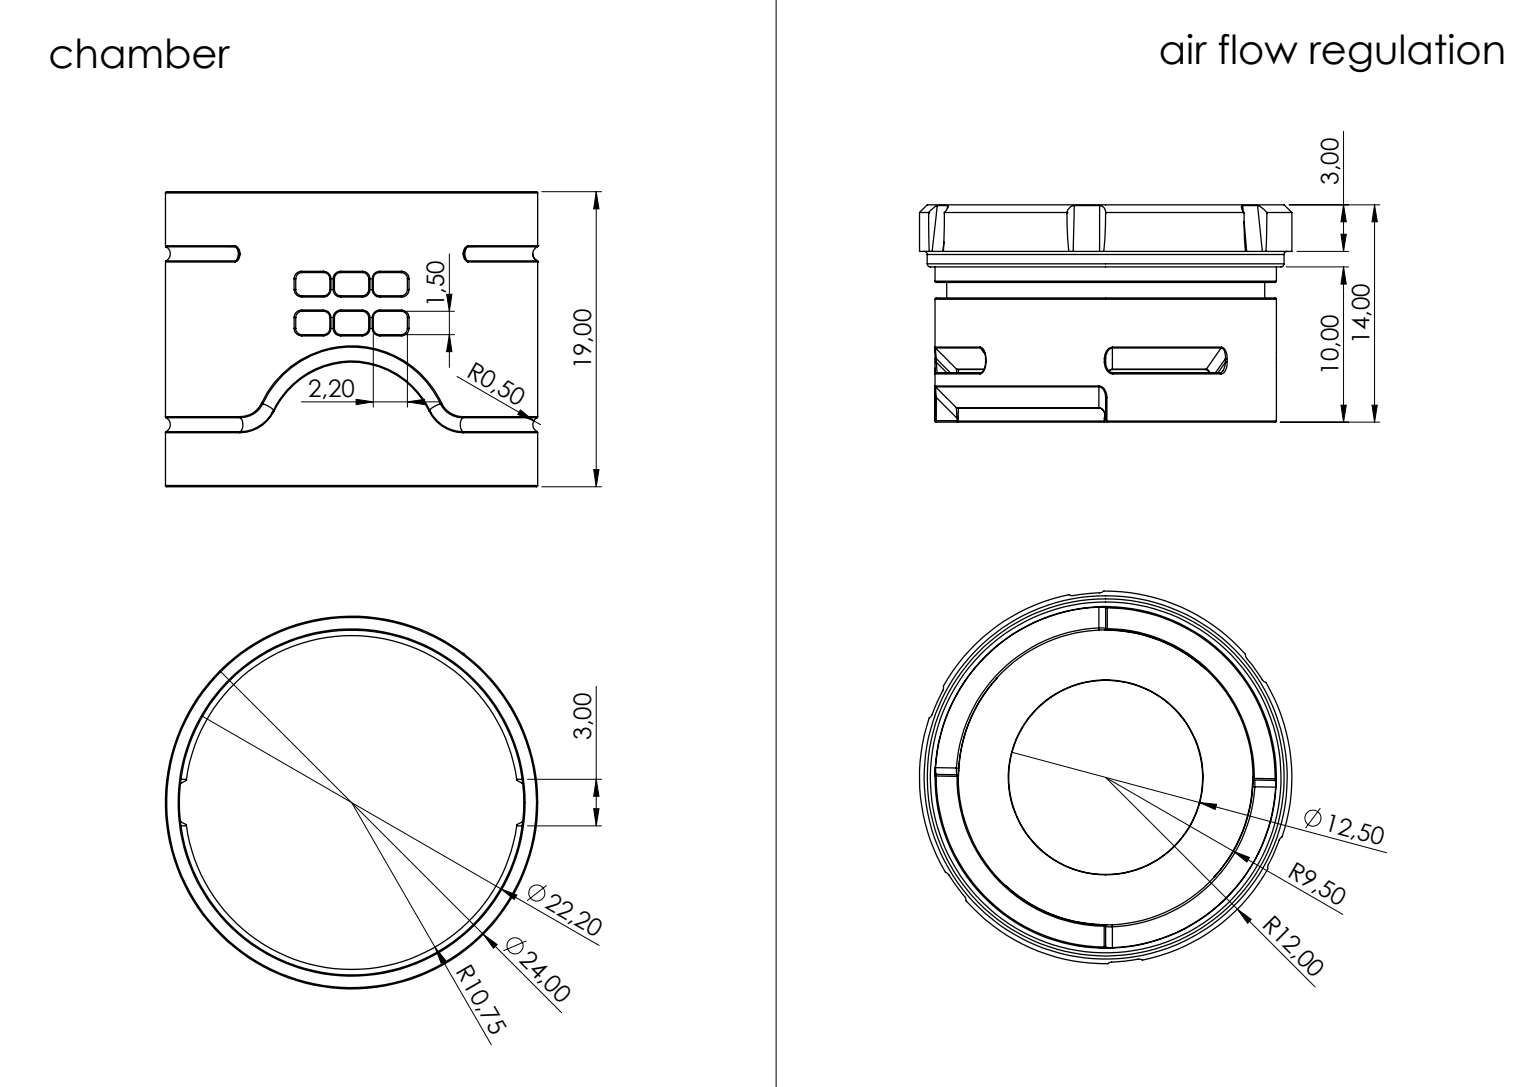
ISO-10303-21;
HEADER;
FILE_DESCRIPTION (('STEP AP214'),
    '1' );
FILE_NAME ('chamber.step',
    '2026-10-05T20:10:51',
    ( '' ),
    ( '' ),
    'SwSTEP 2.0',
    'SolidWorks 2020',
    '' );
FILE_SCHEMA (( 'AUTOMOTIVE_DESIGN' ));
ENDSEC;

DATA;
#17=CARTESIAN_POINT ( 'NONE',  ( 11.89942855770814312, 9.799999999999998934, 0.6999999999999992895 ) ) ;
#42=PRESENTATION_STYLE_ASSIGNMENT (( #185202 ) ) ;
#61=FACE_OUTER_BOUND ( 'NONE', #36024, .T. ) ;
#92=CARTESIAN_POINT ( 'NONE',  ( 6.928203230275524760, 15.51845925587262798, -9.797958971132702644 ) ) ;
#96=CARTESIAN_POINT ( 'NONE',  ( 11.88237951145550220, 12.34319347378715115, 0.9087114598430685586 ) ) ;
#105=CARTESIAN_POINT ( 'NONE',  ( -9.333041836226904309, 15.44694763438996077, -7.472413793095822321 ) ) ;
#118=ORIENTED_EDGE ( 'NONE', *, *, #154536, .F. ) ;
#120=CARTESIAN_POINT ( 'NONE',  ( 10.50000000000000355, 11.00832445802304882, -3.600000000000000533 ) ) ;
#124=VERTEX_POINT ( 'NONE', #206751 ) ;
#158=CARTESIAN_POINT ( 'NONE',  ( -10.12724623727299900, 3.700526055228949840, -6.355430437403613020 ) ) ;
#163=CARTESIAN_POINT ( 'NONE',  ( 11.84668730067608244, 12.69999999999998153, 1.399999999999998357 ) ) ;
#164=CARTESIAN_POINT ( 'NONE',  ( -11.92051736251532112, 12.44819756207321149, -1.381800029228967386 ) ) ;
#189=DIRECTION ( 'NONE',  ( 0.000000000000000000, 1.000000000000000000, 0.000000000000000000 ) ) ;
#190=FACE_OUTER_BOUND ( 'NONE', #152846, .T. ) ;
#192=ORIENTED_EDGE ( 'NONE', *, *, #191821, .F. ) ;
#199=ORIENTED_EDGE ( 'NONE', *, *, #95230, .T. ) ;
#216=CARTESIAN_POINT ( 'NONE',  ( 11.84668730067608244, 12.69999999999999929, -1.320000000000001616 ) ) ;
#223=EDGE_LOOP ( 'NONE', ( #165565, #34083, #144999, #128787 ) ) ;
#227=ORIENTED_EDGE ( 'NONE', *, *, #162616, .F. ) ;
#234=ORIENTED_EDGE ( 'NONE', *, *, #52222, .T. ) ;
#242=( NAMED_UNIT ( * ) PLANE_ANGLE_UNIT ( ) SI_UNIT ( $, .RADIAN. ) );
#252=CARTESIAN_POINT ( 'NONE',  ( 9.376191831160928913, 12.67849274587929820, -8.895508691099047738 ) ) ;
#267=LINE ( 'NONE', #66337, #6225 ) ;
#276=AXIS2_PLACEMENT_3D ( 'NONE', #147982, #164223, #79761 ) ;
#348=CARTESIAN_POINT ( 'NONE',  ( 8.061225138011870683, 15.94050400400142564, -9.794890688158101710 ) ) ;
#407=CARTESIAN_POINT ( 'NONE',  ( 9.501800845313253419, 13.11895608245291101, -7.330069317485494729 ) ) ;
#414=CIRCLE ( 'NONE', #87036, 11.09999999999999964 ) ;
#421=CARTESIAN_POINT ( 'NONE',  ( 11.91826849282518275, 12.69999999999999929, -1.400000000000001465 ) ) ;
#425=EDGE_CURVE ( 'NONE', #105059, #66250, #59241, .T. ) ;
#460=CARTESIAN_POINT ( 'NONE',  ( -11.37874721094434527, 6.569860378138817403, -3.816774967323496082 ) ) ;
#468=DIRECTION ( 'NONE',  ( -0.1510067114093955887, -0.000000000000000000, -0.9885327375000383388 ) ) ;
#486=DIRECTION ( 'NONE',  ( 1.000000000000000000, -0.000000000000000000, -0.000000000000000000 ) ) ;
#487=SURFACE_STYLE_USAGE ( .BOTH. , #166223 ) ;
#499=ORIENTED_EDGE ( 'NONE', *, *, #8528, .T. ) ;
#510=EDGE_CURVE ( 'NONE', #23152, #210434, #174637, .T. ) ;
#516=CARTESIAN_POINT ( 'NONE',  ( -10.62873463776380234, 12.29999999999998295, 3.199999999999997957 ) ) ;
#542=ORIENTED_EDGE ( 'NONE', *, *, #88694, .T. ) ;
#554=VECTOR ( 'NONE', #28356, 1000.000000000000000 ) ;
#599=CYLINDRICAL_SURFACE ( 'NONE', #53747, 0.3999999999999997446 ) ;
#634=CARTESIAN_POINT ( 'NONE',  ( -10.78402850230606447, 8.013881820625746499, 4.046242669647421408 ) ) ;
#648=EDGE_CURVE ( 'NONE', #121570, #167726, #212215, .T. ) ;
#662=UNCERTAINTY_MEASURE_WITH_UNIT (LENGTH_MEASURE( 1.000000000000000082E-05 ), #182215, 'distance_accuracy_value', 'NONE');
#671=DIRECTION ( 'NONE',  ( 1.000000000000000000, -0.000000000000000000, -0.000000000000000000 ) ) ;
#700=ADVANCED_FACE ( 'NONE', ( #185046 ), #198533, .T. ) ;
#702=VERTEX_POINT ( 'NONE', #118001 ) ;
#718=VECTOR ( 'NONE', #62707, 1000.000000000000000 ) ;
#733=CARTESIAN_POINT ( 'NONE',  ( -9.399770542442999144, 4.999985930147239799, -6.933469103752857521 ) ) ;
#743=CARTESIAN_POINT ( 'NONE',  ( -11.96215121607992593, 13.82833553780824154, -0.9565349792967606790 ) ) ;
#749=CARTESIAN_POINT ( 'NONE',  ( 11.53069314862830552, 7.261250335387300581, -3.355468136185856487 ) ) ;
#760=CARTESIAN_POINT ( 'NONE',  ( 10.67997715883384657, 8.352520031436601045, -3.105267373736821046 ) ) ;
#766=CIRCLE ( 'NONE', #108191, 0.07999999999999998779 ) ;
#773=EDGE_LOOP ( 'NONE', ( #1049, #99023, #98681, #151558, #138881, #82301, #133035, #37995, #73322, #97682, #96732, #136112, #8265, #74514, #72858, #38949, #164337, #200453 ) ) ;
#777=CARTESIAN_POINT ( 'NONE',  ( 0.08053691275167890185, 14.48153890507870223, 11.99972973886013961 ) ) ;
#831=EDGE_CURVE ( 'NONE', #191521, #28791, #95318, .T. ) ;
#836=( GEOMETRIC_REPRESENTATION_CONTEXT ( 3 ) GLOBAL_UNCERTAINTY_ASSIGNED_CONTEXT ( ( #213503 ) ) GLOBAL_UNIT_ASSIGNED_CONTEXT ( ( #89871, #123512, #158065 ) ) REPRESENTATION_CONTEXT ( 'NONE', 'WORKASPACE' ) );
#840=ORIENTED_EDGE ( 'NONE', *, *, #141283, .F. ) ;
#885=CARTESIAN_POINT ( 'NONE',  ( 11.84668730067608600, 13.40000000000000036, -1.400000000000001910 ) ) ;
#890=FACE_OUTER_BOUND ( 'NONE', #59511, .T. ) ;
#922=FACE_OUTER_BOUND ( 'NONE', #13196, .T. ) ;
#933=DIRECTION ( 'NONE',  ( 0.000000000000000000, 1.000000000000000000, 0.000000000000000000 ) ) ;
#936=VECTOR ( 'NONE', #86539, 1000.000000000000000 ) ;
#945=CARTESIAN_POINT ( 'NONE',  ( -1.499999999999964029, 8.500000000000000000, 9.886859966642596476 ) ) ;
#971=CARTESIAN_POINT ( 'NONE',  ( 11.33772463945037146, 12.69999999999998153, 3.599999999999999201 ) ) ;
#990=B_SPLINE_CURVE_WITH_KNOTS ( 'NONE', 3,
 ( #112463, #131886, #64702, #162226, #79885, #212006 ),
 .UNSPECIFIED., .F., .F.,
 ( 4, 2, 4 ),
 ( 0.001889712630306643673, 0.002203932548491402497, 0.002518152466676161320 ),
 .UNSPECIFIED. ) ;
#1001=AXIS2_PLACEMENT_3D ( 'NONE', #80650, #164042, #112153 ) ;
#1016=AXIS2_PLACEMENT_3D ( 'NONE', #89451, #186921, #6019 ) ;
#1034=CARTESIAN_POINT ( 'NONE',  ( -10.32660017610915837, 5.019824769181640889, 7.354833152352289183 ) ) ;
#1037=ADVANCED_FACE ( 'NONE', ( #178914 ), #183155, .F. ) ;
#1046=CARTESIAN_POINT ( 'NONE',  ( -11.45842088241054491, 11.09306470877032069, 3.566211699757684261 ) ) ;
#1049=ORIENTED_EDGE ( 'NONE', *, *, #67497, .T. ) ;
#1053=CARTESIAN_POINT ( 'NONE',  ( -15.75000000000000000, 10.19999999999998153, 3.599999999999999201 ) ) ;
#1054=FACE_OUTER_BOUND ( 'NONE', #104348, .T. ) ;
#1062=CARTESIAN_POINT ( 'NONE',  ( -11.37613258624509349, 7.826217927974032484, 3.683897043248439029 ) ) ;
#1063=CARTESIAN_POINT ( 'NONE',  ( 11.78331023100045627, 12.29999999999998295, 1.799999999999999600 ) ) ;
#1081=CARTESIAN_POINT ( 'NONE',  ( 11.89942855770813956, 12.22000000000000064, 0.6999999999999992895 ) ) ;
#1092=VECTOR ( 'NONE', #206274, 1000.000000000000000 ) ;
#1097=CIRCLE ( 'NONE', #56491, 11.92000000000000171 ) ;
#1116=CARTESIAN_POINT ( 'NONE',  ( 0.000000000000000000, 12.22000000000000064, 0.000000000000000000 ) ) ;
#1117=VERTEX_POINT ( 'NONE', #82446 ) ;
#1124=CARTESIAN_POINT ( 'NONE',  ( 11.55950211276791251, 11.37999999999998302, 3.221476510067114329 ) ) ;
#1132=CARTESIAN_POINT ( 'NONE',  ( 11.86239285000045918, 11.37999999999999901, -1.812080536912753059 ) ) ;
#1145=CARTESIAN_POINT ( 'NONE',  ( 6.902720183911290164, 14.55305236562705318, -9.761920501353818835 ) ) ;
#1159=ORIENTED_EDGE ( 'NONE', *, *, #134668, .F. ) ;
#1233=CARTESIAN_POINT ( 'NONE',  ( -10.89183333199790482, 4.909323612238607915, -5.036858318171161919 ) ) ;
#1240=LINE ( 'NONE', #117214, #18483 ) ;
#1265=CARTESIAN_POINT ( 'NONE',  ( -1.785627835867960034, 15.44799008577503585, -11.82984269095817353 ) ) ;
#1266=CARTESIAN_POINT ( 'NONE',  ( 11.78331023100045627, 11.29999999999999893, -1.800000000000001155 ) ) ;
#1268=CIRCLE ( 'NONE', #122445, 12.00000000000000178 ) ;
#1295=CARTESIAN_POINT ( 'NONE',  ( 11.86145016429273191, 10.90000000000000036, 1.099999999999996758 ) ) ;
#1299=VERTEX_POINT ( 'NONE', #59288 ) ;
#1315=CARTESIAN_POINT ( 'NONE',  ( -11.43653507270588499, 5.655220009861049668, 5.468867579827167980 ) ) ;
#1378=CARTESIAN_POINT ( 'NONE',  ( -10.43233925736708301, 5.066585305077033752, -5.254699789447807134 ) ) ;
#1379=CARTESIAN_POINT ( 'NONE',  ( -9.348561386651960348, 4.000000000000000888, 7.001914024036570261 ) ) ;
#1405=FACE_OUTER_BOUND ( 'NONE', #99903, .T. ) ;
#1425=CARTESIAN_POINT ( 'NONE',  ( 7.320801413324473650, 14.00000000000000000, -10.35317664616355771 ) ) ;
#1442=CARTESIAN_POINT ( 'NONE',  ( 10.62873463776380056, 12.30000000000000071, -3.200000000000001510 ) ) ;
#1480=CARTESIAN_POINT ( 'NONE',  ( 1.448815997565377156, 7.903552007303750848, -10.65195286442484601 ) ) ;
#1482=EDGE_CURVE ( 'NONE', #30243, #96092, #98102, .T. ) ;
#1521=CARTESIAN_POINT ( 'NONE',  ( -9.333041836230696831, 14.55305236563169302, -7.472413793098840351 ) ) ;
#1554=ORIENTED_EDGE ( 'NONE', *, *, #33991, .T. ) ;
#1620=CIRCLE ( 'NONE', #57014, 0.07999999999999998779 ) ;
#1668=AXIS2_PLACEMENT_3D ( 'NONE', #81303, #62908, #211285 ) ;
#1710=CARTESIAN_POINT ( 'NONE',  ( 0.3263184169966619752, 15.00000000000058265, -11.67999999558625213 ) ) ;
#1712=CARTESIAN_POINT ( 'NONE',  ( -10.44369633504468631, 5.112959841837462882, -5.232137017608344820 ) ) ;
#1743=DIRECTION ( 'NONE',  ( 0.000000000000000000, 0.000000000000000000, 1.000000000000000000 ) ) ;
#1752=DIRECTION ( 'NONE',  ( 0.000000000000000000, 0.000000000000000000, 1.000000000000000000 ) ) ;
#1769=CIRCLE ( 'NONE', #174839, 0.5000000000000016653 ) ;
#1774=( NAMED_UNIT ( * ) PLANE_ANGLE_UNIT ( ) SI_UNIT ( $, .RADIAN. ) );
#1783=CARTESIAN_POINT ( 'NONE',  ( 11.95359438121989726, 9.995781002913002311, -1.059536798430469107 ) ) ;
#1810=CARTESIAN_POINT ( 'NONE',  ( -11.75342398721120141, 4.618418902329548992, -5.022351803590792585 ) ) ;
#1821=( NAMED_UNIT ( * ) PLANE_ANGLE_UNIT ( ) SI_UNIT ( $, .RADIAN. ) );
#1825=ORIENTED_EDGE ( 'NONE', *, *, #25480, .F. ) ;
#1828=CARTESIAN_POINT ( 'NONE',  ( 11.09870862492791233, 7.996335997987229049, -4.583701278145491109 ) ) ;
#1840=CARTESIAN_POINT ( 'NONE',  ( 10.48872307347595090, 11.88768493876267485, 6.438521854865753014 ) ) ;
#1849=CARTESIAN_POINT ( 'NONE',  ( -11.88235317400313917, 12.34335760226970358, 0.9089793033029930358 ) ) ;
#1856=STYLED_ITEM ( 'NONE', ( #32642 ), #1037 ) ;
#1895=CARTESIAN_POINT ( 'NONE',  ( 0.000000000000000000, 3.553052365627050513, 0.000000000000000000 ) ) ;
#1976=CIRCLE ( 'NONE', #22858, 0.07999999999999946043 ) ;
#1999=DIRECTION ( 'NONE',  ( 0.000000000000000000, 1.000000000000000000, 0.000000000000000000 ) ) ;
#2010=CARTESIAN_POINT ( 'NONE',  ( 0.000000000000000000, 18.91999999999999815, 0.000000000000000000 ) ) ;
#2037=CARTESIAN_POINT ( 'NONE',  ( 8.748033642589533088, 13.52645069410513479, 8.214566069811549909 ) ) ;
#2094=FILL_AREA_STYLE_COLOUR ( '', #209766 ) ;
#2096=CARTESIAN_POINT ( 'NONE',  ( -9.928151704202875294, 5.423124072284297270, 6.082134274749043001 ) ) ;
#2098=LINE ( 'NONE', #81258, #144593 ) ;
#2101=AXIS2_PLACEMENT_3D ( 'NONE', #159302, #14090, #63931 ) ;
#2120=CARTESIAN_POINT ( 'NONE',  ( -10.63115277548007498, 5.888090174969209833, -5.475543521278559922 ) ) ;
#2123=FACE_OUTER_BOUND ( 'NONE', #176365, .T. ) ;
#2148=EDGE_CURVE ( 'NONE', #31723, #61426, #1268, .T. ) ;
#2180=DIRECTION ( 'NONE',  ( 0.000000000000000000, -1.000000000000000000, -9.023263958591317418E-17 ) ) ;
#2199=ORIENTED_EDGE ( 'NONE', *, *, #9864, .T. ) ;
#2205=DIRECTION ( 'NONE',  ( 1.000000000000000000, -0.000000000000000000, -0.000000000000000000 ) ) ;
#2216=VECTOR ( 'NONE', #157528, 1000.000000000000000 ) ;
#2241=CARTESIAN_POINT ( 'NONE',  ( -10.51596412982177853, 9.986590817315772028, -3.553961965504329967 ) ) ;
#2257=CIRCLE ( 'NONE', #26555, 12.00000000000000178 ) ;
#2259=ORIENTED_EDGE ( 'NONE', *, *, #27400, .F. ) ;
#2292=CARTESIAN_POINT ( 'NONE',  ( -10.84253909858433218, 4.919570308430901484, -5.035411995924089723 ) ) ;
#2295=DIRECTION ( 'NONE',  ( -0.000000000000000000, -1.000000000000000000, -0.000000000000000000 ) ) ;
#2314=EDGE_CURVE ( 'NONE', #158402, #95365, #73964, .T. ) ;
#2318=VERTEX_POINT ( 'NONE', #66709 ) ;
#2327=LINE ( 'NONE', #34843, #100006 ) ;
#2336=ORIENTED_EDGE ( 'NONE', *, *, #208712, .T. ) ;
#2343=( BOUNDED_SURFACE ( )  B_SPLINE_SURFACE ( 3, 2, ( 
 ( #205237, #55808, #154383 ),
 ( #105661, #204153, #141381 ),
 ( #56878, #5960, #187929 ),
 ( #41724, #157600, #207391 ),
 ( #73106, #125168, #189007 ),
 ( #158656, #171688, #191127 ) ),
 .UNSPECIFIED., .F., .F., .T. ) 
 B_SPLINE_SURFACE_WITH_KNOTS ( ( 4, 2, 4 ),
 ( 3, 3 ),
 ( 0.000000000000000000, 0.0003754689591423960443, 0.0007509379182847920886 ),
 ( 0.000000000000000000, 1.000000000000000000 ),
 .UNSPECIFIED. ) 
 GEOMETRIC_REPRESENTATION_ITEM ( )  RATIONAL_B_SPLINE_SURFACE ( (
 ( 1.000000000000000000, 0.7071067811865551223, 1.000000000000000000),
 ( 1.000000000000000000, 0.7018599272024059754, 1.000000000000000000),
 ( 1.000000000000000000, 0.6927733177260235742, 1.000000000000000000),
 ( 1.000000000000000000, 0.6772007068873748814, 1.000000000000000000),
 ( 1.000000000000000000, 0.6709974581637072610, 1.000000000000000000),
 ( 1.000000000000000000, 0.6711954675835395401, 1.000000000000000000) ) ) 
 REPRESENTATION_ITEM ( '' )  SURFACE ( )  );
#2377=CARTESIAN_POINT ( 'NONE',  ( -12.65133343644925823, 8.691152131673410608, 1.253321570098529181 ) ) ;
#2390=CARTESIAN_POINT ( 'NONE',  ( 12.43511541931632891, 7.569548269842172772, -1.878403980710225518 ) ) ;
#2396=CARTESIAN_POINT ( 'NONE',  ( -11.86145016429273191, 12.69999999999999929, 1.099999999999996758 ) ) ;
#2399=FACE_OUTER_BOUND ( 'NONE', #26284, .T. ) ;
#2404=ADVANCED_FACE ( 'NONE', ( #7621 ), #121100, .F. ) ;
#2430=DIRECTION ( 'NONE',  ( -0.6250000000000002220, 1.408756634010579298E-16, -0.7806247497997996776 ) ) ;
#2431=EDGE_CURVE ( 'NONE', #156842, #15788, #193107, .T. ) ;
#2440=CARTESIAN_POINT ( 'NONE',  ( -11.25771003949915539, 3.534410846742664702, -5.930344140359695260 ) ) ;
#2441=CARTESIAN_POINT ( 'NONE',  ( -9.811677024507259759, 4.107325997343203028, 6.339424533126782002 ) ) ;
#2445=CARTESIAN_POINT ( 'NONE',  ( -11.99141368677939035, 8.009080577729674744, -0.5230012777734741602 ) ) ;
#2489=CARTESIAN_POINT ( 'NONE',  ( 6.938157974219377522, 13.99567801284426416, -9.395936565436949550 ) ) ;
#2508=CARTESIAN_POINT ( 'NONE',  ( -9.569358774130488854, 4.446955548196734220, -7.167287524826102540 ) ) ;
#2546=CARTESIAN_POINT ( 'NONE',  ( 9.605087238846238051, 12.70381962237584972, -7.196083043797907308 ) ) ;
#2550=CARTESIAN_POINT ( 'NONE',  ( 11.88168329227126563, 13.88000000000000256, -1.685799833707129380 ) ) ;
#2561=B_SPLINE_CURVE_WITH_KNOTS ( 'NONE', 3,
 ( #59467, #111488, #126690, #58410, #193728, #8580, #125626, #176430, #94134, #192652 ),
 .UNSPECIFIED., .F., .F.,
 ( 4, 2, 2, 2, 4 ),
 ( 0.000000000000000000, 0.0003474354322518759990, 0.0006948708645037519980, 0.001042306296755630491, 0.001389741729007509200 ),
 .UNSPECIFIED. ) ;
#2571=CIRCLE ( 'NONE', #5975, 12.00000000000000178 ) ;
#2590=AXIS2_PLACEMENT_3D ( 'NONE', #106985, #204391, #120046 ) ;
#2602=CARTESIAN_POINT ( 'NONE',  ( -11.89942855770814134, 11.29999999999999893, 0.6999999999999992895 ) ) ;
#2611=CARTESIAN_POINT ( 'NONE',  ( -11.75854610579106563, 8.612401473491297921, 2.412033672967001774 ) ) ;
#2626=DIRECTION ( 'NONE',  ( 0.000000000000000000, 1.000000000000000000, 0.000000000000000000 ) ) ;
#2649=ORIENTED_EDGE ( 'NONE', *, *, #149426, .T. ) ;
#2690=EDGE_CURVE ( 'NONE', #41918, #170318, #144540, .T. ) ;
#2723=CARTESIAN_POINT ( 'NONE',  ( -11.88172094500854037, 13.87999994398404269, 1.685553348215819147 ) ) ;
#2748=CARTESIAN_POINT ( 'NONE',  ( -10.50000000000000533, 11.00709944181895494, 3.599999999999998312 ) ) ;
#2773=CARTESIAN_POINT ( 'NONE',  ( -3.501245407923440300, 14.00000000000179057, -11.28115623562633019 ) ) ;
#2776=CARTESIAN_POINT ( 'NONE',  ( -10.07169253693141897, 5.946554136026001913, 5.792750394403223702 ) ) ;
#2786=ORIENTED_EDGE ( 'NONE', *, *, #64280, .T. ) ;
#2791=ORIENTED_EDGE ( 'NONE', *, *, #98727, .F. ) ;
#2823=EDGE_CURVE ( 'NONE', #173974, #75921, #6244, .T. ) ;
#2828=AXIS2_PLACEMENT_3D ( 'NONE', #8850, #126966, #62933 ) ;
#2846=FACE_OUTER_BOUND ( 'NONE', #122610, .T. ) ;
#2872=CARTESIAN_POINT ( 'NONE',  ( -11.94654170777226376, 11.15174326158935969, -1.134972293687621647 ) ) ;
#2875=CARTESIAN_POINT ( 'NONE',  ( -11.29167836119662738, 5.103960725615834804, -5.764738477843053488 ) ) ;
#2885=CARTESIAN_POINT ( 'NONE',  ( -15.75000000000000000, 9.799999999999982947, 3.199999999999997957 ) ) ;
#2891=CARTESIAN_POINT ( 'NONE',  ( 10.91404093077409243, 8.232440706712328193, 5.004496970253279109 ) ) ;
#2902=STYLED_ITEM ( 'NONE', ( #95623 ), #40584 ) ;
#2903=DIRECTION ( 'NONE',  ( -0.000000000000000000, 1.000000000000000000, -0.000000000000000000 ) ) ;
#2904=CARTESIAN_POINT ( 'NONE',  ( 9.476778946274437843, 12.06403068260519795, 6.318147453416640857 ) ) ;
#2914=LINE ( 'NONE', #200062, #99689 ) ;
#2915=CARTESIAN_POINT ( 'NONE',  ( 8.731305104352237834, 13.51198939287863610, -8.232175732474900087 ) ) ;
#2916=CARTESIAN_POINT ( 'NONE',  ( -8.140681553543240412, 15.44816072426944409, -8.801270232398126225 ) ) ;
#2931=( NAMED_UNIT ( * ) SI_UNIT ( $, .STERADIAN. ) SOLID_ANGLE_UNIT ( ) );
#2979=DIRECTION ( 'NONE',  ( -0.000000000000000000, -1.000000000000000000, -0.000000000000000000 ) ) ;
#2982=EDGE_CURVE ( 'NONE', #8666, #41918, #10157, .T. ) ;
#3034=TOROIDAL_SURFACE ( 'NONE', #20367, 11.92000000000000171, 0.08000000000000000167 ) ;
#3047=DIRECTION ( 'NONE',  ( 0.000000000000000000, 0.000000000000000000, 1.000000000000000000 ) ) ;
#3078=SURFACE_STYLE_USAGE ( .BOTH. , #103821 ) ;
#3092=EDGE_CURVE ( 'NONE', #147946, #136086, #58918, .T. ) ;
#3164=CARTESIAN_POINT ( 'NONE',  ( -9.541824394042135893, 5.027248526908232762, 6.730710380108894775 ) ) ;
#3176=TOROIDAL_SURFACE ( 'NONE', #93235, 12.18000000000000149, 0.5000000000000008882 ) ;
#3208=FILL_AREA_STYLE ('',( #71413 ) ) ;
#3217=CARTESIAN_POINT ( 'NONE',  ( 9.305047017613615523, 4.518459255872631530, 7.450000000000001954 ) ) ;
#3226=AXIS2_PLACEMENT_3D ( 'NONE', #149518, #38967, #133299 ) ;
#3244=( NAMED_UNIT ( * ) SI_UNIT ( $, .STERADIAN. ) SOLID_ANGLE_UNIT ( ) );
#3251=CARTESIAN_POINT ( 'NONE',  ( -11.48243876534946040, 12.30000000000000071, -3.200000000000001510 ) ) ;
#3274=CARTESIAN_POINT ( 'NONE',  ( -11.55950211276791428, 9.719999999999982876, 3.221476510067114329 ) ) ;
#3277=DIRECTION ( 'NONE',  ( 0.000000000000000000, 1.000000000000000000, 0.000000000000000000 ) ) ;
#3278=CARTESIAN_POINT ( 'NONE',  ( -11.86145016429273014, 13.40000000000000036, -1.100000000000002087 ) ) ;
#3283=EDGE_CURVE ( 'NONE', #56620, #154122, #103069, .T. ) ;
#3292=ORIENTED_EDGE ( 'NONE', *, *, #59260, .F. ) ;
#3311=CYLINDRICAL_SURFACE ( 'NONE', #106397, 0.08000000000000020983 ) ;
#3312=CARTESIAN_POINT ( 'NONE',  ( -9.399990540229763880, 5.000000000000003553, 6.933248713717822476 ) ) ;
#3315=UNCERTAINTY_MEASURE_WITH_UNIT (LENGTH_MEASURE( 1.000000000000000082E-05 ), #57416, 'distance_accuracy_value', 'NONE');
#3327=DIRECTION ( 'NONE',  ( 0.000000000000000000, -1.000000000000000000, 0.000000000000000000 ) ) ;
#3345=CARTESIAN_POINT ( 'NONE',  ( -9.498276863157586902, 15.41940897614170147, -7.333831086994896609 ) ) ;
#3349=SURFACE_SIDE_STYLE ('',( #151777 ) ) ;
#3363=ORIENTED_EDGE ( 'NONE', *, *, #64050, .T. ) ;
#3376=CARTESIAN_POINT ( 'NONE',  ( 11.41381675112453387, 13.40000000000000036, -3.704697986577182522 ) ) ;
#3399=CARTESIAN_POINT ( 'NONE',  ( 11.86145016429272836, 10.90000000000000036, -1.100000000000000533 ) ) ;
#3408=CARTESIAN_POINT ( 'NONE',  ( -11.84668730067608600, 13.39999999999998259, 1.319999999999998286 ) ) ;
#3410=EDGE_CURVE ( 'NONE', #81409, #108056, #78356, .T. ) ;
#3443=DIRECTION ( 'NONE',  ( 0.000000000000000000, -1.000000000000000000, 0.000000000000000000 ) ) ;
#3450=CARTESIAN_POINT ( 'NONE',  ( -10.48266952940149466, 5.268049057482275366, -5.154014898524191146 ) ) ;
#3451=CARTESIAN_POINT ( 'NONE',  ( -15.75000000000000000, 10.90000000000000036, -1.400000000000001910 ) ) ;
#3473=ORIENTED_EDGE ( 'NONE', *, *, #13918, .F. ) ;
#3508=CARTESIAN_POINT ( 'NONE',  ( -11.78331023100045627, 9.719999999999998863, -1.800000000000001155 ) ) ;
#3527=DIRECTION ( 'NONE',  ( 1.000000000000000000, -0.000000000000000000, -0.000000000000000000 ) ) ;
#3534=AXIS2_PLACEMENT_3D ( 'NONE', #143410, #145552, #92518 ) ;
#3545=B_SPLINE_CURVE_WITH_KNOTS ( 'NONE', 3,
 ( #74509, #140613, #124411, #190369, #86484, #21450, #4136, #70204 ),
 .UNSPECIFIED., .F., .F.,
 ( 4, 2, 2, 4 ),
 ( 0.000000000000000000, 0.0007626201316526405984, 0.001525240263305281197, 0.003050480526610564996 ),
 .UNSPECIFIED. ) ;
#3558=CARTESIAN_POINT ( 'NONE',  ( 7.320801413324473650, 15.00000000000000000, -10.35317664616355771 ) ) ;
#3574=CARTESIAN_POINT ( 'NONE',  ( 11.92051736251532823, 13.65180243792678638, -1.381800029228912763 ) ) ;
#3585=CARTESIAN_POINT ( 'NONE',  ( -11.14501278000869355, 7.223412960316487386, -3.546411330735405265 ) ) ;
#3606=CARTESIAN_POINT ( 'NONE',  ( -9.380315450342122219, 15.46908200564950775, 7.483989756882012401 ) ) ;
#3626=CARTESIAN_POINT ( 'NONE',  ( 11.81905481421901705, 9.842643443827320482, 1.592167362352177262 ) ) ;
#3659=CARTESIAN_POINT ( 'NONE',  ( -11.89942855770814134, 12.30000000000000071, -0.7000000000000009548 ) ) ;
#3660=CARTESIAN_POINT ( 'NONE',  ( -11.86687934130374522, 11.10951949616558565, 1.056332641424306606 ) ) ;
#3670=CARTESIAN_POINT ( 'NONE',  ( -11.56555315273234719, 8.166926488375429116, 3.210420282871015996 ) ) ;
#3699=VERTEX_POINT ( 'NONE', #161302 ) ;
#3700=CARTESIAN_POINT ( 'NONE',  ( 11.92619526913699879, 13.39999999999998259, 1.328859060402684644 ) ) ;
#3703=ORIENTED_EDGE ( 'NONE', *, *, #93584, .T. ) ;
#3725=CARTESIAN_POINT ( 'NONE',  ( -11.99998504853427583, 9.073077996143771529, -0.6178450063080842547 ) ) ;
#3774=EDGE_CURVE ( 'NONE', #12777, #158047, #212151, .T. ) ;
#3832=CARTESIAN_POINT ( 'NONE',  ( 0.7124089920921370389, 15.00000000000000711, -12.66466791154696558 ) ) ;
#3834=CARTESIAN_POINT ( 'NONE',  ( -11.52114515671133610, 8.081606464056415362, 2.192706985476595261 ) ) ;
#3843=DIRECTION ( 'NONE',  ( -0.000000000000000000, 0.000000000000000000, -1.000000000000000000 ) ) ;
#3877=SURFACE_STYLE_USAGE ( .BOTH. , #85161 ) ;
#3879=AXIS2_PLACEMENT_3D ( 'NONE', #113728, #933, #69137 ) ;
#3912=DIRECTION ( 'NONE',  ( -0.1510067114093955887, -0.000000000000000000, -0.9885327375000383388 ) ) ;
#3914=EDGE_CURVE ( 'NONE', #204988, #120419, #141146, .T. ) ;
#3934=ORIENTED_EDGE ( 'NONE', *, *, #112984, .F. ) ;
#3938=EDGE_CURVE ( 'NONE', #101924, #2318, #9654, .T. ) ;
#3942=CARTESIAN_POINT ( 'NONE',  ( -10.83049189199067719, 4.361170120774730208, -4.636001201543571426 ) ) ;
#3953=CARTESIAN_POINT ( 'NONE',  ( 0.000000000000000000, 13.79999999999999893, 0.000000000000000000 ) ) ;
#3959=CARTESIAN_POINT ( 'NONE',  ( 11.65634836436412947, 7.079629224059313053, -2.645114728738123144 ) ) ;
#3971=CARTESIAN_POINT ( 'NONE',  ( 9.390682975800181964, 11.17576483377143681, 6.985571074475002362 ) ) ;
#3972=AXIS2_PLACEMENT_3D ( 'NONE', #186734, #173725, #206181 ) ;
#3998=FACE_OUTER_BOUND ( 'NONE', #11820, .T. ) ;
#4014=PRESENTATION_STYLE_ASSIGNMENT (( #149227 ) ) ;
#4035=MECHANICAL_DESIGN_GEOMETRIC_PRESENTATION_REPRESENTATION('',(#132131),#83686);
#4041=EDGE_CURVE ( 'NONE', #37994, #61984, #37334, .T. ) ;
#4062=ADVANCED_FACE ( 'NONE', ( #182490 ), #100491, .T. ) ;
#4080=CARTESIAN_POINT ( 'NONE',  ( -11.86685672517501899, 9.990810821401886699, 1.056525322636010289 ) ) ;
#4085=ORIENTED_EDGE ( 'NONE', *, *, #79933, .T. ) ;
#4132=CARTESIAN_POINT ( 'NONE',  ( -15.75000000000000000, 9.799999999999998934, -0.7000000000000009548 ) ) ;
#4134=STYLED_ITEM ( 'NONE', ( #8897 ), #173118 ) ;
#4136=CARTESIAN_POINT ( 'NONE',  ( -9.913101724262725511, 3.481548657788669399, -6.781968449710928049 ) ) ;
#4169=DIRECTION ( 'NONE',  ( 1.224643483124941457E-16, 0.002327115863041261980, 0.9999972922622142324 ) ) ;
#4178=CARTESIAN_POINT ( 'NONE',  ( 11.41381675112453387, 12.69999999999998153, 3.704697986577180746 ) ) ;
#4186=( GEOMETRIC_REPRESENTATION_CONTEXT ( 3 ) GLOBAL_UNCERTAINTY_ASSIGNED_CONTEXT ( ( #153294 ) ) GLOBAL_UNIT_ASSIGNED_CONTEXT ( ( #105235, #6623, #42376 ) ) REPRESENTATION_CONTEXT ( 'NONE', 'WORKASPACE' ) );
#4246=AXIS2_PLACEMENT_3D ( 'NONE', #61852, #191832, #43495 ) ;
#4278=CARTESIAN_POINT ( 'NONE',  ( 11.86145016429272836, 12.69999999999999929, 1.179999999999997051 ) ) ;
#4296=CARTESIAN_POINT ( 'NONE',  ( -11.94980361058169116, 10.89999999999999858, 1.099999999999994982 ) ) ;
#4304=CARTESIAN_POINT ( 'NONE',  ( -9.904322480959008246, 3.508507969777028279, 6.779889285468879478 ) ) ;
#4340=DIRECTION ( 'NONE',  ( 0.000000000000000000, -1.000000000000000000, 0.000000000000000000 ) ) ;
#4372=DIRECTION ( 'NONE',  ( 1.000000000000000000, -0.000000000000000000, -0.000000000000000000 ) ) ;
#4373=CARTESIAN_POINT ( 'NONE',  ( -10.36733242867369142, 5.031604590660524678, 7.295138277318285347 ) ) ;
#4380=ORIENTED_EDGE ( 'NONE', *, *, #59990, .T. ) ;
#4385=EDGE_LOOP ( 'NONE', ( #39707, #165219, #127190, #169715 ) ) ;
#4387=CARTESIAN_POINT ( 'NONE',  ( 10.51593585047793233, 11.11323312775290439, -3.554043120631340535 ) ) ;
#4390=ORIENTED_EDGE ( 'NONE', *, *, #129415, .F. ) ;
#4403=CIRCLE ( 'NONE', #77098, 0.07999999999999998779 ) ;
#4405=CIRCLE ( 'NONE', #87472, 0.08000000000000040412 ) ;
#4413=CARTESIAN_POINT ( 'NONE',  ( 11.94980361723123785, 13.50238056585427060, 1.099999926404769290 ) ) ;
#4421=ORIENTED_EDGE ( 'NONE', *, *, #70055, .F. ) ;
#4427=DIRECTION ( 'NONE',  ( 0.9885327375000381167, 0.000000000000000000, 0.1510067114093955609 ) ) ;
#4441=CARTESIAN_POINT ( 'NONE',  ( -15.75000000000000000, 10.19999999999998153, 3.599999999999999201 ) ) ;
#4454=CARTESIAN_POINT ( 'NONE',  ( -3.518398841103404173, 15.44797950387303054, -11.43484029727943607 ) ) ;
#4468=FACE_BOUND ( 'NONE', #29943, .T. ) ;
#4487=DIRECTION ( 'NONE',  ( -1.224646799147343346E-16, 0.000000000000000000, -1.000000000000000000 ) ) ;
#4490=ORIENTED_EDGE ( 'NONE', *, *, #99349, .T. ) ;
#4497=COLOUR_RGB ( '', 0.08235294, 0.09019608, 0.10196078) ;
#4506=CARTESIAN_POINT ( 'NONE',  ( -10.45142907045522129, 5.144535043903895932, -5.216774619840575333 ) ) ;
#4518=CARTESIAN_POINT ( 'NONE',  ( 9.741349722503858999, 13.15934765701661391, 8.090281636115273400 ) ) ;
#4563=VERTEX_POINT ( 'NONE', #5856 ) ;
#4571=CARTESIAN_POINT ( 'NONE',  ( -10.37901820579008039, 4.889546506944066451, 5.358714317323078014 ) ) ;
#4636=ORIENTED_EDGE ( 'NONE', *, *, #3283, .T. ) ;
#4637=ORIENTED_EDGE ( 'NONE', *, *, #35345, .F. ) ;
#4669=CARTESIAN_POINT ( 'NONE',  ( 7.046081134561259951, 15.44736638506130610, 9.660548086161224290 ) ) ;
#4670=CARTESIAN_POINT ( 'NONE',  ( -11.88168329227127096, 13.87999999999998479, 1.685799833707126050 ) ) ;
#4671=VERTEX_POINT ( 'NONE', #73005 ) ;
#4680=CARTESIAN_POINT ( 'NONE',  ( 11.86687934130374522, 11.10951949616558565, -1.056332641424308827 ) ) ;
#4734=CARTESIAN_POINT ( 'NONE',  ( -11.06825346762359885, 7.101010065767195734, 4.641007292122007577 ) ) ;
#4777=CARTESIAN_POINT ( 'NONE',  ( -0.07926568655891585991, 15.51719745866557432, 11.99972817042865181 ) ) ;
#4784=CARTESIAN_POINT ( 'NONE',  ( 0.000000000000000000, 9.719999999999982876, 0.000000000000000000 ) ) ;
#4785=CARTESIAN_POINT ( 'NONE',  ( 0.000000000000000000, 14.48154074412737202, 0.000000000000000000 ) ) ;
#4802=EDGE_CURVE ( 'NONE', #135251, #147625, #51264, .T. ) ;
#4811=CARTESIAN_POINT ( 'NONE',  ( 1.050790385995002740, 15.00000000000000355, 12.64745918785790302 ) ) ;
#4822=B_SPLINE_CURVE_WITH_KNOTS ( 'NONE', 3,
 ( #135801, #115345, #99038, #50281, #83828, #68630, #84903, #82769, #152050, #148843, #100092, #150990, #182388, #184520 ),
 .UNSPECIFIED., .F., .F.,
 ( 4, 2, 2, 2, 2, 2, 4 ),
 ( -5.999999995607368656E-08, 0.0007641236830326251584, 0.001146215524548915496, 0.001528307366065205725, 0.002292491049097787267, 0.002674582890614078581, 0.003056674732130369894 ),
 .UNSPECIFIED. ) ;
#4829=VERTEX_POINT ( 'NONE', #157128 ) ;
#4836=SURFACE_SIDE_STYLE ('',( #105612 ) ) ;
#4847=FILL_AREA_STYLE ('',( #86143 ) ) ;
#4875=DIRECTION ( 'NONE',  ( 0.000000000000000000, 0.000000000000000000, -1.000000000000000000 ) ) ;
#4898=CARTESIAN_POINT ( 'NONE',  ( -11.21884318011362147, 9.005685702144777594, -2.479759622982018463 ) ) ;
#4909=ORIENTED_EDGE ( 'NONE', *, *, #72896, .F. ) ;
#4914=DIRECTION ( 'NONE',  ( 1.000000000000000000, -0.000000000000000000, -0.000000000000000000 ) ) ;
#4937=SURFACE_STYLE_USAGE ( .BOTH. , #35333 ) ;
#4980=B_SPLINE_CURVE_WITH_KNOTS ( 'NONE', 3,
 ( #104074, #204735, #20656, #38002, #186367, #205819, #87819 ),
 .UNSPECIFIED., .F., .F.,
 ( 4, 3, 4 ),
 ( 6.324901595874412133E-18, 3.303462137167311185E-05, 4.225156140141500603E-05 ),
 .UNSPECIFIED. ) ;
#4997=ORIENTED_EDGE ( 'NONE', *, *, #104111, .F. ) ;
#5006=DIRECTION ( 'NONE',  ( -0.000000000000000000, -1.000000000000000000, -0.000000000000000000 ) ) ;
#5007=CARTESIAN_POINT ( 'NONE',  ( -11.27976636440881641, 5.060096319113082330, -5.788224378391188196 ) ) ;
#5019=FILL_AREA_STYLE ('',( #166486 ) ) ;
#5025=CARTESIAN_POINT ( 'NONE',  ( 11.99989096720821991, 6.571554264009413338, 0.5037914602360314964 ) ) ;
#5039=ORIENTED_EDGE ( 'NONE', *, *, #19138, .T. ) ;
#5045=CARTESIAN_POINT ( 'NONE',  ( -9.345718720454772921, 15.44302540324981976, 7.452154232107743859 ) ) ;
#5048=CARTESIAN_POINT ( 'NONE',  ( -8.771960149507961546, 15.44694760938148548, -8.173204598701103052 ) ) ;
#5088=DIRECTION ( 'NONE',  ( -0.000000000000000000, 1.000000000000000000, 0.000000000000000000 ) ) ;
#5118=( LENGTH_UNIT ( ) NAMED_UNIT ( * ) SI_UNIT ( .MILLI., .METRE. ) );
#5186=PRESENTATION_STYLE_ASSIGNMENT (( #8411 ) ) ;
#5190=ORIENTED_EDGE ( 'NONE', *, *, #154855, .F. ) ;
#5195=( NAMED_UNIT ( * ) SI_UNIT ( $, .STERADIAN. ) SOLID_ANGLE_UNIT ( ) );
#5203=CIRCLE ( 'NONE', #147041, 12.00000000000000178 ) ;
#5223=AXIS2_PLACEMENT_3D ( 'NONE', #188377, #207821, #58390 ) ;
#5255=EDGE_CURVE ( 'NONE', #20303, #8789, #204233, .T. ) ;
#5258=AXIS2_PLACEMENT_3D ( 'NONE', #56140, #70223, #39899 ) ;
#5285=CARTESIAN_POINT ( 'NONE',  ( 11.88156762547254175, 13.87999991545966516, 1.686557021358693786 ) ) ;
#5290=SURFACE_SIDE_STYLE ('',( #7441 ) ) ;
#5291=CARTESIAN_POINT ( 'NONE',  ( -10.40865662669954084, 4.028931174475638421, 7.242212795919873436 ) ) ;
#5324=ORIENTED_EDGE ( 'NONE', *, *, #193355, .T. ) ;
#5330=FACE_BOUND ( 'NONE', #144187, .T. ) ;
#5337=DIRECTION ( 'NONE',  ( 0.5994789404140788980, 1.518179186858609835E-15, -0.8003905296791143931 ) ) ;
#5355=CIRCLE ( 'NONE', #209464, 0.08000000000000015432 ) ;
#5373=DIRECTION ( 'NONE',  ( -1.124869321039521280E-29, -7.437565543542506798E-15, -1.000000000000000000 ) ) ;
#5390=CARTESIAN_POINT ( 'NONE',  ( -8.799907370706367971, 15.46908217234898153, 8.208919216386629358 ) ) ;
#5418=ORIENTED_EDGE ( 'NONE', *, *, #51505, .F. ) ;
#5438=CARTESIAN_POINT ( 'NONE',  ( -10.77299012366456310, 5.423410747438590640, 6.621146351739780833 ) ) ;
#5452=ORIENTED_EDGE ( 'NONE', *, *, #138983, .T. ) ;
#5467=CARTESIAN_POINT ( 'NONE',  ( -9.568429106564499520, 15.10400138847699303, -7.242208005537321469 ) ) ;
#5476=ORIENTED_EDGE ( 'NONE', *, *, #125755, .T. ) ;
#5489=CARTESIAN_POINT ( 'NONE',  ( -3.447813423226582241, 14.52993373270244248, 11.50294194160398753 ) ) ;
#5496=CARTESIAN_POINT ( 'NONE',  ( -11.86239285000045918, 9.719999999999982876, 1.812080536912751061 ) ) ;
#5500=CARTESIAN_POINT ( 'NONE',  ( 11.86145016429273369, 13.50587408513255383, 1.099999999999996758 ) ) ;
#5518=CARTESIAN_POINT ( 'NONE',  ( 11.80235830595197655, 11.29999999999998117, 1.696088231482818065 ) ) ;
#5519=DIRECTION ( 'NONE',  ( -0.000000000000000000, -1.000000000000000000, -0.000000000000000000 ) ) ;
#5529=AXIS2_PLACEMENT_3D ( 'NONE', #173864, #210596, #141386 ) ;
#5540=FILL_AREA_STYLE ('',( #20737 ) ) ;
#5570=SURFACE_STYLE_USAGE ( .BOTH. , #189686 ) ;
#5571=CARTESIAN_POINT ( 'NONE',  ( -11.04433755984576848, 5.142917986253679352, 4.203129294766247526 ) ) ;
#5582=CARTESIAN_POINT ( 'NONE',  ( 11.73212044392280262, 8.686627382477217552, -4.360314433000339385 ) ) ;
#5602=LINE ( 'NONE', #35998, #143466 ) ;
#5613=VECTOR ( 'NONE', #152995, 1000.000000000000000 ) ;
#5634=CARTESIAN_POINT ( 'NONE',  ( 11.07123604129543359, 12.30000000000000249, 0.8055550039003240848 ) ) ;
#5638=CARTESIAN_POINT ( 'NONE',  ( -11.48243876534946217, 13.87999999999998302, 3.199999999999997957 ) ) ;
#5686=CARTESIAN_POINT ( 'NONE',  ( 9.220166054920730048, 13.21238179712012517, -9.025879716107306550 ) ) ;
#5704=EDGE_LOOP ( 'NONE', ( #210630, #106119, #15688, #178224 ) ) ;
#5717=EDGE_CURVE ( 'NONE', #200740, #3699, #112531, .T. ) ;
#5734=PLANE ( 'NONE',  #209870 ) ;
#5743=CARTESIAN_POINT ( 'NONE',  ( 0.000000000000000000, 18.91999999999999815, 0.000000000000000000 ) ) ;
#5822=CARTESIAN_POINT ( 'NONE',  ( -11.44800751630026880, 13.79999999999998295, 3.302956944461236777 ) ) ;
#5824=B_SPLINE_CURVE_WITH_KNOTS ( 'NONE', 3,
 ( #7897, #90247, #89187, #73985, #139004, #57736, #140080, #205026, #77174, #155238, #174713, #56672, #209287, #121752, #40433, #107618, #8978, #92401, #206103, #173649, #39348, #25223, #91326, #157386, #75052, #43644, #141166, #190916, #207175, #124954 ),
 .UNSPECIFIED., .F., .F.,
 ( 4, 2, 2, 2, 2, 2, 2, 2, 2, 2, 2, 2, 2, 2, 4 ),
 ( 0.3904182756812821231, 0.3921283039710705687, 0.3938383322608589587, 0.3972583888404358499, 0.4040985019995896321, 0.4177787283178971967, 0.4451391809545123257, 0.4999364453639513206, 0.5547656701200603946, 0.5821739285757332460, 0.5958780578035696163, 0.6027301224174878014, 0.6061561547244469494, 0.6078691708779264680, 0.6095821870314059865 ),
 .UNSPECIFIED. ) ;
#5831=CIRCLE ( 'NONE', #113094, 0.08000000000000014044 ) ;
#5841=CARTESIAN_POINT ( 'NONE',  ( -11.33772465723282785, 10.09131699265171278, -3.600000000000076472 ) ) ;
#5856=CARTESIAN_POINT ( 'NONE',  ( -10.62873463776380234, 9.799999999999982947, 3.199999999999997957 ) ) ;
#5862=( NAMED_UNIT ( * ) PLANE_ANGLE_UNIT ( ) SI_UNIT ( $, .RADIAN. ) );
#5922=FILL_AREA_STYLE_COLOUR ( '', #102666 ) ;
#5933=CARTESIAN_POINT ( 'NONE',  ( 9.412522317677918693, 11.54714845510762267, -7.460155439063340665 ) ) ;
#5940=CARTESIAN_POINT ( 'NONE',  ( 9.663580702207960726, 13.51594383518721365, 8.187698013202092895 ) ) ;
#5960=CARTESIAN_POINT ( 'NONE',  ( 11.96535697748077887, 9.847373329355470162, 0.9148528286454596925 ) ) ;
#5974=CARTESIAN_POINT ( 'NONE',  ( -11.15881748666195072, 6.758040191959135079, 5.811769976250384495 ) ) ;
#5975=AXIS2_PLACEMENT_3D ( 'NONE', #125796, #123675, #208014 ) ;
#6003=ORIENTED_EDGE ( 'NONE', *, *, #129984, .T. ) ;
#6019=DIRECTION ( 'NONE',  ( 0.000000000000000000, 0.000000000000000000, -1.000000000000000000 ) ) ;
#6048=EDGE_CURVE ( 'NONE', #44585, #1117, #134517, .T. ) ;
#6072=VECTOR ( 'NONE', #69836, 1000.000000000000000 ) ;
#6084=CARTESIAN_POINT ( 'NONE',  ( -10.71748749772954135, 5.309591131546671505, -6.727448623506740333 ) ) ;
#6096=CARTESIAN_POINT ( 'NONE',  ( -11.14501278000869355, 7.223412960316487386, -3.546411330735405265 ) ) ;
#6121=CARTESIAN_POINT ( 'NONE',  ( 1.500000000000035971, 7.750000000000000000, 10.99818166789401275 ) ) ;
#6126=EDGE_LOOP ( 'NONE', ( #42355, #112917, #69573, #134900 ) ) ;
#6129=DIRECTION ( 'NONE',  ( 0.000000000000000000, -1.000000000000000000, -9.023263958591317418E-17 ) ) ;
#6145=ORIENTED_EDGE ( 'NONE', *, *, #69227, .T. ) ;
#6171=CARTESIAN_POINT ( 'NONE',  ( -9.587917471435847716, 4.026361754648488223, -6.670783315233271615 ) ) ;
#6177=VERTEX_POINT ( 'NONE', #87865 ) ;
#6225=VECTOR ( 'NONE', #14403, 1000.000000000000000 ) ;
#6243=STYLED_ITEM ( 'NONE', ( #12046 ), #202610 ) ;
#6244=CIRCLE ( 'NONE', #51117, 0.08000000000000020983 ) ;
#6263=DIRECTION ( 'NONE',  ( 0.000000000000000000, 0.000000000000000000, -1.000000000000000000 ) ) ;
#6272=FACE_OUTER_BOUND ( 'NONE', #116734, .T. ) ;
#6285=VECTOR ( 'NONE', #132442, 1000.000000000000000 ) ;
#6305=EDGE_CURVE ( 'NONE', #19175, #99973, #137695, .T. ) ;
#6321=CARTESIAN_POINT ( 'NONE',  ( -1.500000000000038636, 7.750000000000000000, -10.64483442802187341 ) ) ;
#6355=CARTESIAN_POINT ( 'NONE',  ( 11.52460864928264783, 13.87999999999999723, -3.346683403123526190 ) ) ;
#6358=FACE_OUTER_BOUND ( 'NONE', #202985, .T. ) ;
#6375=CARTESIAN_POINT ( 'NONE',  ( -9.348561386651960348, 2.999999999999999112, 7.001914024036568485 ) ) ;
#6385=EDGE_LOOP ( 'NONE', ( #14648, #122426, #53005, #29470 ) ) ;
#6405=ORIENTED_EDGE ( 'NONE', *, *, #209722, .T. ) ;
#6415=( NAMED_UNIT ( * ) SI_UNIT ( $, .STERADIAN. ) SOLID_ANGLE_UNIT ( ) );
#6426=PLANE ( 'NONE',  #164910 ) ;
#6427=CARTESIAN_POINT ( 'NONE',  ( -11.94105721237523099, 10.90000000000000036, -1.187919463087249827 ) ) ;
#6486=CARTESIAN_POINT ( 'NONE',  ( 11.01931693160843118, 9.191946463694739222, 4.624380626795012716 ) ) ;
#6507=SURFACE_STYLE_FILL_AREA ( #169027 ) ;
#6508=ADVANCED_FACE ( 'NONE', ( #60686 ), #119494, .T. ) ;
#6517=CARTESIAN_POINT ( 'NONE',  ( -11.05071387823260487, 4.509444648491869323, 6.218574854545789066 ) ) ;
#6532=DIRECTION ( 'NONE',  ( 0.000000000000000000, -9.023263958591316185E-17, 1.000000000000000000 ) ) ;
#6534=AXIS2_PLACEMENT_3D ( 'NONE', #87452, #5088, #170826 ) ;
#6549=CIRCLE ( 'NONE', #89152, 11.09999999999999964 ) ;
#6555=LINE ( 'NONE', #139807, #74618 ) ;
#6564=EDGE_CURVE ( 'NONE', #45616, #11502, #160330, .T. ) ;
#6571=CARTESIAN_POINT ( 'NONE',  ( -11.44789321844504215, 9.800000000000000711, -3.303298730975397834 ) ) ;
#6598=VECTOR ( 'NONE', #206948, 1000.000000000000000 ) ;
#6600=DIRECTION ( 'NONE',  ( 1.000000000000000000, -0.000000000000000000, -0.000000000000000000 ) ) ;
#6610=EDGE_CURVE ( 'NONE', #7772, #62106, #136314, .T. ) ;
#6623=( NAMED_UNIT ( * ) PLANE_ANGLE_UNIT ( ) SI_UNIT ( $, .RADIAN. ) );
#6635=DIRECTION ( 'NONE',  ( 0.000000000000000000, -7.254698431505058073E-17, 1.000000000000000000 ) ) ;
#6649=CARTESIAN_POINT ( 'NONE',  ( 10.97010717055062479, 13.80000000000000071, -1.696399592028411396 ) ) ;
#6651=AXIS2_PLACEMENT_3D ( 'NONE', #173243, #146076, #207837 ) ;
#6655=( NAMED_UNIT ( * ) SI_UNIT ( $, .STERADIAN. ) SOLID_ANGLE_UNIT ( ) );
#6656=CARTESIAN_POINT ( 'NONE',  ( -11.69380381030441107, 8.410673437356566140, -1.083569014401829955 ) ) ;
#6669=CARTESIAN_POINT ( 'NONE',  ( 11.89204169242350595, 12.30000000000000071, 0.8046421800351223341 ) ) ;
#6723=PRESENTATION_STYLE_ASSIGNMENT (( #156218 ) ) ;
#6727=AXIS2_PLACEMENT_3D ( 'NONE', #5743, #88104, #20933 ) ;
#6764=CARTESIAN_POINT ( 'NONE',  ( 9.228859063121788608, 14.17280082594779600, 7.673751449575783035 ) ) ;
#6825=CARTESIAN_POINT ( 'NONE',  ( -6.756024855156518072, 14.53008480311059714, -9.927621727203854718 ) ) ;
#6870=CARTESIAN_POINT ( 'NONE',  ( -11.97929049433705373, 12.22000000000000064, 0.7046979865771804130 ) ) ;
#6920=ORIENTED_EDGE ( 'NONE', *, *, #131120, .T. ) ;
#6922=CARTESIAN_POINT ( 'NONE',  ( 9.651614352920288908, 4.121347559867349020, -7.130841425383052545 ) ) ;
#6932=CARTESIAN_POINT ( 'NONE',  ( -11.94041551183581262, 8.961066757473448163, 1.233743901448089764 ) ) ;
#7002=CARTESIAN_POINT ( 'NONE',  ( 8.983336459935364005, 13.98445560454119629, 7.957668677609153640 ) ) ;
#7007=CARTESIAN_POINT ( 'NONE',  ( -11.52460864928265138, 12.21999999999999709, -3.346683403123526190 ) ) ;
#7010=CARTESIAN_POINT ( 'NONE',  ( 8.131154284199636706, 15.75938775753455801, 8.460579169278151568 ) ) ;
#7043=CARTESIAN_POINT ( 'NONE',  ( -11.88731729969462059, 7.000411858491159656, -4.404230128874679906 ) ) ;
#7050=EDGE_CURVE ( 'NONE', #35130, #78193, #53410, .T. ) ;
#7053=( NAMED_UNIT ( * ) SI_UNIT ( $, .STERADIAN. ) SOLID_ANGLE_UNIT ( ) );
#7060=CARTESIAN_POINT ( 'NONE',  ( 11.41381675112453387, 10.90000000000000036, -3.704697986577182522 ) ) ;
#7085=DIRECTION ( 'NONE',  ( 0.000000000000000000, 0.000000000000000000, -1.000000000000000000 ) ) ;
#7149=ORIENTED_EDGE ( 'NONE', *, *, #82737, .F. ) ;
#7154=CARTESIAN_POINT ( 'NONE',  ( -11.96215121607992593, 11.32833553780823799, -0.9565349792967606790 ) ) ;
#7157=DIRECTION ( 'NONE',  ( 1.000000000000000000, -0.000000000000000000, -0.000000000000000000 ) ) ;
#7162=ADVANCED_FACE ( 'NONE', ( #144223 ), #84647, .T. ) ;
#7167=CARTESIAN_POINT ( 'NONE',  ( -10.93377262805118555, 5.994763374826558966, -6.297255446303106297 ) ) ;
#7238=CARTESIAN_POINT ( 'NONE',  ( -9.348561386899501002, 3.999985931113709814, -7.001914024221969512 ) ) ;
#7255=LINE ( 'NONE', #60291, #96440 ) ;
#7290=DIRECTION ( 'NONE',  ( 0.1653894851707868319, -0.9636043447860246358, -0.2100309141636969024 ) ) ;
#7322=ADVANCED_FACE ( 'NONE', ( #68216 ), #52000, .F. ) ;
#7335=CARTESIAN_POINT ( 'NONE',  ( 0.000000000000000000, 12.22000000000000064, 0.000000000000000000 ) ) ;
#7341=CARTESIAN_POINT ( 'NONE',  ( 11.07790593930098311, 13.79999999999999893, -0.7000000000000009548 ) ) ;
#7342=CARTESIAN_POINT ( 'NONE',  ( 11.94980361723123785, 11.00238056585436652, 1.099999926404769290 ) ) ;
#7359=FILL_AREA_STYLE_COLOUR ( '', #175023 ) ;
#7370=( LENGTH_UNIT ( ) NAMED_UNIT ( * ) SI_UNIT ( .MILLI., .METRE. ) );
#7392=CIRCLE ( 'NONE', #55803, 12.00000000000000178 ) ;
#7412=DIRECTION ( 'NONE',  ( 0.000000000000000000, 1.000000000000000000, 0.000000000000000000 ) ) ;
#7415=CARTESIAN_POINT ( 'NONE',  ( 9.649519325286297189, 4.269047477884574171, 7.134145662718395897 ) ) ;
#7425=CARTESIAN_POINT ( 'NONE',  ( -11.92050416151433012, 9.947946247203631742, 1.381922468431395767 ) ) ;
#7441=SURFACE_STYLE_FILL_AREA ( #173185 ) ;
#7442=CARTESIAN_POINT ( 'NONE',  ( -10.47051000334347570, 4.046481986658133856, 7.152373939818348347 ) ) ;
#7445=( BOUNDED_SURFACE ( )  B_SPLINE_SURFACE ( 3, 2, ( 
 ( #108228, #91935, #21537 ),
 ( #87647, #153717, #5285 ),
 ( #10634, #127699, #109297 ),
 ( #29043, #61533, #193659 ),
 ( #110359, #176363, #76710 ),
 ( #43184, #126620, #192583 ) ),
 .UNSPECIFIED., .F., .F., .T. ) 
 B_SPLINE_SURFACE_WITH_KNOTS ( ( 4, 2, 4 ),
 ( 3, 3 ),
 ( 0.000000000000000000, 0.0003766405729503175871, 0.0007532811459006351741 ),
 ( 0.000000000000000000, 1.000000000000000000 ),
 .UNSPECIFIED. ) 
 GEOMETRIC_REPRESENTATION_ITEM ( )  RATIONAL_B_SPLINE_SURFACE ( (
 ( 1.000000000000000000, 0.7071067811865551223, 1.000000000000000000),
 ( 1.000000000000000000, 0.7211294902950703412, 1.000000000000000000),
 ( 1.000000000000000000, 0.7311181975234362085, 1.000000000000000000),
 ( 1.000000000000000000, 0.7429553055057509514, 1.000000000000000000),
 ( 1.000000000000000000, 0.7451698531061192732, 1.000000000000000000),
 ( 1.000000000000000000, 0.7452309222763021657, 1.000000000000000000) ) ) 
 REPRESENTATION_ITEM ( '' )  SURFACE ( )  );
#7450=AXIS2_PLACEMENT_3D ( 'NONE', #119670, #169424, #134819 ) ;
#7468=CARTESIAN_POINT ( 'NONE',  ( 0.000000000000000000, 12.29999999999998295, 0.000000000000000000 ) ) ;
#7481=CARTESIAN_POINT ( 'NONE',  ( 11.92045683181315674, 11.15275927879483220, 1.382340670101856350 ) ) ;
#7490=( NAMED_UNIT ( * ) SI_UNIT ( $, .STERADIAN. ) SOLID_ANGLE_UNIT ( ) );
#7494=CARTESIAN_POINT ( 'NONE',  ( -8.752316528461410172, 14.55265192235988536, 8.156921273040330433 ) ) ;
#7507=VECTOR ( 'NONE', #53106, 1000.000000000000000 ) ;
#7510=CARTESIAN_POINT ( 'NONE',  ( -10.51337128857758074, 4.000503439385035165, 5.786193332252632437 ) ) ;
#7513=ORIENTED_EDGE ( 'NONE', *, *, #197258, .F. ) ;
#7519=CARTESIAN_POINT ( 'NONE',  ( 1.734723475976807292E-15, 15.42691958146951414, 11.91973154060106665 ) ) ;
#7553=CARTESIAN_POINT ( 'NONE',  ( 11.41381675112453387, 19.00000000000000000, -3.704697986577182522 ) ) ;
#7565=VERTEX_POINT ( 'NONE', #136459 ) ;
#7569=EDGE_CURVE ( 'NONE', #18531, #71097, #98950, .T. ) ;
#7581=CARTESIAN_POINT ( 'NONE',  ( 11.41381675112453387, 12.69999999999999929, -3.704697986577184299 ) ) ;
#7586=CARTESIAN_POINT ( 'NONE',  ( -10.39851513827935747, 3.504673854002353206, 5.419231829292963099 ) ) ;
#7587=EDGE_LOOP ( 'NONE', ( #123989, #41831, #16770, #109642 ) ) ;
#7602=CARTESIAN_POINT ( 'NONE',  ( -15.75000000000000000, 13.79999999999999893, -0.7000000000000009548 ) ) ;
#7604=AXIS2_PLACEMENT_3D ( 'NONE', #94446, #62976, #101876 ) ;
#7621=FACE_OUTER_BOUND ( 'NONE', #13282, .T. ) ;
#7627=CARTESIAN_POINT ( 'NONE',  ( 11.97929049433705373, 13.88000000000000078, 0.7046979865771804130 ) ) ;
#7637=CARTESIAN_POINT ( 'NONE',  ( -10.06363042846879807, 3.665155796981559355, -6.455816864028870228 ) ) ;
#7640=DIRECTION ( 'NONE',  ( 0.05872483221476467591, 7.952201780260630618E-17, 0.9982742078614211811 ) ) ;
#7643=CARTESIAN_POINT ( 'NONE',  ( -11.84668729035137069, 11.00518580017409143, 1.399999999999998357 ) ) ;
#7651=VECTOR ( 'NONE', #194721, 1000.000000000000000 ) ;
#7674=VERTEX_POINT ( 'NONE', #158041 ) ;
#7675=CARTESIAN_POINT ( 'NONE',  ( 0.000000000000000000, 13.87999999999998302, 0.000000000000000000 ) ) ;
#7704=CARTESIAN_POINT ( 'NONE',  ( 7.032125997333287692, 15.00041888085534758, 9.944927957745147040 ) ) ;
#7706=CARTESIAN_POINT ( 'NONE',  ( 11.44786932348528907, 9.799999999999998934, -3.303370173849653035 ) ) ;
#7711=VERTEX_POINT ( 'NONE', #8562 ) ;
#7713=ORIENTED_EDGE ( 'NONE', *, *, #70219, .F. ) ;
#7720=ADVANCED_FACE ( 'NONE', ( #74642 ), #56262, .F. ) ;
#7726=CARTESIAN_POINT ( 'NONE',  ( -11.04445182892037813, 5.143275749589305335, -4.203165840917552742 ) ) ;
#7728=CARTESIAN_POINT ( 'NONE',  ( 7.449721630645223414, 15.00158243878686726, 10.26201403118819044 ) ) ;
#7738=CARTESIAN_POINT ( 'NONE',  ( 11.97185388258315086, 12.22000009279607546, 0.8311143155443657671 ) ) ;
#7740=ORIENTED_EDGE ( 'NONE', *, *, #78129, .T. ) ;
#7744=CARTESIAN_POINT ( 'NONE',  ( 10.62873463776380056, 12.30000000000000071, -3.200000000000001510 ) ) ;
#7755=DIRECTION ( 'NONE',  ( 0.000000000000000000, 1.000000000000000000, 0.000000000000000000 ) ) ;
#7772=VERTEX_POINT ( 'NONE', #122420 ) ;
#7776=LINE ( 'NONE', #173529, #53129 ) ;
#7794=CYLINDRICAL_SURFACE ( 'NONE', #162836, 10.75000000000000000 ) ;
#7822=CIRCLE ( 'NONE', #35498, 11.68000000000000149 ) ;
#7835=CARTESIAN_POINT ( 'NONE',  ( 9.427850895902814443, 13.54474674066948481, 7.423989997610747515 ) ) ;
#7839=( NAMED_UNIT ( * ) PLANE_ANGLE_UNIT ( ) SI_UNIT ( $, .RADIAN. ) );
#7860=EDGE_LOOP ( 'NONE', ( #175725, #207513, #107386, #19877, #104616, #115424 ) ) ;
#7897=CARTESIAN_POINT ( 'NONE',  ( -10.44369227015510049, 5.112964020592959180, 5.232143560358710310 ) ) ;
#7901=CARTESIAN_POINT ( 'NONE',  ( -8.803307360466531506, 14.48154073751409499, -8.204672630978624426 ) ) ;
#7906=DIRECTION ( 'NONE',  ( -0.000000000000000000, 1.000000000000000000, -0.000000000000000000 ) ) ;
#7913=EDGE_CURVE ( 'NONE', #139957, #62806, #110663, .T. ) ;
#7940=CARTESIAN_POINT ( 'NONE',  ( -11.84668730067608422, 13.40000000000000036, -1.320000000000001616 ) ) ;
#7964=SURFACE_STYLE_USAGE ( .BOTH. , #57801 ) ;
#7968=VERTEX_POINT ( 'NONE', #167592 ) ;
#7979=EDGE_LOOP ( 'NONE', ( #85596, #131208, #146291, #20492 ) ) ;
#7987=AXIS2_PLACEMENT_3D ( 'NONE', #124601, #59503, #93101 ) ;
#7988=CARTESIAN_POINT ( 'NONE',  ( 8.417021892111831605, 12.86188997900043596, -8.495519444159276290 ) ) ;
#7991=CARTESIAN_POINT ( 'NONE',  ( -11.43190902327450509, 9.944778717421446146, -3.649704988378223991 ) ) ;
#7994=ORIENTED_EDGE ( 'NONE', *, *, #110028, .T. ) ;
#8003=CARTESIAN_POINT ( 'NONE',  ( 9.649010003797926061, 3.730310916805920751, -7.134817918383260071 ) ) ;
#8013=DIRECTION ( 'NONE',  ( 0.000000000000000000, 0.000000000000000000, -1.000000000000000000 ) ) ;
#8053=CARTESIAN_POINT ( 'NONE',  ( 0.000000000000000000, 4.518467169708412889, 0.000000000000000000 ) ) ;
#8066=ORIENTED_EDGE ( 'NONE', *, *, #173298, .T. ) ;
#8072=( LENGTH_UNIT ( ) NAMED_UNIT ( * ) SI_UNIT ( .MILLI., .METRE. ) );
#8079=PLANE ( 'NONE',  #88919 ) ;
#8098=CARTESIAN_POINT ( 'NONE',  ( 9.246599373783906728, 13.75186350236544008, 6.856982591890075085 ) ) ;
#8133=CARTESIAN_POINT ( 'NONE',  ( -10.83922355283164229, 5.627439893072521571, -6.488667358217314884 ) ) ;
#8135=AXIS2_PLACEMENT_3D ( 'NONE', #26444, #24290, #92554 ) ;
#8150=CARTESIAN_POINT ( 'NONE',  ( 0.000000000000000000, 0.000000000000000000, 0.000000000000000000 ) ) ;
#8161=ORIENTED_EDGE ( 'NONE', *, *, #209369, .T. ) ;
#8173=FACE_BOUND ( 'NONE', #130131, .T. ) ;
#8209=CARTESIAN_POINT ( 'NONE',  ( -10.50000000000000000, 10.89999999999998259, 3.599999999999999201 ) ) ;
#8227=AXIS2_PLACEMENT_3D ( 'NONE', #91337, #213301, #126026 ) ;
#8233=ORIENTED_EDGE ( 'NONE', *, *, #206552, .T. ) ;
#8241=CARTESIAN_POINT ( 'NONE',  ( -15.75000000000000000, 13.39999999999998259, 1.799999999999999600 ) ) ;
#8243=CARTESIAN_POINT ( 'NONE',  ( 11.94105721237523277, 13.40000000000000036, -1.187919463087249827 ) ) ;
#8249=CARTESIAN_POINT ( 'NONE',  ( -10.07169253693141897, 5.946554136026001913, 5.792750394403223702 ) ) ;
#8255=CARTESIAN_POINT ( 'NONE',  ( 6.928203230275514990, 14.48195938056239385, 9.797958971132711525 ) ) ;
#8265=ORIENTED_EDGE ( 'NONE', *, *, #28369, .T. ) ;
#8290=VECTOR ( 'NONE', #86267, 1000.000000000000000 ) ;
#8291=CYLINDRICAL_SURFACE ( 'NONE', #128927, 0.3999999999999997446 ) ;
#8300=( BOUNDED_SURFACE ( )  B_SPLINE_SURFACE ( 3, 2, ( 
 ( #163682, #110725, #210271 ),
 ( #197221, #15264, #132268 ),
 ( #114976, #194027, #129132 ),
 ( #113930, #146383, #97624 ),
 ( #61909, #195108, #30484 ),
 ( #46744, #81351, #131233 ) ),
 .UNSPECIFIED., .F., .F., .F. ) 
 B_SPLINE_SURFACE_WITH_KNOTS ( ( 4, 2, 4 ),
 ( 3, 3 ),
 ( 0.000000000000000000, 0.0003754691837024766443, 0.0007509383674049532886 ),
 ( 0.000000000000000000, 1.000000000000000000 ),
 .UNSPECIFIED. ) 
 GEOMETRIC_REPRESENTATION_ITEM ( )  RATIONAL_B_SPLINE_SURFACE ( (
 ( 1.000000000000000000, 0.6711954675835484219, 1.000000000000000000),
 ( 1.000000000000000000, 0.6709646295272747585, 1.000000000000000000),
 ( 1.000000000000000000, 0.6771840716652173242, 1.000000000000000000),
 ( 1.000000000000000000, 0.6927481755874340674, 1.000000000000000000),
 ( 1.000000000000000000, 0.7017972101304913446, 1.000000000000000000),
 ( 1.000000000000000000, 0.7071067811865399122, 1.000000000000000000) ) ) 
 REPRESENTATION_ITEM ( '' )  SURFACE ( )  );
#8325=CARTESIAN_POINT ( 'NONE',  ( -9.541882734523161602, 5.027466607964795386, -6.730450668810338044 ) ) ;
#8377=EDGE_LOOP ( 'NONE', ( #172657, #93375, #55514, #112718 ) ) ;
#8388=CARTESIAN_POINT ( 'NONE',  ( 11.78331023100045627, 13.79999999999999893, -1.800000000000001155 ) ) ;
#8411=SURFACE_STYLE_USAGE ( .BOTH. , #141670 ) ;
#8423=DIRECTION ( 'NONE',  ( -0.000000000000000000, 1.000000000000000000, -0.000000000000000000 ) ) ;
#8436=( LENGTH_UNIT ( ) NAMED_UNIT ( * ) SI_UNIT ( .MILLI., .METRE. ) );
#8444=AXIS2_PLACEMENT_3D ( 'NONE', #3451, #103118, #83650 ) ;
#8448=CARTESIAN_POINT ( 'NONE',  ( 11.33772465723237666, 10.09131699265169146, 3.600000000000073364 ) ) ;
#8456=FILL_AREA_STYLE_COLOUR ( '', #110720 ) ;
#8482=EDGE_LOOP ( 'NONE', ( #56450, #139771, #96590, #210350 ) ) ;
#8499=CIRCLE ( 'NONE', #181367, 0.07999999999999998779 ) ;
#8505=CARTESIAN_POINT ( 'NONE',  ( -11.81907076198591966, 9.842687754035246428, 1.592066415281218505 ) ) ;
#8520=PRESENTATION_STYLE_ASSIGNMENT (( #171025 ) ) ;
#8521=CARTESIAN_POINT ( 'NONE',  ( -11.38450596090590849, 3.710255710271473273, 5.708599601896569453 ) ) ;
#8528=EDGE_CURVE ( 'NONE', #45649, #29327, #145119, .T. ) ;
#8555=ORIENTED_EDGE ( 'NONE', *, *, #39340, .F. ) ;
#8562=CARTESIAN_POINT ( 'NONE',  ( -11.84668730067608600, 10.19999999999999929, -1.400000000000001910 ) ) ;
#8575=CARTESIAN_POINT ( 'NONE',  ( 11.86145016429272836, 10.90000000000000036, -1.180000000000002158 ) ) ;
#8576=FILL_AREA_STYLE_COLOUR ( '', #160658 ) ;
#8580=CARTESIAN_POINT ( 'NONE',  ( 9.601932019700244680, 4.115787151892719820, 7.121345993713853240 ) ) ;
#8598=SURFACE_STYLE_FILL_AREA ( #41135 ) ;
#8616=CARTESIAN_POINT ( 'NONE',  ( -5.577074488906905714, 15.46905280921072467, 10.63472345728874835 ) ) ;
#8626=ORIENTED_EDGE ( 'NONE', *, *, #1482, .T. ) ;
#8628=CARTESIAN_POINT ( 'NONE',  ( -10.95308175811721085, 13.79999999999999893, -1.800000000000001155 ) ) ;
#8632=CARTESIAN_POINT ( 'NONE',  ( 10.80547401163854460, 9.581360759087717227, 5.116132519491706887 ) ) ;
#8654=AXIS2_PLACEMENT_3D ( 'NONE', #50930, #51999, #37875 ) ;
#8657=FILL_AREA_STYLE_COLOUR ( '', #167590 ) ;
#8666=VERTEX_POINT ( 'NONE', #162705 ) ;
#8680=FACE_OUTER_BOUND ( 'NONE', #108782, .T. ) ;
#8714=DIRECTION ( 'NONE',  ( 0.000000000000000000, 0.000000000000000000, 1.000000000000000000 ) ) ;
#8752=CARTESIAN_POINT ( 'NONE',  ( 0.000000000000000000, 19.00000000000000000, 0.000000000000000000 ) ) ;
#8754=DIRECTION ( 'NONE',  ( -0.000000000000000000, -1.000000000000000000, -0.000000000000000000 ) ) ;
#8755=ORIENTED_EDGE ( 'NONE', *, *, #207217, .T. ) ;
#8757=MECHANICAL_DESIGN_GEOMETRIC_PRESENTATION_REPRESENTATION('',(#195542),#98904);
#8789=VERTEX_POINT ( 'NONE', #79668 ) ;
#8791=AXIS2_PLACEMENT_3D ( 'NONE', #173451, #56481, #6635 ) ;
#8803=FILL_AREA_STYLE_COLOUR ( '', #35287 ) ;
#8807=CARTESIAN_POINT ( 'NONE',  ( -11.48243876534946217, 13.79999999999998295, 3.199999999999997957 ) ) ;
#8815=VECTOR ( 'NONE', #127497, 1000.000000000000000 ) ;
#8830=CARTESIAN_POINT ( 'NONE',  ( -11.44786932348563901, 13.79999999999999893, -3.303370173849772051 ) ) ;
#8850=CARTESIAN_POINT ( 'NONE',  ( 0.000000000000000000, 9.719999999999982876, 0.000000000000000000 ) ) ;
#8889=CARTESIAN_POINT ( 'NONE',  ( 11.86239285000045740, 11.37999999999998302, 1.812080536912751061 ) ) ;
#8897=PRESENTATION_STYLE_ASSIGNMENT (( #158372 ) ) ;
#8902=AXIS2_PLACEMENT_3D ( 'NONE', #55554, #61679, #171434 ) ;
#8916=PRESENTATION_STYLE_ASSIGNMENT (( #125961 ) ) ;
#8929=CARTESIAN_POINT ( 'NONE',  ( -7.247736482493301047, 14.00000000000600231, -10.57961706324514850 ) ) ;
#8935=VERTEX_POINT ( 'NONE', #69782 ) ;
#8954=STYLED_ITEM ( 'NONE', ( #189453 ), #7720 ) ;
#8966=CIRCLE ( 'NONE', #12352, 0.08000000000000020983 ) ;
#8977=CARTESIAN_POINT ( 'NONE',  ( 11.80248046418316044, 13.79999999999998295, 1.695421849633139466 ) ) ;
#8978=CARTESIAN_POINT ( 'NONE',  ( -11.52570357830391323, 8.091488070261075194, -2.173620758456770830 ) ) ;
#8982=CARTESIAN_POINT ( 'NONE',  ( -7.093660771577591895, 14.55189863974096554, -9.633804998953056753 ) ) ;
#9043=CARTESIAN_POINT ( 'NONE',  ( -11.48243876534946217, 9.799999999999982947, 3.199999999999997957 ) ) ;
#9046=ORIENTED_EDGE ( 'NONE', *, *, #41548, .F. ) ;
#9048=PRESENTATION_STYLE_ASSIGNMENT (( #7964 ) ) ;
#9058=CARTESIAN_POINT ( 'NONE',  ( -11.41381676900475917, 13.53041960022397916, 3.704697931490214646 ) ) ;
#9062=ADVANCED_FACE ( 'NONE', ( #24091 ), #141106, .F. ) ;
#9070=CARTESIAN_POINT ( 'NONE',  ( 11.30883932465314601, 7.475091753786390569, 3.226902027701133324 ) ) ;
#9074=CARTESIAN_POINT ( 'NONE',  ( -11.45842088241054135, 10.00693529122955283, -3.566211699757781073 ) ) ;
#9086=CARTESIAN_POINT ( 'NONE',  ( 9.534866695232221190, 3.538528462892257309, -7.286654780214764315 ) ) ;
#9099=DIRECTION ( 'NONE',  ( 0.000000000000000000, 0.000000000000000000, 1.000000000000000000 ) ) ;
#9123=DIRECTION ( 'NONE',  ( 1.000000000000000000, -0.000000000000000000, -0.000000000000000000 ) ) ;
#9126=CARTESIAN_POINT ( 'NONE',  ( -8.752560967067513076, 14.99999998465384365, 9.356054886187056496 ) ) ;
#9131=DIRECTION ( 'NONE',  ( -0.000000000000000000, -1.000000000000000000, 0.000000000000000000 ) ) ;
#9137=DIRECTION ( 'NONE',  ( -0.2684563758389304500, -0.000000000000000000, -0.9632918427306581544 ) ) ;
#9166=CARTESIAN_POINT ( 'NONE',  ( 9.086253353280449474, 13.40000000000000036, 7.838367176906169576 ) ) ;
#9173=CARTESIAN_POINT ( 'NONE',  ( 8.788338075491303414, 15.71983230968314871, 9.216794715973650298 ) ) ;
#9208=CARTESIAN_POINT ( 'NONE',  ( -12.36781821011106963, 9.649948393628900334, 1.413879826568002152 ) ) ;
#9210=CIRCLE ( 'NONE', #175283, 11.95586206896552284 ) ;
#9224=EDGE_CURVE ( 'NONE', #208182, #71097, #179294, .T. ) ;
#9235=CARTESIAN_POINT ( 'NONE',  ( 10.65509502169168776, 9.862988198964483644, 5.421291348111367370 ) ) ;
#9246=CARTESIAN_POINT ( 'NONE',  ( 11.04536101718726115, 13.50457272964008482, 1.099999999999998979 ) ) ;
#9255=AXIS2_PLACEMENT_3D ( 'NONE', #116887, #182886, #34503 ) ;
#9284=FILL_AREA_STYLE ('',( #106842 ) ) ;
#9318=EDGE_CURVE ( 'NONE', #14390, #90767, #24263, .T. ) ;
#9324=CARTESIAN_POINT ( 'NONE',  ( -10.99318506637795956, 6.209869560752310669, 6.173358988436974393 ) ) ;
#9346=( BOUNDED_SURFACE ( )  B_SPLINE_SURFACE ( 3, 2, ( 
 ( #194969, #212265, #161421 ),
 ( #144142, #159268, #210134 ),
 ( #62830, #10868, #131102 ),
 ( #197091, #78017, #63899 ),
 ( #163545, #45544, #110594 ),
 ( #13004, #30350, #61777 ) ),
 .UNSPECIFIED., .F., .F., .F. ) 
 B_SPLINE_SURFACE_WITH_KNOTS ( ( 4, 2, 4 ),
 ( 3, 3 ),
 ( 0.000000000000000000, 0.0003831327362561333209, 0.0007662654725122666419 ),
 ( 0.000000000000000000, 1.000000000000000000 ),
 .UNSPECIFIED. ) 
 GEOMETRIC_REPRESENTATION_ITEM ( )  RATIONAL_B_SPLINE_SURFACE ( (
 ( 1.000000000000000000, 0.5879095031487548972, 1.000000000000000000),
 ( 1.000000000000000000, 0.5873691247580644648, 1.000000000000000000),
 ( 1.000000000000000000, 0.6054349545494872586, 1.000000000000000000),
 ( 1.000000000000000000, 0.6533334602768978705, 1.000000000000000000),
 ( 1.000000000000000000, 0.6828746263149305662, 1.000000000000000000),
 ( 1.000000000000000000, 0.7071067811865475727, 1.000000000000000000) ) ) 
 REPRESENTATION_ITEM ( '' )  SURFACE ( )  );
#9365=SURFACE_STYLE_USAGE ( .BOTH. , #41894 ) ;
#9367=DIRECTION ( 'NONE',  ( -0.000000000000000000, 0.000000000000000000, -1.000000000000000000 ) ) ;
#9375=EDGE_LOOP ( 'NONE', ( #56325, #99381, #111070, #54880, #69649, #141268 ) ) ;
#9392=DIRECTION ( 'NONE',  ( 0.000000000000000000, 1.000000000000000000, 0.000000000000000000 ) ) ;
#9397=CARTESIAN_POINT ( 'NONE',  ( -10.36744940472232379, 5.031894517187950555, -7.294791872146300982 ) ) ;
#9403=DIRECTION ( 'NONE',  ( 1.000000000000000000, -0.000000000000000000, -0.000000000000000000 ) ) ;
#9404=ORIENTED_EDGE ( 'NONE', *, *, #80728, .T. ) ;
#9470=FACE_OUTER_BOUND ( 'NONE', #120220, .T. ) ;
#9487=CARTESIAN_POINT ( 'NONE',  ( -9.367496997608871112, 15.42330868759649043, 7.413898975919298806 ) ) ;
#9492=ORIENTED_EDGE ( 'NONE', *, *, #132683, .T. ) ;
#9497=CARTESIAN_POINT ( 'NONE',  ( 11.97178994924802353, 11.37999993797205178, 0.8322011300497306197 ) ) ;
#9498=CARTESIAN_POINT ( 'NONE',  ( 9.006795113616758996, 12.35945717444475278, -7.859917408111167347 ) ) ;
#9508=ORIENTED_EDGE ( 'NONE', *, *, #119125, .T. ) ;
#9514=LINE ( 'NONE', #210899, #29991 ) ;
#9525=CARTESIAN_POINT ( 'NONE',  ( -15.75000000000000000, 9.799999999999982947, 1.799999999999999600 ) ) ;
#9549=AXIS2_PLACEMENT_3D ( 'NONE', #7335, #73412, #156826 ) ;
#9590=CARTESIAN_POINT ( 'NONE',  ( -10.21581353488473987, 4.000000000000001776, 7.512123095767014647 ) ) ;
#9596=CARTESIAN_POINT ( 'NONE',  ( -11.41381675112453387, 10.90000000000000036, -3.704697986577184299 ) ) ;
#9627=DIRECTION ( 'NONE',  ( 0.000000000000000000, 1.000000000000000000, 0.000000000000000000 ) ) ;
#9628=DIRECTION ( 'NONE',  ( 0.000000000000000000, 0.000000000000000000, -1.000000000000000000 ) ) ;
#9641=VECTOR ( 'NONE', #41368, 1000.000000000000000 ) ;
#9646=SURFACE_SIDE_STYLE ('',( #25890 ) ) ;
#9651=CARTESIAN_POINT ( 'NONE',  ( -15.75000000000000000, 10.90000000000000036, -3.200000000000001510 ) ) ;
#9654=CIRCLE ( 'NONE', #130808, 0.07999999999999933553 ) ;
#9656=CARTESIAN_POINT ( 'NONE',  ( -10.52647613395849646, 3.958815601275306406, 5.762288996714484135 ) ) ;
#9666=CARTESIAN_POINT ( 'NONE',  ( -11.04536101718726293, 11.00581235719507411, 1.099999999999996536 ) ) ;
#9685=FACE_OUTER_BOUND ( 'NONE', #36607, .T. ) ;
#9688=( GEOMETRIC_REPRESENTATION_CONTEXT ( 3 ) GLOBAL_UNCERTAINTY_ASSIGNED_CONTEXT ( ( #174663 ) ) GLOBAL_UNIT_ASSIGNED_CONTEXT ( ( #124382, #209785, #28930 ) ) REPRESENTATION_CONTEXT ( 'NONE', 'WORKASPACE' ) );
#9698=FILL_AREA_STYLE_COLOUR ( '', #180717 ) ;
#9700=CARTESIAN_POINT ( 'NONE',  ( 11.75999501215279963, 7.882567973567104147, -2.166920717415847353 ) ) ;
#9702=CIRCLE ( 'NONE', #123918, 0.08000000000000014044 ) ;
#9705=EDGE_CURVE ( 'NONE', #116397, #209056, #27484, .T. ) ;
#9732=CARTESIAN_POINT ( 'NONE',  ( -10.30047605039691128, 4.688744718740807116, 5.507884344589919934 ) ) ;
#9832=SURFACE_SIDE_STYLE ('',( #145216 ) ) ;
#9864=EDGE_CURVE ( 'NONE', #11502, #91840, #197304, .T. ) ;
#9892=CARTESIAN_POINT ( 'NONE',  ( -11.43195036480942051, 13.65524496285257783, -3.649565797774410036 ) ) ;
#9918=CARTESIAN_POINT ( 'NONE',  ( 7.107960593699191421, 14.55347105030218913, 9.616793498005540286 ) ) ;
#9920=ORIENTED_EDGE ( 'NONE', *, *, #56811, .F. ) ;
#9924=FACE_OUTER_BOUND ( 'NONE', #89852, .T. ) ;
#9929=VERTEX_POINT ( 'NONE', #124206 ) ;
#9936=CARTESIAN_POINT ( 'NONE',  ( -11.94105721237523099, 12.69999999999999929, 1.187919463087248273 ) ) ;
#9944=CARTESIAN_POINT ( 'NONE',  ( 11.81911962874442068, 11.25710573484113475, -1.591749704452471326 ) ) ;
#9955=ORIENTED_EDGE ( 'NONE', *, *, #14467, .T. ) ;
#9964=DIRECTION ( 'NONE',  ( 0.05872483221476467591, -7.952201780260630618E-17, -0.9982742078614211811 ) ) ;
#9966=TOROIDAL_SURFACE ( 'NONE', #154844, 11.92000000000000171, 0.08000000000000000167 ) ;
#9990=UNCERTAINTY_MEASURE_WITH_UNIT (LENGTH_MEASURE( 1.000000000000000082E-05 ), #73905, 'distance_accuracy_value', 'NONE');
#9995=VERTEX_POINT ( 'NONE', #26601 ) ;
#10029=EDGE_CURVE ( 'NONE', #84082, #144349, #111127, .T. ) ;
#10082=( LENGTH_UNIT ( ) NAMED_UNIT ( * ) SI_UNIT ( .MILLI., .METRE. ) );
#10099=CARTESIAN_POINT ( 'NONE',  ( -11.41108574530281494, 11.25836855377625589, -3.405883542057589253 ) ) ;
#10111=CARTESIAN_POINT ( 'NONE',  ( 11.99427146011852763, 7.649902820345518606, -0.4312808647509002724 ) ) ;
#10117=FILL_AREA_STYLE ('',( #12248 ) ) ;
#10126=CARTESIAN_POINT ( 'NONE',  ( 8.811349696246875141, 13.35371418836173696, 7.678511501153402641 ) ) ;
#10130=CARTESIAN_POINT ( 'NONE',  ( -5.995491898843540390, 14.48115541367089953, -10.40458799043917359 ) ) ;
#10140=CARTESIAN_POINT ( 'NONE',  ( -0.9040546642425820734, 15.46908217946011455, -11.99999999974921394 ) ) ;
#10157=LINE ( 'NONE', #159624, #161826 ) ;
#10188=CARTESIAN_POINT ( 'NONE',  ( -9.117697077659501659, 15.00000000000574829, 7.299999999990889776 ) ) ;
#10209=CARTESIAN_POINT ( 'NONE',  ( -9.367496997601190145, 14.57669131240758276, 7.413898975931879853 ) ) ;
#10216=( NAMED_UNIT ( * ) SI_UNIT ( $, .STERADIAN. ) SOLID_ANGLE_UNIT ( ) );
#10232=CARTESIAN_POINT ( 'NONE',  ( -11.55950211276791428, 12.22000000000000064, -3.221476510067114329 ) ) ;
#10234=CARTESIAN_POINT ( 'NONE',  ( 7.615526167148707337, 15.99525620954516292, 10.13761593936639294 ) ) ;
#10254=CARTESIAN_POINT ( 'NONE',  ( -11.97929049433705373, 9.719999999999998863, 0.7046979865771783036 ) ) ;
#10267=CARTESIAN_POINT ( 'NONE',  ( -11.33523815116046229, 5.279172990141937305, 5.677742996778201601 ) ) ;
#10279=FACE_OUTER_BOUND ( 'NONE', #198975, .T. ) ;
#10292=CARTESIAN_POINT ( 'NONE',  ( 11.14442593998487219, 9.074645745019246590, -4.464617754680513251 ) ) ;
#10298=VECTOR ( 'NONE', #111373, 1000.000000000000000 ) ;
#10303=CARTESIAN_POINT ( 'NONE',  ( -11.89942855770814134, 13.79999999999999893, 0.6999999999999992895 ) ) ;
#10341=B_SPLINE_CURVE_WITH_KNOTS ( 'NONE', 3,
 ( #36646, #69128, #123342, #103804, #121197, #169853 ),
 .UNSPECIFIED., .F., .F.,
 ( 4, 2, 4 ),
 ( 0.000000000000000000, 0.0003767011250903910184, 0.0007534022501807820368 ),
 .UNSPECIFIED. ) ;
#10362=ORIENTED_EDGE ( 'NONE', *, *, #196360, .F. ) ;
#10371=VERTEX_POINT ( 'NONE', #20731 ) ;
#10376=ADVANCED_FACE ( 'NONE', ( #137727, #86826, #55391, #4468, #22863, #70540, #136659, #54333 ), #120472, .F. ) ;
#10378=CARTESIAN_POINT ( 'NONE',  ( -10.83925572545688176, 5.627432043407306850, 6.488667418600651438 ) ) ;
#10381=ORIENTED_EDGE ( 'NONE', *, *, #158942, .F. ) ;
#10383=CARTESIAN_POINT ( 'NONE',  ( 7.127657509075540965, 14.48195938056236898, 9.656923498056537269 ) ) ;
#10427=ADVANCED_FACE ( 'NONE', ( #60716 ), #3176, .F. ) ;
#10446=FACE_OUTER_BOUND ( 'NONE', #165738, .T. ) ;
#10452=CARTESIAN_POINT ( 'NONE',  ( -9.970593631352514308, 5.552127128363319564, -5.997086463700067149 ) ) ;
#10478=ADVANCED_FACE ( 'NONE', ( #95389 ), #96455, .F. ) ;
#10508=ORIENTED_EDGE ( 'NONE', *, *, #21226, .T. ) ;
#10518=CARTESIAN_POINT ( 'NONE',  ( 11.84668730067608600, 13.40000000000000036, -1.400000000000001910 ) ) ;
#10525=SURFACE_SIDE_STYLE ('',( #43070 ) ) ;
#10546=ADVANCED_FACE ( 'NONE', ( #50868 ), #173918, .T. ) ;
#10550=CARTESIAN_POINT ( 'NONE',  ( 9.976179289984715481, 9.863349661746255492, -6.608275209389087301 ) ) ;
#10553=CARTESIAN_POINT ( 'NONE',  ( -9.770225302207578011, 4.446947604919802011, 6.899101747692366615 ) ) ;
#10557=CARTESIAN_POINT ( 'NONE',  ( -9.380315451526849202, 14.53091799469200396, -7.483989755400268784 ) ) ;
#10570=CARTESIAN_POINT ( 'NONE',  ( -11.01135777277262129, 13.40000000000000036, -1.400000000000001910 ) ) ;
#10579=( NAMED_UNIT ( * ) SI_UNIT ( $, .STERADIAN. ) SOLID_ANGLE_UNIT ( ) );
#10634=CARTESIAN_POINT ( 'NONE',  ( 11.81907076198591966, 13.75731224596471769, 1.592066415281218505 ) ) ;
#10639=CARTESIAN_POINT ( 'NONE',  ( 11.48888942944796021, 8.940748223555385010, 3.094007481724269315 ) ) ;
#10684=CARTESIAN_POINT ( 'NONE',  ( 11.97181042169641962, 11.37999999999999901, -0.8318531151397201562 ) ) ;
#10685=FILL_AREA_STYLE ('',( #126670 ) ) ;
#10698=CARTESIAN_POINT ( 'NONE',  ( -4.779331034874314099, 14.55303417034376423, 10.96804219640860012 ) ) ;
#10700=TOROIDAL_SURFACE ( 'NONE', #211399, 11.92000000000000348, 0.08000000000000000167 ) ;
#10701=LINE ( 'NONE', #209958, #145088 ) ;
#10706=CIRCLE ( 'NONE', #183731, 0.5000000000000015543 ) ;
#10708=DIRECTION ( 'NONE',  ( 0.000000000000000000, 0.000000000000000000, -1.000000000000000000 ) ) ;
#10756=CARTESIAN_POINT ( 'NONE',  ( 11.22152876905117402, 8.821419385122529988, 4.110082514564867395 ) ) ;
#10777=CARTESIAN_POINT ( 'NONE',  ( 11.81900460097218186, 11.25757134874136334, 1.592493057836596115 ) ) ;
#10789=ORIENTED_EDGE ( 'NONE', *, *, #36106, .F. ) ;
#10794=DIRECTION ( 'NONE',  ( 0.000000000000000000, 1.000000000000000000, 0.000000000000000000 ) ) ;
#10835=CARTESIAN_POINT ( 'NONE',  ( -3.007788591379378040, 14.48002907089885483, 11.62584875609310231 ) ) ;
#10840=CARTESIAN_POINT ( 'NONE',  ( -11.86239285000045740, 11.37999999999998302, 1.812080536912751283 ) ) ;
#10868=CARTESIAN_POINT ( 'NONE',  ( 11.45846087878779329, 12.50688399218553748, -3.566076377698155664 ) ) ;
#10881=CARTESIAN_POINT ( 'NONE',  ( 1.500000000000035971, 7.750000000000000000, 10.64483442802187696 ) ) ;
#10922=CIRCLE ( 'NONE', #52517, 11.92000000000000171 ) ;
#10941=ORIENTED_EDGE ( 'NONE', *, *, #183326, .T. ) ;
#10952=( GEOMETRIC_REPRESENTATION_CONTEXT ( 3 ) GLOBAL_UNCERTAINTY_ASSIGNED_CONTEXT ( ( #17993 ) ) GLOBAL_UNIT_ASSIGNED_CONTEXT ( ( #71744, #172486, #58725 ) ) REPRESENTATION_CONTEXT ( 'NONE', 'WORKASPACE' ) );
#10954=CARTESIAN_POINT ( 'NONE',  ( -15.75000000000000000, 9.799999999999982947, 1.799999999999999600 ) ) ;
#10972=CARTESIAN_POINT ( 'NONE',  ( 8.790098660144264997, 13.29414747594432455, 8.101455065885630802 ) ) ;
#10982=ORIENTED_EDGE ( 'NONE', *, *, #205622, .T. ) ;
#10984=ORIENTED_EDGE ( 'NONE', *, *, #7050, .F. ) ;
#10999=CARTESIAN_POINT ( 'NONE',  ( 11.89844258446855818, 11.32852689329961215, -1.560502987793222163 ) ) ;
#11006=MECHANICAL_DESIGN_GEOMETRIC_PRESENTATION_REPRESENTATION('',(#121815),#118389);
#11012=CARTESIAN_POINT ( 'NONE',  ( -15.75000000000000000, 12.30000000000000071, 0.6999999999999992895 ) ) ;
#11033=CARTESIAN_POINT ( 'NONE',  ( 7.219650724572225897, 15.51887837940885895, 9.591874471555675186 ) ) ;
#11035=CARTESIAN_POINT ( 'NONE',  ( 1.499999999999961364, 8.500000000000000000, -10.64483442802188939 ) ) ;
#11041=CARTESIAN_POINT ( 'NONE',  ( 11.94655611907589154, 12.44799055453095527, 1.134828163062136852 ) ) ;
#11051=CARTESIAN_POINT ( 'NONE',  ( -3.796053574490474869, 15.00000000000207656, -12.24940615670125510 ) ) ;
#11080=B_SPLINE_CURVE_WITH_KNOTS ( 'NONE', 3,
 ( #11085, #24132, #188780, #76100, #205011, #158425, #106521, #208218, #57723, #206088, #91312, #155225 ),
 .UNSPECIFIED., .F., .F.,
 ( 4, 2, 2, 2, 2, 4 ),
 ( -5.999999997212162571E-08, 0.0007498576660960367670, 0.001124816499144041257, 0.001499775332192045639, 0.002249692998288053102, 0.002999610664384060564 ),
 .UNSPECIFIED. ) ;
#11085=CARTESIAN_POINT ( 'NONE',  ( -10.84254087577847869, 4.919568073182958301, 5.035408296252059657 ) ) ;
#11102=CARTESIAN_POINT ( 'NONE',  ( -3.111427816635929045, 14.48006665644674484, -11.59831529056025801 ) ) ;
#11148=CARTESIAN_POINT ( 'NONE',  ( -11.94105722165067363, 12.57417237917041142, 1.187919369849792295 ) ) ;
#11166=( NAMED_UNIT ( * ) SI_UNIT ( $, .STERADIAN. ) SOLID_ANGLE_UNIT ( ) );
#11170=CARTESIAN_POINT ( 'NONE',  ( 11.80937116653883123, 7.958520514542954949, 2.169913335582353664 ) ) ;
#11171=ORIENTED_EDGE ( 'NONE', *, *, #206662, .F. ) ;
#11176=DIRECTION ( 'NONE',  ( -0.1510067114093955887, 0.000000000000000000, -0.9885327375000383388 ) ) ;
#11179=LINE ( 'NONE', #188872, #139754 ) ;
#11189=CARTESIAN_POINT ( 'NONE',  ( 11.38909496574627056, 7.479950087089620503, -5.016624281428613941 ) ) ;
#11194=ORIENTED_EDGE ( 'NONE', *, *, #152817, .T. ) ;
#11196=VERTEX_POINT ( 'NONE', #86565 ) ;
#11204=DIRECTION ( 'NONE',  ( 1.000000000000000000, -0.000000000000000000, -0.000000000000000000 ) ) ;
#11240=EDGE_CURVE ( 'NONE', #33454, #1299, #188318, .T. ) ;
#11251=CARTESIAN_POINT ( 'NONE',  ( -11.44789321844504215, 13.79999999999998295, 3.303298730975396946 ) ) ;
#11279=CARTESIAN_POINT ( 'NONE',  ( -15.75000000000000000, 13.39999999999998259, 3.599999999999999201 ) ) ;
#11296=CARTESIAN_POINT ( 'NONE',  ( 6.742108083425078391, 15.99925261518604636, 9.534780690565009209 ) ) ;
#11323=CIRCLE ( 'NONE', #59729, 12.00000000000000178 ) ;
#11330=CARTESIAN_POINT ( 'NONE',  ( -11.83627402213341107, 4.942735150756283780, -4.855302456647772935 ) ) ;
#11353=CARTESIAN_POINT ( 'NONE',  ( 11.97020876039858628, 7.690570200886937435, -0.8734403169683351287 ) ) ;
#11376=EDGE_CURVE ( 'NONE', #2318, #33454, #142846, .T. ) ;
#11416=CARTESIAN_POINT ( 'NONE',  ( -11.08262820474602250, 7.067544101916862331, -4.606611893229879406 ) ) ;
#11435=PRESENTATION_STYLE_ASSIGNMENT (( #26625 ) ) ;
#11447=CARTESIAN_POINT ( 'NONE',  ( -10.44369633504468631, 5.112959841837462882, -5.232137017608344820 ) ) ;
#11453=SURFACE_SIDE_STYLE ('',( #147877 ) ) ;
#11456=ORIENTED_EDGE ( 'NONE', *, *, #48444, .T. ) ;
#11463=ORIENTED_EDGE ( 'NONE', *, *, #107473, .F. ) ;
#11474=AXIS2_PLACEMENT_3D ( 'NONE', #84087, #150175, #1743 ) ;
#11477=VERTEX_POINT ( 'NONE', #175296 ) ;
#11479=FACE_OUTER_BOUND ( 'NONE', #135491, .T. ) ;
#11492=DIRECTION ( 'NONE',  ( 0.000000000000000000, 0.000000000000000000, -1.000000000000000000 ) ) ;
#11502=VERTEX_POINT ( 'NONE', #191508 ) ;
#11508=CARTESIAN_POINT ( 'NONE',  ( 0.000000000000000000, 9.799999999999982947, 0.000000000000000000 ) ) ;
#11519=DIRECTION ( 'NONE',  ( 0.000000000000000000, 0.000000000000000000, -1.000000000000000000 ) ) ;
#11524=CARTESIAN_POINT ( 'NONE',  ( -11.38600250725030172, 3.712543481068769857, -5.706073308245968256 ) ) ;
#11529=EDGE_LOOP ( 'NONE', ( #127053, #177665, #111076, #68710 ) ) ;
#11541=ORIENTED_EDGE ( 'NONE', *, *, #81633, .F. ) ;
#11599=VERTEX_POINT ( 'NONE', #162232 ) ;
#11601=CARTESIAN_POINT ( 'NONE',  ( 11.92619525870748021, 10.07377703206318031, 1.328859154005125554 ) ) ;
#11618=CARTESIAN_POINT ( 'NONE',  ( 11.35396574786309998, 7.538279440392132713, 3.751616533526511699 ) ) ;
#11622=FILL_AREA_STYLE_COLOUR ( '', #100701 ) ;
#11650=CARTESIAN_POINT ( 'NONE',  ( 11.41381676900476805, 10.06958039977608088, 3.704697931490188889 ) ) ;
#11661=CARTESIAN_POINT ( 'NONE',  ( 8.386878554176760758, 15.11743023405602848, -8.584041405059041452 ) ) ;
#11689=MECHANICAL_DESIGN_GEOMETRIC_PRESENTATION_REPRESENTATION('',(#60243),#42963);
#11712=CARTESIAN_POINT ( 'NONE',  ( 9.962237412473150755, 12.35880645891234408, 7.801823201411741238 ) ) ;
#11766=CARTESIAN_POINT ( 'NONE',  ( -5.972841284750454172, 14.55272318667275933, 10.36653721697756936 ) ) ;
#11773=FILL_AREA_STYLE ('',( #124564 ) ) ;
#11814=CARTESIAN_POINT ( 'NONE',  ( 0.000000000000000000, 4.000007913748540922, 1.105031132475055157E-32 ) ) ;
#11820=EDGE_LOOP ( 'NONE', ( #18910, #197386, #111993, #73215 ) ) ;
#11823=SURFACE_SIDE_STYLE ('',( #142948 ) ) ;
#11829=( GEOMETRIC_REPRESENTATION_CONTEXT ( 3 ) GLOBAL_UNCERTAINTY_ASSIGNED_CONTEXT ( ( #204976 ) ) GLOBAL_UNIT_ASSIGNED_CONTEXT ( ( #111538, #61654, #146131 ) ) REPRESENTATION_CONTEXT ( 'NONE', 'WORKASPACE' ) );
#11859=CARTESIAN_POINT ( 'NONE',  ( -10.19097401674926395, 4.476076320095182304, 5.708917106338025960 ) ) ;
#11874=ORIENTED_EDGE ( 'NONE', *, *, #110186, .F. ) ;
#11905=TOROIDAL_SURFACE ( 'NONE', #129666, 11.92000000000000171, 0.08000000000000000167 ) ;
#11908=EDGE_CURVE ( 'NONE', #48473, #131174, #111815, .T. ) ;
#11948=DIRECTION ( 'NONE',  ( 0.000000000000000000, 0.000000000000000000, 1.000000000000000000 ) ) ;
#11957=ORIENTED_EDGE ( 'NONE', *, *, #98123, .F. ) ;
#11958=DIRECTION ( 'NONE',  ( 0.000000000000000000, 0.000000000000000000, 1.000000000000000000 ) ) ;
#11962=PRESENTATION_STYLE_ASSIGNMENT (( #160359 ) ) ;
#11964=DIRECTION ( 'NONE',  ( -0.05872483221476467591, 7.952201780260630618E-17, -0.9982742078614211811 ) ) ;
#12015=MECHANICAL_DESIGN_GEOMETRIC_PRESENTATION_REPRESENTATION('',(#98457),#133123);
#12043=EDGE_CURVE ( 'NONE', #35130, #84148, #193256, .T. ) ;
#12046=PRESENTATION_STYLE_ASSIGNMENT (( #124826 ) ) ;
#12057=CARTESIAN_POINT ( 'NONE',  ( -15.75000000000000000, 12.29999999999998295, 3.199999999999997957 ) ) ;
#12097=CARTESIAN_POINT ( 'NONE',  ( -15.75000000000000000, 11.29999999999999893, -0.7000000000000009548 ) ) ;
#12126=CARTESIAN_POINT ( 'NONE',  ( -1.878313713276733132, 14.99999999999692157, -12.68000002627077905 ) ) ;
#12139=EDGE_LOOP ( 'NONE', ( #143365, #194864, #17986, #174081, #45867, #151216, #71902, #109574 ) ) ;
#12155=ORIENTED_EDGE ( 'NONE', *, *, #31143, .T. ) ;
#12187=CIRCLE ( 'NONE', #39884, 0.5000000000000013323 ) ;
#12213=ORIENTED_EDGE ( 'NONE', *, *, #178173, .T. ) ;
#12237=DIRECTION ( 'NONE',  ( 0.3162277660168373861, -0.9486832980505139901, 0.000000000000000000 ) ) ;
#12240=CARTESIAN_POINT ( 'NONE',  ( 11.99957350801783562, 7.640677523568208507, 0.4513943822151063046 ) ) ;
#12248=FILL_AREA_STYLE_COLOUR ( '', #108722 ) ;
#12259=CARTESIAN_POINT ( 'NONE',  ( 9.742269887272128059, 13.15996534559037912, -8.088430353861673083 ) ) ;
#12269=ADVANCED_FACE ( 'NONE', ( #56857 ), #158705, .F. ) ;
#12290=EDGE_CURVE ( 'NONE', #7674, #49203, #193677, .T. ) ;
#12313=CARTESIAN_POINT ( 'NONE',  ( -7.247736482493067456, 14.00000000000182254, 10.57961706324693019 ) ) ;
#12334=CARTESIAN_POINT ( 'NONE',  ( 11.78331023100045627, 11.29999999999998117, 1.799999999999999600 ) ) ;
#12342=PLANE ( 'NONE',  #213339 ) ;
#12352=AXIS2_PLACEMENT_3D ( 'NONE', #49112, #199592, #181222 ) ;
#12358=CARTESIAN_POINT ( 'NONE',  ( 8.724581073908543871, 13.71543862355972188, -7.774732811725550974 ) ) ;
#12361=CARTESIAN_POINT ( 'NONE',  ( 7.210140354588870260, 13.96302891847841998, 9.188013455993196743 ) ) ;
#12394=CARTESIAN_POINT ( 'NONE',  ( -11.83256397649420677, 7.177290438377375459, -1.867481893931521419 ) ) ;
#12412=CARTESIAN_POINT ( 'NONE',  ( -9.568394635444461116, 15.10427918654218082, 7.242253469826407830 ) ) ;
#12419=CARTESIAN_POINT ( 'NONE',  ( 11.96976056191701154, 7.637744957010472291, -0.8800080678311683613 ) ) ;
#12428=DIRECTION ( 'NONE',  ( -0.000000000000000000, 1.000000000000000000, -0.000000000000000000 ) ) ;
#12435=EDGE_CURVE ( 'NONE', #7968, #210693, #178891, .T. ) ;
#12473=CARTESIAN_POINT ( 'NONE',  ( -11.32659722783424705, 6.354439326305993951, -3.967491859357531236 ) ) ;
#12482=CARTESIAN_POINT ( 'NONE',  ( -11.90622689666433942, 8.910945625224377054, -1.226100016398791404 ) ) ;
#12485=CARTESIAN_POINT ( 'NONE',  ( -15.75000000000000000, 13.40000000000000036, -3.200000000000001510 ) ) ;
#12489=EDGE_LOOP ( 'NONE', ( #157261, #153499, #210964, #130672 ) ) ;
#12500=( GEOMETRIC_REPRESENTATION_CONTEXT ( 3 ) GLOBAL_UNCERTAINTY_ASSIGNED_CONTEXT ( ( #135990 ) ) GLOBAL_UNIT_ASSIGNED_CONTEXT ( ( #89847, #188378, #6415 ) ) REPRESENTATION_CONTEXT ( 'NONE', 'WORKASPACE' ) );
#12514=CARTESIAN_POINT ( 'NONE',  ( -11.36817070414822695, 5.406007704794011381, -5.610921796774237968 ) ) ;
#12550=CARTESIAN_POINT ( 'NONE',  ( 9.452508394161716510, 3.481540833006149249, 7.393820799723206605 ) ) ;
#12566=( GEOMETRIC_REPRESENTATION_CONTEXT ( 3 ) GLOBAL_UNCERTAINTY_ASSIGNED_CONTEXT ( ( #66671 ) ) GLOBAL_UNIT_ASSIGNED_CONTEXT ( ( #76426, #142535, #177137 ) ) REPRESENTATION_CONTEXT ( 'NONE', 'WORKASPACE' ) );
#12581=CARTESIAN_POINT ( 'NONE',  ( -10.22593938286385296, 3.000029897349846930, -7.498676971688964521 ) ) ;
#12589=( LENGTH_UNIT ( ) NAMED_UNIT ( * ) SI_UNIT ( .MILLI., .METRE. ) );
#12594=MECHANICAL_DESIGN_GEOMETRIC_PRESENTATION_REPRESENTATION('',(#50633),#74777);
#12598=TOROIDAL_SURFACE ( 'NONE', #29942, 11.92000000000000171, 0.08000000000000000167 ) ;
#12623=UNCERTAINTY_MEASURE_WITH_UNIT (LENGTH_MEASURE( 1.000000000000000082E-05 ), #103543, 'distance_accuracy_value', 'NONE');
#12638=TOROIDAL_SURFACE ( 'NONE', #164794, 11.91999999999999993, 0.08000000000000000167 ) ;
#12661=ADVANCED_FACE ( 'NONE', ( #161591 ), #96601, .T. ) ;
#12675=DIRECTION ( 'NONE',  ( 0.000000000000000000, -1.000000000000000000, -9.023263958591317418E-17 ) ) ;
#12680=SURFACE_STYLE_FILL_AREA ( #143817 ) ;
#12684=FILL_AREA_STYLE_COLOUR ( '', #72343 ) ;
#12695=CARTESIAN_POINT ( 'NONE',  ( -0.0004021858452125243177, 15.43212108951242634, 11.92774328084775171 ) ) ;
#12713=( BOUNDED_SURFACE ( )  B_SPLINE_SURFACE ( 3, 2, ( 
 ( #74486, #192479, #193561 ),
 ( #91827, #157886, #11601 ),
 ( #110252, #207672, #144859 ),
 ( #191411, #143795, #30006 ),
 ( #158936, #93959, #58232 ),
 ( #45204, #140592, #111318 ) ),
 .UNSPECIFIED., .F., .F., .T. ) 
 B_SPLINE_SURFACE_WITH_KNOTS ( ( 4, 2, 4 ),
 ( 3, 3 ),
 ( 0.000000000000000000, 0.0003766365702389427254, 0.0007532731404778854507 ),
 ( 0.000000000000000000, 1.000000000000000000 ),
 .UNSPECIFIED. ) 
 GEOMETRIC_REPRESENTATION_ITEM ( )  RATIONAL_B_SPLINE_SURFACE ( (
 ( 1.000000000000000000, 0.7452309222762957264, 1.000000000000000000),
 ( 1.000000000000000000, 0.7451892422671834160, 1.000000000000000000),
 ( 1.000000000000000000, 0.7429606254238495522, 1.000000000000000000),
 ( 1.000000000000000000, 0.7311462761265991039, 1.000000000000000000),
 ( 1.000000000000000000, 0.7212257702791121661, 1.000000000000000000),
 ( 1.000000000000000000, 0.7071067811865475727, 1.000000000000000000) ) ) 
 REPRESENTATION_ITEM ( '' )  SURFACE ( )  );
#12716=CARTESIAN_POINT ( 'NONE',  ( 0.000000000000000000, 11.29999999999999893, 0.000000000000000000 ) ) ;
#12735=ORIENTED_EDGE ( 'NONE', *, *, #136253, .F. ) ;
#12743=CARTESIAN_POINT ( 'NONE',  ( 9.681420934716557625, 3.864711529694057290, 7.090140244710065431 ) ) ;
#12766=CARTESIAN_POINT ( 'NONE',  ( 10.74631150800302670, 10.90885146202907663, -5.675916053542507278 ) ) ;
#12777=VERTEX_POINT ( 'NONE', #30520 ) ;
#12778=VECTOR ( 'NONE', #53984, 1000.000000000000000 ) ;
#12791=CARTESIAN_POINT ( 'NONE',  ( -11.88168509644349058, 11.37999999999999901, -1.685788023084331400 ) ) ;
#12821=( NAMED_UNIT ( * ) SI_UNIT ( $, .STERADIAN. ) SOLID_ANGLE_UNIT ( ) );
#12829=EDGE_CURVE ( 'NONE', #201145, #201330, #197257, .T. ) ;
#12835=EDGE_CURVE ( 'NONE', #102037, #84082, #179943, .T. ) ;
#12871=CARTESIAN_POINT ( 'NONE',  ( -11.86145016429273014, 10.19999999999999929, 1.099999999999996980 ) ) ;
#12909=FILL_AREA_STYLE ('',( #59539 ) ) ;
#12919=CARTESIAN_POINT ( 'NONE',  ( -10.90754186426655004, 4.636108433425621733, 4.485516275142084730 ) ) ;
#12933=EDGE_CURVE ( 'NONE', #157191, #187611, #14224, .T. ) ;
#12948=ORIENTED_EDGE ( 'NONE', *, *, #136122, .F. ) ;
#12978=CARTESIAN_POINT ( 'NONE',  ( -11.89844258446855285, 11.32852689329959439, 1.560502987793273233 ) ) ;
#12981=CARTESIAN_POINT ( 'NONE',  ( -10.98550897202509269, 11.25719568827052974, -1.591908179352835351 ) ) ;
#13004=CARTESIAN_POINT ( 'NONE',  ( 11.48243876534946217, 12.30000000000000071, -3.200000000000001510 ) ) ;
#13045=VECTOR ( 'NONE', #20795, 1000.000000000000000 ) ;
#13056=CARTESIAN_POINT ( 'NONE',  ( -11.04536101718726293, 10.90000000000000036, 1.099999999999996758 ) ) ;
#13067=PLANE ( 'NONE',  #136646 ) ;
#13115=ORIENTED_EDGE ( 'NONE', *, *, #35015, .T. ) ;
#13142=CARTESIAN_POINT ( 'NONE',  ( -11.44779965693287416, 12.60313923201275799, 3.599999932275866676 ) ) ;
#13177=UNCERTAINTY_MEASURE_WITH_UNIT (LENGTH_MEASURE( 1.000000000000000082E-05 ), #106243, 'distance_accuracy_value', 'NONE');
#13180=CARTESIAN_POINT ( 'NONE',  ( -11.84668730067608600, 13.39999999999998259, 1.399999999999998579 ) ) ;
#13181=EDGE_CURVE ( 'NONE', #159273, #176022, #202247, .T. ) ;
#13186=CARTESIAN_POINT ( 'NONE',  ( 11.97181042169640897, 12.22000000000000064, 0.8318531151397160484 ) ) ;
#13196=EDGE_LOOP ( 'NONE', ( #154646, #111216, #105783, #111891 ) ) ;
#13207=VECTOR ( 'NONE', #45628, 1000.000000000000000 ) ;
#13244=ORIENTED_EDGE ( 'NONE', *, *, #120497, .F. ) ;
#13282=EDGE_LOOP ( 'NONE', ( #34437, #147889, #139099, #39048 ) ) ;
#13289=VERTEX_POINT ( 'NONE', #185859 ) ;
#13304=DIRECTION ( 'NONE',  ( 0.000000000000000000, 0.000000000000000000, 1.000000000000000000 ) ) ;
#13306=DIRECTION ( 'NONE',  ( 0.000000000000000000, -1.000000000000000000, 0.000000000000000000 ) ) ;
#13313=CARTESIAN_POINT ( 'NONE',  ( 0.000000000000000000, 9.719999999999998863, 0.000000000000000000 ) ) ;
#13335=CARTESIAN_POINT ( 'NONE',  ( 9.263363473337784981, 13.05588735459848948, -8.991178861817273216 ) ) ;
#13357=CARTESIAN_POINT ( 'NONE',  ( 11.41176686791169104, 11.25950803486853502, -3.404018756831829418 ) ) ;
#13361=EDGE_CURVE ( 'NONE', #178392, #132967, #145557, .T. ) ;
#13364=CARTESIAN_POINT ( 'NONE',  ( -11.94105722165071093, 11.02582762082958467, -1.187919369849417484 ) ) ;
#13386=CARTESIAN_POINT ( 'NONE',  ( -11.07629303812015564, 5.828651784584821804, 4.512940454653985967 ) ) ;
#13389=CARTESIAN_POINT ( 'NONE',  ( -9.898321827460007327, 14.00000000000624034, 7.924999999990797406 ) ) ;
#13429=CARTESIAN_POINT ( 'NONE',  ( -10.62763048033980517, 4.753116220844278317, -5.576244429778776102 ) ) ;
#13433=CARTESIAN_POINT ( 'NONE',  ( 9.483953901554681210, 14.00935217397140953, -8.399901643884886582 ) ) ;
#13436=CARTESIAN_POINT ( 'NONE',  ( 6.744795205365000434, 13.99925803066161478, 9.538580854856197888 ) ) ;
#13468=CARTESIAN_POINT ( 'NONE',  ( -10.52284959769361805, 5.420271152154175986, 5.071911021504272199 ) ) ;
#13494=CARTESIAN_POINT ( 'NONE',  ( 11.34491280883428033, 8.770310257811074095, 3.915374332514163669 ) ) ;
#13508=MECHANICAL_DESIGN_GEOMETRIC_PRESENTATION_REPRESENTATION('',(#106962),#37630);
#13509=CARTESIAN_POINT ( 'NONE',  ( 11.78331023100045627, 9.799999999999998934, -1.800000000000001155 ) ) ;
#13546=CARTESIAN_POINT ( 'NONE',  ( -11.51196935752114392, 6.864815107568656316, 3.393625645527715395 ) ) ;
#13554=CIRCLE ( 'NONE', #6727, 12.00000000000000178 ) ;
#13555=CARTESIAN_POINT ( 'NONE',  ( -10.81298704238391650, 6.434023936693727741, -5.221020569155840008 ) ) ;
#13585=CARTESIAN_POINT ( 'NONE',  ( -12.26673246283585961, 6.254089313302478637, -3.851195297204758727 ) ) ;
#13588=PLANE ( 'NONE',  #42477 ) ;
#13603=CARTESIAN_POINT ( 'NONE',  ( -11.91292854676714974, 12.48518470326975205, 1.446370920797324100 ) ) ;
#13647=CARTESIAN_POINT ( 'NONE',  ( 0.002914018882855369096, 14.55305236535103397, 11.95586205439599681 ) ) ;
#13661=SURFACE_STYLE_USAGE ( .BOTH. , #213963 ) ;
#13668=ORIENTED_EDGE ( 'NONE', *, *, #212293, .T. ) ;
#13672=DIRECTION ( 'NONE',  ( 0.000000000000000000, 0.000000000000000000, -1.000000000000000000 ) ) ;
#13691=FACE_OUTER_BOUND ( 'NONE', #188013, .T. ) ;
#13720=COLOUR_RGB ( '', 0.09019608, 0.27058824, 0.51372549) ;
#13749=EDGE_CURVE ( 'NONE', #193462, #180190, #138050, .T. ) ;
#13750=CARTESIAN_POINT ( 'NONE',  ( 11.65646892497034592, 7.079448886673395336, -2.644575417635384618 ) ) ;
#13809=EDGE_CURVE ( 'NONE', #101924, #127020, #210704, .T. ) ;
#13814=CARTESIAN_POINT ( 'NONE',  ( -10.44369633504468631, 5.112959841837462882, -5.232137017608346596 ) ) ;
#13835=CARTESIAN_POINT ( 'NONE',  ( 11.15656239214823664, 9.703780284206802165, -5.826040129427457970 ) ) ;
#13852=CARTESIAN_POINT ( 'NONE',  ( 0.06005724485651787320, 14.50193764430533250, 11.99783616005606035 ) ) ;
#13860=DIRECTION ( 'NONE',  ( 0.05872483221476459958, 0.000000000000000000, -0.9982742078614211811 ) ) ;
#13866=CARTESIAN_POINT ( 'NONE',  ( -9.348561386899502779, 3.999985931113709814, -7.001914024221965960 ) ) ;
#13890=SURFACE_STYLE_USAGE ( .BOTH. , #17085 ) ;
#13900=CIRCLE ( 'NONE', #93578, 0.07999999999999998779 ) ;
#13918=EDGE_CURVE ( 'NONE', #11196, #202127, #26572, .T. ) ;
#13959=DIRECTION ( 'NONE',  ( -0.000000000000000000, -1.000000000000000000, -0.000000000000000000 ) ) ;
#13971=CARTESIAN_POINT ( 'NONE',  ( -9.586151930903435314, 14.76609868405410886, 7.218760141420751175 ) ) ;
#13985=ORIENTED_EDGE ( 'NONE', *, *, #66840, .T. ) ;
#14021=EDGE_CURVE ( 'NONE', #7711, #43590, #84924, .T. ) ;
#14036=CARTESIAN_POINT ( 'NONE',  ( 8.717236016799597920, 13.50218641590694979, 8.247095274259196529 ) ) ;
#14076=CARTESIAN_POINT ( 'NONE',  ( -15.75000000000000000, 11.29999999999998117, 3.199999999999997957 ) ) ;
#14090=DIRECTION ( 'NONE',  ( 1.000000000000000000, -0.000000000000000000, -0.000000000000000000 ) ) ;
#14120=DIRECTION ( 'NONE',  ( 0.000000000000000000, 1.000000000000000000, 0.000000000000000000 ) ) ;
#14122=FILL_AREA_STYLE_COLOUR ( '', #105569 ) ;
#14127=EDGE_CURVE ( 'NONE', #29424, #162756, #75728, .T. ) ;
#14130=EDGE_LOOP ( 'NONE', ( #27426, #159998, #185496, #114749 ) ) ;
#14138=FACE_BOUND ( 'NONE', #86725, .T. ) ;
#14162=ORIENTED_EDGE ( 'NONE', *, *, #124080, .T. ) ;
#14199=ORIENTED_EDGE ( 'NONE', *, *, #74843, .F. ) ;
#14208=CARTESIAN_POINT ( 'NONE',  ( 11.84668730067608600, 10.89999999999998259, 1.399999999999998579 ) ) ;
#14213=VERTEX_POINT ( 'NONE', #25255 ) ;
#14224=LINE ( 'NONE', #11035, #58873 ) ;
#14225=CARTESIAN_POINT ( 'NONE',  ( 11.86687934130374522, 12.49048050383441755, 1.056332641424306606 ) ) ;
#14234=ORIENTED_EDGE ( 'NONE', *, *, #173298, .F. ) ;
#14236=UNCERTAINTY_MEASURE_WITH_UNIT (LENGTH_MEASURE( 1.000000000000000082E-05 ), #133148, 'distance_accuracy_value', 'NONE');
#14287=VERTEX_POINT ( 'NONE', #202920 ) ;
#14294=CARTESIAN_POINT ( 'NONE',  ( 11.33772463945043718, 10.90000000000000924, -3.600000000000078693 ) ) ;
#14313=DIRECTION ( 'NONE',  ( 0.000000000000000000, 0.000000000000000000, 1.000000000000000000 ) ) ;
#14322=ADVANCED_FACE ( 'NONE', ( #46875 ), #115733, .T. ) ;
#14359=CARTESIAN_POINT ( 'NONE',  ( 0.000000000000000000, 12.21999999999998288, 0.000000000000000000 ) ) ;
#14365=DIRECTION ( 'NONE',  ( 0.000000000000000000, 1.804652791718263484E-16, -1.000000000000000000 ) ) ;
#14368=CARTESIAN_POINT ( 'NONE',  ( -11.91826849282518452, 10.19999999999999929, -1.400000000000001465 ) ) ;
#14385=ADVANCED_FACE ( 'NONE', ( #190 ), #3034, .T. ) ;
#14386=CARTESIAN_POINT ( 'NONE',  ( 10.16691492120896712, 10.85832867828739090, -8.127724911529011109 ) ) ;
#14390=VERTEX_POINT ( 'NONE', #1266 ) ;
#14392=EDGE_LOOP ( 'NONE', ( #110334, #150269, #110375, #15961 ) ) ;
#14403=DIRECTION ( 'NONE',  ( 1.000000000000000000, -0.000000000000000000, -0.000000000000000000 ) ) ;
#14408=STYLED_ITEM ( 'NONE', ( #71261 ), #60652 ) ;
#14417=CARTESIAN_POINT ( 'NONE',  ( -11.94105721237523099, 10.90000000000000036, -1.187919463087248939 ) ) ;
#14439=CARTESIAN_POINT ( 'NONE',  ( -11.26783843162779775, 6.407685724923858572, -3.998516562640498151 ) ) ;
#14440=EDGE_CURVE ( 'NONE', #124, #4829, #2327, .T. ) ;
#14443=CARTESIAN_POINT ( 'NONE',  ( -11.41176686791169281, 13.75950803486851903, 3.404018756831824533 ) ) ;
#14448=CARTESIAN_POINT ( 'NONE',  ( 0.000000000000000000, 19.00000000000000000, 11.18000000000000149 ) ) ;
#14467=EDGE_CURVE ( 'NONE', #14213, #19175, #37703, .T. ) ;
#14472=DIRECTION ( 'NONE',  ( 1.000000000000000000, 0.000000000000000000, -0.000000000000000000 ) ) ;
#14484=CARTESIAN_POINT ( 'NONE',  ( -10.08983450696851669, 4.085200418580138049, 6.506611369081194418 ) ) ;
#14488=CARTESIAN_POINT ( 'NONE',  ( 8.498552245539556793, 15.83935224703753875, -9.434290412321708175 ) ) ;
#14491=CARTESIAN_POINT ( 'NONE',  ( 6.861935260488042587, 14.99925532292382790, 9.452900204311735166 ) ) ;
#14497=EDGE_LOOP ( 'NONE', ( #167537, #79639, #140741, #60778 ) ) ;
#14523=CARTESIAN_POINT ( 'NONE',  ( -11.14389002924298566, 7.220603907090449525, 3.549113525960188031 ) ) ;
#14535=FACE_OUTER_BOUND ( 'NONE', #29609, .T. ) ;
#14541=FACE_OUTER_BOUND ( 'NONE', #49899, .T. ) ;
#14547=EDGE_LOOP ( 'NONE', ( #51688, #164098, #18057, #7513 ) ) ;
#14550=CARTESIAN_POINT ( 'NONE',  ( 11.63317533773959589, 8.260435399328212469, -2.973782887496474459 ) ) ;
#14563=VECTOR ( 'NONE', #191994, 1000.000000000000000 ) ;
#14588=CARTESIAN_POINT ( 'NONE',  ( 0.000000000000000000, 14.55305236562704252, -11.95586206896551928 ) ) ;
#14600=CARTESIAN_POINT ( 'NONE',  ( -12.00016184804641206, 8.029277273509505264, -0.2582136249091951385 ) ) ;
#14627=VECTOR ( 'NONE', #139931, 1000.000000000000000 ) ;
#14640=CARTESIAN_POINT ( 'NONE',  ( -11.77619280525687451, 4.711391180887883223, -4.977117663154129623 ) ) ;
#14645=FILL_AREA_STYLE ('',( #93809 ) ) ;
#14648=ORIENTED_EDGE ( 'NONE', *, *, #139829, .T. ) ;
#14658=AXIS2_PLACEMENT_3D ( 'NONE', #188451, #101875, #19543 ) ;
#14661=CARTESIAN_POINT ( 'NONE',  ( -11.92050416151433012, 12.44794624720363174, 1.381922468431395767 ) ) ;
#14680=CARTESIAN_POINT ( 'NONE',  ( 9.333041836227126353, 3.553052365627043852, 7.472413793103449997 ) ) ;
#14697=EDGE_CURVE ( 'NONE', #36899, #132416, #45546, .T. ) ;
#14732=FACE_OUTER_BOUND ( 'NONE', #188611, .T. ) ;
#14754=UNCERTAINTY_MEASURE_WITH_UNIT (LENGTH_MEASURE( 1.000000000000000082E-05 ), #46865, 'distance_accuracy_value', 'NONE');
#14755=CARTESIAN_POINT ( 'NONE',  ( 11.04536101718726293, 11.00581808788928306, 1.099999999999996980 ) ) ;
#14798=CIRCLE ( 'NONE', #87489, 0.08000000000000015432 ) ;
#14810=VECTOR ( 'NONE', #46946, 1000.000000000000000 ) ;
#14812=CARTESIAN_POINT ( 'NONE',  ( 10.59765138761703085, 12.29999999999998472, 3.303242380465396533 ) ) ;
#14845=CARTESIAN_POINT ( 'NONE',  ( 8.230276427067300560, 15.16059583899921037, -8.673450386635328968 ) ) ;
#14860=CIRCLE ( 'NONE', #139531, 12.00000000000000178 ) ;
#14883=CARTESIAN_POINT ( 'NONE',  ( 9.449756383040847751, 11.01506308870569306, -7.402102152998049078 ) ) ;
#14892=CARTESIAN_POINT ( 'NONE',  ( 9.686381629184177555, 13.40773330361598248, 8.159561931930056744 ) ) ;
#14893=MECHANICAL_DESIGN_GEOMETRIC_PRESENTATION_REPRESENTATION('',(#59920),#63328);
#14896=VERTEX_POINT ( 'NONE', #28209 ) ;
#14903=CARTESIAN_POINT ( 'NONE',  ( 8.634934822016738565, 13.76316009741527679, -8.269602696052166024 ) ) ;
#14927=ORIENTED_EDGE ( 'NONE', *, *, #212414, .T. ) ;
#14934=SURFACE_STYLE_FILL_AREA ( #81030 ) ;
#14949=( NAMED_UNIT ( * ) SI_UNIT ( $, .STERADIAN. ) SOLID_ANGLE_UNIT ( ) );
#14967=ORIENTED_EDGE ( 'NONE', *, *, #198798, .F. ) ;
#14998=( BOUNDED_SURFACE ( )  B_SPLINE_SURFACE ( 3, 2, ( 
 ( #101774, #167842, #85519 ),
 ( #135362, #201377, #117023 ),
 ( #180891, #53018, #32513 ),
 ( #149463, #1046, #16234 ),
 ( #166782, #183019, #102845 ),
 ( #168902, #18377, #70309 ) ),
 .UNSPECIFIED., .F., .F., .F. ) 
 B_SPLINE_SURFACE_WITH_KNOTS ( ( 4, 2, 4 ),
 ( 3, 3 ),
 ( 0.000000000000000000, 0.0003831416164015014384, 0.0007662832328030028768 ),
 ( 0.000000000000000000, 1.000000000000000000 ),
 .UNSPECIFIED. ) 
 GEOMETRIC_REPRESENTATION_ITEM ( )  RATIONAL_B_SPLINE_SURFACE ( (
 ( 1.000000000000000000, 0.7071067811865475727, 1.000000000000000000),
 ( 1.000000000000000000, 0.6829713513656784363, 1.000000000000000000),
 ( 1.000000000000000000, 0.6534833722367711095, 1.000000000000000000),
 ( 1.000000000000000000, 0.6054027484667287018, 1.000000000000000000),
 ( 1.000000000000000000, 0.5875453974411402047, 1.000000000000000000),
 ( 1.000000000000000000, 0.5879095031487528988, 1.000000000000000000) ) ) 
 REPRESENTATION_ITEM ( '' )  SURFACE ( )  );
#15000=STYLED_ITEM ( 'NONE', ( #143462 ), #66312 ) ;
#15039=CARTESIAN_POINT ( 'NONE',  ( 0.000000000000000000, 8.500000000000000000, 0.000000000000000000 ) ) ;
#15049=FILL_AREA_STYLE ('',( #165590 ) ) ;
#15050=ORIENTED_EDGE ( 'NONE', *, *, #188144, .F. ) ;
#15108=CARTESIAN_POINT ( 'NONE',  ( 8.727830756187987760, 13.53690963525370883, 8.169218635041765708 ) ) ;
#15130=CARTESIAN_POINT ( 'NONE',  ( 11.89839339040395139, 11.32877468403908772, 1.560885614203548100 ) ) ;
#15164=FACE_OUTER_BOUND ( 'NONE', #178813, .T. ) ;
#15178=CYLINDRICAL_SURFACE ( 'NONE', #111247, 0.3999999999999997446 ) ;
#15243=CARTESIAN_POINT ( 'NONE',  ( -10.29842937900060207, 4.863661338910580945, -6.166703023499271019 ) ) ;
#15261=CARTESIAN_POINT ( 'NONE',  ( 11.88172094500853504, 11.37999994398405867, -1.685553348215862446 ) ) ;
#15264=CARTESIAN_POINT ( 'NONE',  ( -11.94980361723156470, 13.50238056585419777, -1.099999926404080064 ) ) ;
#15275=FACE_OUTER_BOUND ( 'NONE', #123458, .T. ) ;
#15276=SURFACE_STYLE_USAGE ( .BOTH. , #48872 ) ;
#15307=CARTESIAN_POINT ( 'NONE',  ( 10.95308175811721085, 11.29999999999999893, -1.800000000000001155 ) ) ;
#15363=CARTESIAN_POINT ( 'NONE',  ( -11.86145016429273191, 13.50587876334730453, 1.099999999999996758 ) ) ;
#15380=PRESENTATION_STYLE_ASSIGNMENT (( #127113 ) ) ;
#15395=EDGE_LOOP ( 'NONE', ( #146551, #25720, #164995, #147572 ) ) ;
#15397=CIRCLE ( 'NONE', #43121, 0.08000000000000069555 ) ;
#15410=AXIS2_PLACEMENT_3D ( 'NONE', #185176, #167882, #118132 ) ;
#15442=( GEOMETRIC_REPRESENTATION_CONTEXT ( 3 ) GLOBAL_UNCERTAINTY_ASSIGNED_CONTEXT ( ( #162350 ) ) GLOBAL_UNIT_ASSIGNED_CONTEXT ( ( #46512, #113706, #97404 ) ) REPRESENTATION_CONTEXT ( 'NONE', 'WORKASPACE' ) );
#15453=CARTESIAN_POINT ( 'NONE',  ( 9.729489633724101694, 13.21513059140455759, -8.104625967152696120 ) ) ;
#15459=EDGE_LOOP ( 'NONE', ( #169150, #151400, #72684, #117556, #124402 ) ) ;
#15532=ADVANCED_FACE ( 'NONE', ( #201334 ), #52973, .F. ) ;
#15551=CARTESIAN_POINT ( 'NONE',  ( 9.412040618821951199, 14.12872955391332930, -8.482482427019883531 ) ) ;
#15583=CARTESIAN_POINT ( 'NONE',  ( -10.97409330344778944, 4.894225957061862253, -4.351021568302368969 ) ) ;
#15596=VECTOR ( 'NONE', #191566, 1000.000000000000000 ) ;
#15599=DIRECTION ( 'NONE',  ( 0.000000000000000000, 0.000000000000000000, 1.000000000000000000 ) ) ;
#15602=EDGE_CURVE ( 'NONE', #175384, #11599, #194446, .T. ) ;
#15605=CARTESIAN_POINT ( 'NONE',  ( -9.367496997601303832, 14.48154074412966175, 7.499999999995374367 ) ) ;
#15613=CARTESIAN_POINT ( 'NONE',  ( 10.19663671862204524, 10.80960751611106829, -6.241374320370645989 ) ) ;
#15666=CARTESIAN_POINT ( 'NONE',  ( -11.72945658997776519, 7.464408392728353547, -2.545424847964329995 ) ) ;
#15674=CARTESIAN_POINT ( 'NONE',  ( -11.62989982712325521, 8.355808186217915434, -2.970614550598404069 ) ) ;
#15678=( NAMED_UNIT ( * ) PLANE_ANGLE_UNIT ( ) SI_UNIT ( $, .RADIAN. ) );
#15688=ORIENTED_EDGE ( 'NONE', *, *, #79134, .F. ) ;
#15725=CARTESIAN_POINT ( 'NONE',  ( -10.59781858645781405, 12.29999999999997939, 3.302687032930891498 ) ) ;
#15726=DIRECTION ( 'NONE',  ( 0.9632918427306595976, 0.000000000000000000, -0.2684563758389253985 ) ) ;
#15733=FILL_AREA_STYLE ('',( #160948 ) ) ;
#15739=VECTOR ( 'NONE', #83387, 1000.000000000000000 ) ;
#15744=CARTESIAN_POINT ( 'NONE',  ( 9.574107575049751517, 3.767509416808738187, 7.159700411437358802 ) ) ;
#15748=TOROIDAL_SURFACE ( 'NONE', #188631, 11.92000000000000171, 0.08000000000000000167 ) ;
#15753=ORIENTED_EDGE ( 'NONE', *, *, #123817, .T. ) ;
#15788=VERTEX_POINT ( 'NONE', #29830 ) ;
#15792=FACE_BOUND ( 'NONE', #83613, .T. ) ;
#15819=CARTESIAN_POINT ( 'NONE',  ( -0.08053691275167716712, 15.51887838114830132, 11.99972973886013961 ) ) ;
#15838=DIRECTION ( 'NONE',  ( 0.000000000000000000, 0.000000000000000000, -1.000000000000000000 ) ) ;
#15840=VECTOR ( 'NONE', #107578, 1000.000000000000000 ) ;
#15851=B_SPLINE_CURVE_WITH_KNOTS ( 'NONE', 3,
 ( #133956, #33214, #197839, #135005, #151245, #101413 ),
 .UNSPECIFIED., .F., .F.,
 ( 4, 2, 4 ),
 ( 0.000000000000000000, 0.0003155923098472859139, 0.0006311846196945721530 ),
 .UNSPECIFIED. ) ;
#15896=DIRECTION ( 'NONE',  ( 0.8594003466332824637, -0.03762549425793430824, 0.5099170191202098135 ) ) ;
#15898=CARTESIAN_POINT ( 'NONE',  ( -15.75000000000000000, 11.29999999999999893, 0.6999999999999992895 ) ) ;
#15900=ADVANCED_FACE ( 'NONE', ( #81764 ), #159815, .F. ) ;
#15902=AXIS2_PLACEMENT_3D ( 'NONE', #107468, #124804, #89033 ) ;
#15907=CARTESIAN_POINT ( 'NONE',  ( -15.75000000000000000, 9.799999999999998934, 0.6999999999999992895 ) ) ;
#15958=CARTESIAN_POINT ( 'NONE',  ( 10.42905686949577060, 8.762263237317901243, 3.815400753447676152 ) ) ;
#15961=ORIENTED_EDGE ( 'NONE', *, *, #71135, .F. ) ;
#15968=DIRECTION ( 'NONE',  ( -0.000000000000000000, -1.000000000000000000, -0.000000000000000000 ) ) ;
#15987=CARTESIAN_POINT ( 'NONE',  ( 1.386567914617462760, 8.090296256147720300, 10.72428812184712044 ) ) ;
#16015=CARTESIAN_POINT ( 'NONE',  ( -10.84254087577847869, 4.919568073182958301, 5.035408296252059657 ) ) ;
#16025=ADVANCED_FACE ( 'NONE', ( #152102 ), #20996, .F. ) ;
#16157=FILL_AREA_STYLE_COLOUR ( '', #55709 ) ;
#16160=EDGE_CURVE ( 'NONE', #79990, #211004, #116451, .T. ) ;
#16163=CARTESIAN_POINT ( 'NONE',  ( 8.589851454039761691, 13.83000113107204143, 8.380017385823880005 ) ) ;
#16170=STYLED_ITEM ( 'NONE', ( #130869 ), #100155 ) ;
#16234=CARTESIAN_POINT ( 'NONE',  ( -11.43190902327453529, 11.15522128257853396, 3.649704988378119186 ) ) ;
#16247=CARTESIAN_POINT ( 'NONE',  ( -10.56141428364488277, 5.615930626961760375, 5.603115303083649579 ) ) ;
#16256=ORIENTED_EDGE ( 'NONE', *, *, #150960, .T. ) ;
#16262=COLOUR_RGB ( '', 0.08235294, 0.09019608, 0.10196078) ;
#16299=( LENGTH_UNIT ( ) NAMED_UNIT ( * ) SI_UNIT ( .MILLI., .METRE. ) );
#16300=ORIENTED_EDGE ( 'NONE', *, *, #102591, .F. ) ;
#16302=EDGE_CURVE ( 'NONE', #198860, #158402, #185431, .T. ) ;
#16308=CARTESIAN_POINT ( 'NONE',  ( -11.44779963594995387, 12.69999999999999041, -3.600000000000078693 ) ) ;
#16319=DIRECTION ( 'NONE',  ( 0.000000000000000000, 0.000000000000000000, 1.000000000000000000 ) ) ;
#16322=AXIS2_PLACEMENT_3D ( 'NONE', #36666, #53999, #87570 ) ;
#16328=VERTEX_POINT ( 'NONE', #9043 ) ;
#16334=PRESENTATION_STYLE_ASSIGNMENT (( #15276 ) ) ;
#16336=COLOUR_RGB ( '', 0.09019608, 0.27058824, 0.51372549) ;
#16371=ORIENTED_EDGE ( 'NONE', *, *, #31880, .F. ) ;
#16384=ORIENTED_EDGE ( 'NONE', *, *, #23869, .T. ) ;
#16402=CARTESIAN_POINT ( 'NONE',  ( -9.438383064689515933, 15.32552904735514687, -7.309821827856222143 ) ) ;
#16425=B_SPLINE_CURVE_WITH_KNOTS ( 'NONE', 3,
 ( #111007, #161841, #162902, #47030, #177012, #129417, #80573, #29703, #76303, #60052 ),
 .UNSPECIFIED., .F., .F.,
 ( 4, 2, 2, 2, 4 ),
 ( 0.000000000000000000, 0.2499999999999998890, 0.4999999999999998890, 0.7500000000000000000, 1.000000000000000000 ),
 .UNSPECIFIED. ) ;
#16430=FACE_OUTER_BOUND ( 'NONE', #140565, .T. ) ;
#16434=CARTESIAN_POINT ( 'NONE',  ( 0.000000000000000000, 19.00000000000000000, 0.000000000000000000 ) ) ;
#16454=PLANE ( 'NONE',  #175134 ) ;
#16455=CARTESIAN_POINT ( 'NONE',  ( 11.94980361058168938, 10.90000000000000036, -1.100000000000000311 ) ) ;
#16469=CARTESIAN_POINT ( 'NONE',  ( 0.07926560466934955140, 14.48322640536331818, 11.99972816967691891 ) ) ;
#16504=DIRECTION ( 'NONE',  ( 0.000000000000000000, -1.000000000000000000, 0.000000000000000000 ) ) ;
#16515=CARTESIAN_POINT ( 'NONE',  ( 12.20411482740001574, 8.058544339043594462, 4.983824382154795174 ) ) ;
#16517=EDGE_LOOP ( 'NONE', ( #60543, #107253, #189168, #213500 ) ) ;
#16571=CARTESIAN_POINT ( 'NONE',  ( -11.93239723206674618, 7.875908177015204181, -1.297019848843022238 ) ) ;
#16596=( GEOMETRIC_REPRESENTATION_CONTEXT ( 3 ) GLOBAL_UNCERTAINTY_ASSIGNED_CONTEXT ( ( #200168 ) ) GLOBAL_UNIT_ASSIGNED_CONTEXT ( ( #60805, #78116, #144246 ) ) REPRESENTATION_CONTEXT ( 'NONE', 'WORKASPACE' ) );
#16616=CARTESIAN_POINT ( 'NONE',  ( 9.212836904423678419, 13.91817412819898259, -6.903416813961001708 ) ) ;
#16636=CARTESIAN_POINT ( 'NONE',  ( 11.94105721237523277, 13.40000000000000036, -1.187919463087249827 ) ) ;
#16651=VECTOR ( 'NONE', #114883, 1000.000000000000000 ) ;
#16659=B_SPLINE_CURVE_WITH_KNOTS ( 'NONE', 3,
 ( #97548, #32522, #98597, #24515, #181953, #90625 ),
 .UNSPECIFIED., .F., .F.,
 ( 4, 2, 4 ),
 ( 0.000000000000000000, 0.0003845013059668464604, 0.0007690026119336929207 ),
 .UNSPECIFIED. ) ;
#16677=CARTESIAN_POINT ( 'NONE',  ( 10.72165486764792952, 9.918110100757866476, -5.398860479493060360 ) ) ;
#16682=CIRCLE ( 'NONE', #137789, 11.18000000000000149 ) ;
#16685=DIRECTION ( 'NONE',  ( 5.578174157656880098E-15, 1.000000000000000000, 7.437565543542506798E-15 ) ) ;
#16690=CARTESIAN_POINT ( 'NONE',  ( 11.86239285000045918, 12.29999999999999716, -1.812080536912752837 ) ) ;
#16712=DIRECTION ( 'NONE',  ( 0.000000000000000000, 0.000000000000000000, 1.000000000000000000 ) ) ;
#16724=CARTESIAN_POINT ( 'NONE',  ( -11.89204169242383458, 12.30000000000000071, -0.8046421800350854747 ) ) ;
#16726=CARTESIAN_POINT ( 'NONE',  ( -11.72847922660204034, 7.461677940835538259, 2.549820816093626430 ) ) ;
#16770=ORIENTED_EDGE ( 'NONE', *, *, #29782, .F. ) ;
#16782=( LENGTH_UNIT ( ) NAMED_UNIT ( * ) SI_UNIT ( .MILLI., .METRE. ) );
#16785=CARTESIAN_POINT ( 'NONE',  ( 11.33772463945043718, 13.40000000000000924, -3.600000000000078693 ) ) ;
#16792=( NAMED_UNIT ( * ) PLANE_ANGLE_UNIT ( ) SI_UNIT ( $, .RADIAN. ) );
#16807=EDGE_CURVE ( 'NONE', #166496, #128985, #145500, .T. ) ;
#16811=ORIENTED_EDGE ( 'NONE', *, *, #179751, .T. ) ;
#16819=CARTESIAN_POINT ( 'NONE',  ( 11.33772463945037146, 13.39999999999998259, 3.679999999999999272 ) ) ;
#16872=SURFACE_STYLE_USAGE ( .BOTH. , #179418 ) ;
#16899=CARTESIAN_POINT ( 'NONE',  ( -7.247736482492233456, 16.00000000000443023, -10.57961706324464402 ) ) ;
#16927=VERTEX_POINT ( 'NONE', #64206 ) ;
#16928=ADVANCED_FACE ( 'NONE', ( #113021 ), #189146, .T. ) ;
#16934=TOROIDAL_SURFACE ( 'NONE', #165701, 11.92000000000000348, 0.08000000000000000167 ) ;
#16968=DIRECTION ( 'NONE',  ( 0.000000000000000000, 0.000000000000000000, -1.000000000000000000 ) ) ;
#16979=( GEOMETRIC_REPRESENTATION_CONTEXT ( 3 ) GLOBAL_UNCERTAINTY_ASSIGNED_CONTEXT ( ( #86164 ) ) GLOBAL_UNIT_ASSIGNED_CONTEXT ( ( #137126, #151244, #51611 ) ) REPRESENTATION_CONTEXT ( 'NONE', 'WORKASPACE' ) );
#16988=AXIS2_PLACEMENT_3D ( 'NONE', #30384, #180880, #196082 ) ;
#16992=EDGE_CURVE ( 'NONE', #143616, #210726, #150079, .T. ) ;
#16999=B_SPLINE_CURVE_WITH_KNOTS ( 'NONE', 3,
 ( #123771, #139953, #41384, #73859, #105315, #107495 ),
 .UNSPECIFIED., .F., .F.,
 ( 4, 2, 4 ),
 ( 0.000000000000000000, 0.0003779448103413554985, 0.0007558896206827109970 ),
 .UNSPECIFIED. ) ;
#17000=DIRECTION ( 'NONE',  ( 0.000000000000000000, 0.000000000000000000, 1.000000000000000000 ) ) ;
#17001=CARTESIAN_POINT ( 'NONE',  ( -10.78926753850537423, 5.463497890167042570, -6.588879020148982413 ) ) ;
#17002=( NAMED_UNIT ( * ) PLANE_ANGLE_UNIT ( ) SI_UNIT ( $, .RADIAN. ) );
#17017=CARTESIAN_POINT ( 'NONE',  ( 10.00676670411244196, 9.850953729071504128, -6.649899283857078736 ) ) ;
#17027=CARTESIAN_POINT ( 'NONE',  ( 9.297838506356004729, 13.23377696881822274, -6.730568833096490344 ) ) ;
#17038=CARTESIAN_POINT ( 'NONE',  ( 8.656189917073545459, 13.74873789216364628, -8.313119079178678206 ) ) ;
#17043=CARTESIAN_POINT ( 'NONE',  ( -11.07124251632621537, 13.79999999999999538, -0.8054525327832626758 ) ) ;
#17070=CARTESIAN_POINT ( 'NONE',  ( -9.586151930456434656, 15.23390131771004974, -7.218760142018259884 ) ) ;
#17079=CIRCLE ( 'NONE', #99986, 12.00000000000000178 ) ;
#17085=SURFACE_SIDE_STYLE ('',( #180672 ) ) ;
#17141=ORIENTED_EDGE ( 'NONE', *, *, #39340, .T. ) ;
#17183=ORIENTED_EDGE ( 'NONE', *, *, #182687, .T. ) ;
#17191=CARTESIAN_POINT ( 'NONE',  ( -9.445283354644308460, 14.68100100830176125, -7.300214616139029999 ) ) ;
#17204=CARTESIAN_POINT ( 'NONE',  ( 11.33772467203841572, 11.00732847981847584, 3.599999999999999201 ) ) ;
#17273=CARTESIAN_POINT ( 'NONE',  ( 11.91826849282518275, 10.19999999999999929, -1.400000000000001465 ) ) ;
#17288=( NAMED_UNIT ( * ) SI_UNIT ( $, .STERADIAN. ) SOLID_ANGLE_UNIT ( ) );
#17290=CARTESIAN_POINT ( 'NONE',  ( -10.14895191633106819, 5.000000000000002665, 7.601392964450658596 ) ) ;
#17305=AXIS2_PLACEMENT_3D ( 'NONE', #23184, #24255, #71934 ) ;
#17317=CARTESIAN_POINT ( 'NONE',  ( -11.59499170316466099, 8.293181854556747723, 2.924389865657003540 ) ) ;
#17334=( NAMED_UNIT ( * ) SI_UNIT ( $, .STERADIAN. ) SOLID_ANGLE_UNIT ( ) );
#17340=ORIENTED_EDGE ( 'NONE', *, *, #161282, .T. ) ;
#17396=CYLINDRICAL_SURFACE ( 'NONE', #132382, 0.07999999999999998779 ) ;
#17430=SURFACE_STYLE_FILL_AREA ( #47863 ) ;
#17435=CARTESIAN_POINT ( 'NONE',  ( -1.271070482941953461, 8.436788551174030815, 10.93994114196923739 ) ) ;
#17439=ORIENTED_EDGE ( 'NONE', *, *, #154446, .F. ) ;
#17445=ORIENTED_EDGE ( 'NONE', *, *, #35088, .F. ) ;
#17463=AXIS2_PLACEMENT_3D ( 'NONE', #62159, #128317, #194280 ) ;
#17543=CARTESIAN_POINT ( 'NONE',  ( 11.86145016429273014, 11.00587408513255028, 1.099999999999996536 ) ) ;
#17545=( BOUNDED_SURFACE ( )  B_SPLINE_SURFACE ( 3, 2, ( 
 ( #90002, #51356, #156055 ),
 ( #7643, #183471, #68635 ),
 ( #134759, #73728, #210107 ),
 ( #209035, #43383, #12978 ),
 ( #141969, #175511, #174456 ),
 ( #91070, #189608, #10840 ) ),
 .UNSPECIFIED., .F., .F., .F. ) 
 B_SPLINE_SURFACE_WITH_KNOTS ( ( 4, 2, 4 ),
 ( 3, 3 ),
 ( 0.000000000000000000, 0.0003766365702389427796, 0.0007532731404778855592 ),
 ( 0.000000000000000000, 1.000000000000000000 ),
 .UNSPECIFIED. ) 
 GEOMETRIC_REPRESENTATION_ITEM ( )  RATIONAL_B_SPLINE_SURFACE ( (
 ( 1.000000000000000000, 0.7452309222762957264, 1.000000000000000000),
 ( 1.000000000000000000, 0.7451892422671814176, 1.000000000000000000),
 ( 1.000000000000000000, 0.7429606254238495522, 1.000000000000000000),
 ( 1.000000000000000000, 0.7311462761265991039, 1.000000000000000000),
 ( 1.000000000000000000, 0.7212257702791110558, 1.000000000000000000),
 ( 1.000000000000000000, 0.7071067811865475727, 1.000000000000000000) ) ) 
 REPRESENTATION_ITEM ( '' )  SURFACE ( )  );
#17565=EDGE_CURVE ( 'NONE', #211004, #54861, #70560, .T. ) ;
#17567=CARTESIAN_POINT ( 'NONE',  ( 11.33772463945037146, 13.39999999999998259, 3.599999999999999201 ) ) ;
#17589=CARTESIAN_POINT ( 'NONE',  ( -5.600986303897101948, 14.48156060235217701, 10.62204783317221235 ) ) ;
#17634=CARTESIAN_POINT ( 'NONE',  ( -11.13976883071979174, 5.784892963039250269, 4.476295437483729600 ) ) ;
#17650=ORIENTED_EDGE ( 'NONE', *, *, #14127, .T. ) ;
#17660=PLANE ( 'NONE',  #194342 ) ;
#17678=CARTESIAN_POINT ( 'NONE',  ( 8.353377556026709172, 13.12787966248234284, -8.539254890958119404 ) ) ;
#17706=CARTESIAN_POINT ( 'NONE',  ( -10.57232049882948388, 5.599334429189661400, -4.968988939937085014 ) ) ;
#17735=CARTESIAN_POINT ( 'NONE',  ( 11.89942855770814312, 11.29999999999999893, -0.7000000000000009548 ) ) ;
#17743=CARTESIAN_POINT ( 'NONE',  ( 10.59781858645781405, 11.29999999999997762, 3.302687032930892830 ) ) ;
#17773=CARTESIAN_POINT ( 'NONE',  ( -5.973258884348944697, 14.55272284716803455, -10.36629430815492903 ) ) ;
#17793=CARTESIAN_POINT ( 'NONE',  ( -11.86239285000045918, 13.87999999999998302, 1.812080536912751061 ) ) ;
#17815=B_SPLINE_CURVE_WITH_KNOTS ( 'NONE', 3,
 ( #71482, #41165, #25946, #158109, #203611, #106196 ),
 .UNSPECIFIED., .F., .F.,
 ( 4, 2, 4 ),
 ( 0.000000000000000000, 0.0003144386176887254184, 0.0006288772353774508368 ),
 .UNSPECIFIED. ) ;
#17839=ORIENTED_EDGE ( 'NONE', *, *, #9224, .F. ) ;
#17844=CARTESIAN_POINT ( 'NONE',  ( -0.08011318657386623521, 15.51804218995383167, 11.99973258272403775 ) ) ;
#17845=CARTESIAN_POINT ( 'NONE',  ( 11.48243876534946217, 13.79999999999999893, -3.200000000000001510 ) ) ;
#17886=CARTESIAN_POINT ( 'NONE',  ( -15.75000000000000000, 10.90000000000000036, -1.100000000000002087 ) ) ;
#17901=MECHANICAL_DESIGN_GEOMETRIC_PRESENTATION_REPRESENTATION('',(#52108),#45637);
#17908=ORIENTED_EDGE ( 'NONE', *, *, #48845, .T. ) ;
#17914=DIRECTION ( 'NONE',  ( -6.938893903907222067E-15, -1.000000000000000000, 0.000000000000000000 ) ) ;
#17963=CARTESIAN_POINT ( 'NONE',  ( -9.898321827452971178, 16.00000000001253753, -7.924999999985292476 ) ) ;
#17965=CARTESIAN_POINT ( 'NONE',  ( -10.99318506637795956, 6.209869560752310669, 6.173358988436974393 ) ) ;
#17986=ORIENTED_EDGE ( 'NONE', *, *, #201940, .T. ) ;
#17993=UNCERTAINTY_MEASURE_WITH_UNIT (LENGTH_MEASURE( 1.000000000000000082E-05 ), #71744, 'distance_accuracy_value', 'NONE');
#17997=CARTESIAN_POINT ( 'NONE',  ( 11.55950211276791251, 13.87999999999998302, 3.221476510067114329 ) ) ;
#18005=DIRECTION ( 'NONE',  ( 0.000000000000000000, -1.000000000000000000, -0.000000000000000000 ) ) ;
#18057=ORIENTED_EDGE ( 'NONE', *, *, #193087, .F. ) ;
#18066=CARTESIAN_POINT ( 'NONE',  ( -10.22593938286385296, 3.000029897349846930, -7.498676971688964521 ) ) ;
#18083=CARTESIAN_POINT ( 'NONE',  ( 9.442551103936683177, 11.02991041777048231, 7.411286945868026166 ) ) ;
#18087=ORIENTED_EDGE ( 'NONE', *, *, #57719, .T. ) ;
#18095=CARTESIAN_POINT ( 'NONE',  ( 9.992730418911948576, 9.901705038286040761, 5.020517729075291591 ) ) ;
#18101=VECTOR ( 'NONE', #204232, 1000.000000000000000 ) ;
#18106=CARTESIAN_POINT ( 'NONE',  ( 7.704073495075588696, 14.42981585874038153, -9.201162189417628312 ) ) ;
#18109=CARTESIAN_POINT ( 'NONE',  ( -11.86239285000045918, 12.22000000000000064, -1.812080536912752837 ) ) ;
#18112=DIRECTION ( 'NONE',  ( -1.000000000000000000, 0.000000000000000000, 1.224646799147352961E-16 ) ) ;
#18128=ORIENTED_EDGE ( 'NONE', *, *, #51352, .F. ) ;
#18169=VECTOR ( 'NONE', #151795, 1000.000000000000000 ) ;
#18182=PRESENTATION_STYLE_ASSIGNMENT (( #149271 ) ) ;
#18224=CARTESIAN_POINT ( 'NONE',  ( 8.868625083907582862, 12.79269056714098163, -8.084906220447308556 ) ) ;
#18263=LINE ( 'NONE', #84347, #90355 ) ;
#18266=AXIS2_PLACEMENT_3D ( 'NONE', #164196, #60551, #182550 ) ;
#18296=CARTESIAN_POINT ( 'NONE',  ( 9.533882584321561993, 4.462909869062322343, -7.287958590253622582 ) ) ;
#18346=ADVANCED_FACE ( 'NONE', ( #34725 ), #88979, .T. ) ;
#18350=CIRCLE ( 'NONE', #129010, 0.08000000000000020983 ) ;
#18366=CARTESIAN_POINT ( 'NONE',  ( 8.937284900545680699, 14.72974997456996604, 8.011501044423479101 ) ) ;
#18367=CARTESIAN_POINT ( 'NONE',  ( -11.01135777277261951, 13.50625186781170584, 1.399999999999998579 ) ) ;
#18368=CARTESIAN_POINT ( 'NONE',  ( -9.979842676043658045, 5.589819607760296627, 5.978770845575332338 ) ) ;
#18377=CARTESIAN_POINT ( 'NONE',  ( -11.44779963594995564, 10.89999999999999147, 3.600000000000075140 ) ) ;
#18379=EDGE_LOOP ( 'NONE', ( #118238, #22959, #162068, #139156 ) ) ;
#18391=CARTESIAN_POINT ( 'NONE',  ( -11.77320363351223342, 8.651382856832046997, 2.094678198626021892 ) ) ;
#18422=MECHANICAL_DESIGN_GEOMETRIC_PRESENTATION_REPRESENTATION('',(#15000),#21955);
#18427=AXIS2_PLACEMENT_3D ( 'NONE', #196777, #114532, #65675 ) ;
#18437=CARTESIAN_POINT ( 'NONE',  ( 11.86145016429272836, 19.00000000000000000, -1.180000000000002158 ) ) ;
#18446=VERTEX_POINT ( 'NONE', #85618 ) ;
#18449=DIRECTION ( 'NONE',  ( 5.578174157656880098E-15, 1.000000000000000000, -7.437565543542506798E-15 ) ) ;
#18453=CARTESIAN_POINT ( 'NONE',  ( 11.41381675112453387, 10.19999999999998153, 3.704697986577180746 ) ) ;
#18470=VERTEX_POINT ( 'NONE', #1145 ) ;
#18483=VECTOR ( 'NONE', #54291, 1000.000000000000000 ) ;
#18484=CIRCLE ( 'NONE', #184541, 12.00000000000000178 ) ;
#18489=ORIENTED_EDGE ( 'NONE', *, *, #125962, .F. ) ;
#18514=CARTESIAN_POINT ( 'NONE',  ( -10.19097401674926395, 4.476076320095182304, 5.708917106338025960 ) ) ;
#18531=VERTEX_POINT ( 'NONE', #126474 ) ;
#18543=CARTESIAN_POINT ( 'NONE',  ( -9.380156870149196635, 15.46908192400845827, -7.484187822904944554 ) ) ;
#18550=CARTESIAN_POINT ( 'NONE',  ( -11.97929049433705373, 9.719999999999998863, 0.7046979865771783036 ) ) ;
#18565=CARTESIAN_POINT ( 'NONE',  ( 0.000000000000000000, 3.481548657788671619, 0.000000000000000000 ) ) ;
#18569=DIRECTION ( 'NONE',  ( 0.000000000000000000, 0.000000000000000000, 1.000000000000000000 ) ) ;
#18571=DIRECTION ( 'NONE',  ( 0.5994789404140892231, -9.687429098727955365E-15, 0.8003905296791066215 ) ) ;
#18578=AXIS2_PLACEMENT_3D ( 'NONE', #90085, #109592, #188628 ) ;
#18629=DIRECTION ( 'NONE',  ( 1.000000000000000000, -8.267061968666011278E-31, -1.224646799147343593E-16 ) ) ;
#18645=AXIS2_PLACEMENT_3D ( 'NONE', #138656, #190572, #90978 ) ;
#18647=CARTESIAN_POINT ( 'NONE',  ( -11.83627402213341107, 4.942735150756283780, -4.855302456647772935 ) ) ;
#18658=CARTESIAN_POINT ( 'NONE',  ( 9.897453898556438645, 12.56651866558563313, 7.888353118025118071 ) ) ;
#18670=EDGE_LOOP ( 'NONE', ( #43333, #56028, #35683, #20544 ) ) ;
#18675=CARTESIAN_POINT ( 'NONE',  ( 11.96533679318060095, 12.34753988812994763, -0.9151144679398871551 ) ) ;
#18689=VECTOR ( 'NONE', #44044, 1000.000000000000000 ) ;
#18704=CARTESIAN_POINT ( 'NONE',  ( -11.04536101718726293, 12.69999999999999929, -1.100000000000000311 ) ) ;
#18706=CARTESIAN_POINT ( 'NONE',  ( -10.97260011637327182, 3.256560822415822454, -6.404599650317903681 ) ) ;
#18707=CARTESIAN_POINT ( 'NONE',  ( 1.469576158976824144E-15, 19.00000000000000000, 12.00000000000000178 ) ) ;
#18710=CARTESIAN_POINT ( 'NONE',  ( -11.99967559429689778, 8.028203318877215722, 0.5374089444583232122 ) ) ;
#18724=ORIENTED_EDGE ( 'NONE', *, *, #15602, .T. ) ;
#18754=CARTESIAN_POINT ( 'NONE',  ( 8.213514019010339950, 13.37925768050776298, -8.583069077171659345 ) ) ;
#18760=EDGE_LOOP ( 'NONE', ( #130636, #200012, #80742, #66766 ) ) ;
#18771=CARTESIAN_POINT ( 'NONE',  ( -9.768463870713130603, 4.463474924597734095, -6.895317384053313070 ) ) ;
#18808=CARTESIAN_POINT ( 'NONE',  ( 9.577100139991578942, 12.68281731961604564, -7.233471777081839527 ) ) ;
#18812=CARTESIAN_POINT ( 'NONE',  ( 11.94105721839855505, 13.52698343341124421, -1.187919402540330127 ) ) ;
#18820=CARTESIAN_POINT ( 'NONE',  ( 10.56536251450128994, 11.25961062549474612, 3.404319718479180690 ) ) ;
#18857=PRESENTATION_STYLE_ASSIGNMENT (( #133737 ) ) ;
#18869=CARTESIAN_POINT ( 'NONE',  ( -11.63630038494604690, 8.312388184584818873, 2.945693487284683165 ) ) ;
#18886=PRESENTATION_STYLE_ASSIGNMENT (( #487 ) ) ;
#18910=ORIENTED_EDGE ( 'NONE', *, *, #52547, .F. ) ;
#18913=CARTESIAN_POINT ( 'NONE',  ( 11.78331023100045627, 13.88000000000000078, -1.800000000000001155 ) ) ;
#18929=AXIS2_PLACEMENT_3D ( 'NONE', #178318, #51231, #193483 ) ;
#18996=COLOUR_RGB ( '', 0.31764706, 0.68627451, 0.89019608) ;
#19036=B_SPLINE_CURVE_WITH_KNOTS ( 'NONE', 3,
 ( #144977, #17043, #132987, #210982, #131929, #100449 ),
 .UNSPECIFIED., .F., .F.,
 ( 4, 2, 4 ),
 ( 0.001877801214402442754, 0.002190719108449961511, 0.002503637002497480051 ),
 .UNSPECIFIED. ) ;
#19038=CARTESIAN_POINT ( 'NONE',  ( -3.501245407923943898, 16.00000000000493117, -11.28115623562582748 ) ) ;
#19040=CARTESIAN_POINT ( 'NONE',  ( -10.05286969158539812, 5.876479340494690895, 5.831501649199077875 ) ) ;
#19080=PRESENTATION_STYLE_ASSIGNMENT (( #4937 ) ) ;
#19081=CYLINDRICAL_SURFACE ( 'NONE', #1016, 0.3999999999999997446 ) ;
#19094=AXIS2_PLACEMENT_3D ( 'NONE', #93354, #144268, #177789 ) ;
#19130=AXIS2_PLACEMENT_3D ( 'NONE', #195268, #29569, #13304 ) ;
#19136=ORIENTED_EDGE ( 'NONE', *, *, #189421, .T. ) ;
#19138=EDGE_CURVE ( 'NONE', #170509, #198869, #28463, .T. ) ;
#19143=CARTESIAN_POINT ( 'NONE',  ( -10.52626310920980757, 3.679096435225583939, -5.196420034295205603 ) ) ;
#19151=DIRECTION ( 'NONE',  ( 0.000000000000000000, 0.000000000000000000, -1.000000000000000000 ) ) ;
#19155=CARTESIAN_POINT ( 'NONE',  ( -11.69380381030441107, 8.410673437356566140, -1.083569014401829955 ) ) ;
#19161=CARTESIAN_POINT ( 'NONE',  ( 11.35739107624612210, 7.533900434079529695, -3.740981627317509606 ) ) ;
#19172=CARTESIAN_POINT ( 'NONE',  ( 9.270933768482571224, 13.53532804777227661, 6.807664277187561730 ) ) ;
#19175=VERTEX_POINT ( 'NONE', #194584 ) ;
#19197=CARTESIAN_POINT ( 'NONE',  ( -15.75000000000000000, 11.29999999999998117, 3.199999999999997957 ) ) ;
#19282=( GEOMETRIC_REPRESENTATION_CONTEXT ( 3 ) GLOBAL_UNCERTAINTY_ASSIGNED_CONTEXT ( ( #84284 ) ) GLOBAL_UNIT_ASSIGNED_CONTEXT ( ( #8436, #60392, #174183 ) ) REPRESENTATION_CONTEXT ( 'NONE', 'WORKASPACE' ) );
#19294=CARTESIAN_POINT ( 'NONE',  ( 11.33772465723237666, 12.59131699265169502, 3.600000000000073364 ) ) ;
#19314=EDGE_CURVE ( 'NONE', #138623, #175932, #78589, .T. ) ;
#19315=CARTESIAN_POINT ( 'NONE',  ( -9.367496996949647325, 15.51845925588232333, 7.500000000809289524 ) ) ;
#19347=DIRECTION ( 'NONE',  ( 0.7806247497998004548, 0.000000000000000000, 0.6249999999999992228 ) ) ;
#19351=CARTESIAN_POINT ( 'NONE',  ( 11.44779963594988814, 13.39999999999998614, 3.600000000000001421 ) ) ;
#19365=CARTESIAN_POINT ( 'NONE',  ( 9.534402287735492365, 3.538071065864172304, -7.287264613139948111 ) ) ;
#19368=DIRECTION ( 'NONE',  ( 0.000000000000000000, 1.000000000000000000, 0.000000000000000000 ) ) ;
#19373=LINE ( 'NONE', #153669, #53298 ) ;
#19400=GEOMETRIC_CURVE_SET ( 'NONE', ( #57871, #104305, #96668, #44855, #140389, #26801, #83573, #153404, #16425, #65515, #192124, #34459 ) ) ;
#19403=COLOUR_RGB ( '', 0.08235294, 0.09019608, 0.10196078) ;
#19427=ORIENTED_EDGE ( 'NONE', *, *, #83347, .T. ) ;
#19430=CARTESIAN_POINT ( 'NONE',  ( -10.48284956170200921, 5.077895721165493370, 7.121295720048954614 ) ) ;
#19443=STYLED_ITEM ( 'NONE', ( #187405 ), #146775 ) ;
#19457=COLOUR_RGB ( '', 0.40784314, 0.44705882, 0.49803922) ;
#19480=ORIENTED_EDGE ( 'NONE', *, *, #203350, .T. ) ;
#19485=( BOUNDED_SURFACE ( )  B_SPLINE_SURFACE ( 3, 2, ( 
 ( #163, #201571, #136615 ),
 ( #38039, #104108, #119348 ),
 ( #132378, #198379, #50020 ),
 ( #116144, #140907, #73729 ),
 ( #72653, #172307, #121502 ),
 ( #27102, #109505, #175512 ) ),
 .UNSPECIFIED., .F., .F., .T. ) 
 B_SPLINE_SURFACE_WITH_KNOTS ( ( 4, 2, 4 ),
 ( 3, 3 ),
 ( 0.000000000000000000, 0.0003766365702389427254, 0.0007532731404778854507 ),
 ( 0.000000000000000000, 1.000000000000000000 ),
 .UNSPECIFIED. ) 
 GEOMETRIC_REPRESENTATION_ITEM ( )  RATIONAL_B_SPLINE_SURFACE ( (
 ( 1.000000000000000000, 0.7452309222762957264, 1.000000000000000000),
 ( 1.000000000000000000, 0.7451892422669574856, 1.000000000000000000),
 ( 1.000000000000000000, 0.7429606254241496455, 1.000000000000000000),
 ( 1.000000000000000000, 0.7311462761262990107, 1.000000000000000000),
 ( 1.000000000000000000, 0.7212257702793347658, 1.000000000000000000),
 ( 1.000000000000000000, 0.7071067811865475727, 1.000000000000000000) ) ) 
 REPRESENTATION_ITEM ( '' )  SURFACE ( )  );
#19488=CARTESIAN_POINT ( 'NONE',  ( -11.07131242353766254, 9.799999999999998934, -0.8043462106219255725 ) ) ;
#19516=CARTESIAN_POINT ( 'NONE',  ( -11.35569630219380777, 12.48731560708633914, -3.554478010595065296 ) ) ;
#19530=EDGE_CURVE ( 'NONE', #61984, #211122, #102873, .T. ) ;
#19543=DIRECTION ( 'NONE',  ( 0.000000000000000000, 0.000000000000000000, -1.000000000000000000 ) ) ;
#19551=AXIS2_PLACEMENT_3D ( 'NONE', #163546, #193898, #79081 ) ;
#19563=EDGE_CURVE ( 'NONE', #185203, #105543, #113688, .T. ) ;
#19583=CARTESIAN_POINT ( 'NONE',  ( -9.811677024507259759, 4.107325997343203028, 6.339424533126782002 ) ) ;
#19612=STYLED_ITEM ( 'NONE', ( #135238 ), #147970 ) ;
#19613=CARTESIAN_POINT ( 'NONE',  ( -9.434262096590540381, 15.42050698104736739, -7.415936069015691245 ) ) ;
#19622=COLOUR_RGB ( '', 0.09019608, 0.27058824, 0.51372549) ;
#19630=VERTEX_POINT ( 'NONE', #68818 ) ;
#19633=CARTESIAN_POINT ( 'NONE',  ( 11.84668730067608244, 12.59363775091781079, -1.400000000000002132 ) ) ;
#19640=CARTESIAN_POINT ( 'NONE',  ( -11.80251051724185984, 12.30000000000000071, -1.695257889419022002 ) ) ;
#19657=VERTEX_POINT ( 'NONE', #162409 ) ;
#19667=ORIENTED_EDGE ( 'NONE', *, *, #103048, .T. ) ;
#19692=ORIENTED_EDGE ( 'NONE', *, *, #138353, .T. ) ;
#19698=CARTESIAN_POINT ( 'NONE',  ( 11.44779965693254375, 10.10313923201305997, -3.599999932276613190 ) ) ;
#19705=ORIENTED_EDGE ( 'NONE', *, *, #82182, .F. ) ;
#19710=CARTESIAN_POINT ( 'NONE',  ( 10.95308175811721085, 13.79999999999999893, -1.800000000000001155 ) ) ;
#19717=CARTESIAN_POINT ( 'NONE',  ( -11.80100919632472589, 4.809168931535662495, -4.927235675632552159 ) ) ;
#19741=CARTESIAN_POINT ( 'NONE',  ( 11.89942855770813956, 12.30000000000000071, -0.7000000000000009548 ) ) ;
#19778=CARTESIAN_POINT ( 'NONE',  ( -10.43230948805442893, 5.066484524551064794, 5.254757398418679060 ) ) ;
#19825=CARTESIAN_POINT ( 'NONE',  ( 7.121823250997191046, 13.97725337314594007, -9.255175167006054693 ) ) ;
#19829=STYLED_ITEM ( 'NONE', ( #74660 ), #20283 ) ;
#19842=CARTESIAN_POINT ( 'NONE',  ( 11.84668730067608244, 13.40000000000000036, -1.400000000000001688 ) ) ;
#19871=ORIENTED_EDGE ( 'NONE', *, *, #81363, .T. ) ;
#19875=CARTESIAN_POINT ( 'NONE',  ( 7.459735474692968715, 15.41013697600841859, 9.344700516680960689 ) ) ;
#19877=ORIENTED_EDGE ( 'NONE', *, *, #129757, .T. ) ;
#19892=DIRECTION ( 'NONE',  ( 0.000000000000000000, 1.000000000000000000, 0.000000000000000000 ) ) ;
#19895=AXIS2_PLACEMENT_3D ( 'NONE', #25728, #175215, #123341 ) ;
#19903=AXIS2_PLACEMENT_3D ( 'NONE', #156088, #75893, #59638 ) ;
#19928=CARTESIAN_POINT ( 'NONE',  ( -11.94980361490462784, 12.59667875264138992, -1.099999952232860512 ) ) ;
#19944=ORIENTED_EDGE ( 'NONE', *, *, #89552, .F. ) ;
#19956=CARTESIAN_POINT ( 'NONE',  ( -15.75000000000000000, 10.19999999999999929, -3.200000000000001510 ) ) ;
#19959=VERTEX_POINT ( 'NONE', #45373 ) ;
#19983=LINE ( 'NONE', #71924, #30603 ) ;
#19985=CARTESIAN_POINT ( 'NONE',  ( -9.800888885521233718, 4.518459255872631530, 6.931788714247765881 ) ) ;
#19990=CIRCLE ( 'NONE', #141130, 0.08000000000000020983 ) ;
#19995=CARTESIAN_POINT ( 'NONE',  ( 1.500000000000039524, 7.000000000000000000, 10.99818166789400742 ) ) ;
#19996=SURFACE_STYLE_USAGE ( .BOTH. , #37325 ) ;
#20002=TOROIDAL_SURFACE ( 'NONE', #2828, 11.92000000000000171, 0.08000000000000000167 ) ;
#20038=ORIENTED_EDGE ( 'NONE', *, *, #154690, .F. ) ;
#20045=DIRECTION ( 'NONE',  ( 0.000000000000000000, 1.000000000000000000, 0.000000000000000000 ) ) ;
#20054=DIRECTION ( 'NONE',  ( 0.000000000000000000, 7.228014483236694583E-17, -1.000000000000000000 ) ) ;
#20101=CARTESIAN_POINT ( 'NONE',  ( -3.501245407923692099, 15.00000000000335731, -11.28115623562607794 ) ) ;
#20104=CARTESIAN_POINT ( 'NONE',  ( -10.01587959479698320, 5.734125918284786572, -5.906598880481439551 ) ) ;
#20115=VERTEX_POINT ( 'NONE', #174316 ) ;
#20127=ORIENTED_EDGE ( 'NONE', *, *, #55681, .T. ) ;
#20143=SURFACE_STYLE_USAGE ( .BOTH. , #104628 ) ;
#20144=FILL_AREA_STYLE ('',( #168548 ) ) ;
#20207=CARTESIAN_POINT ( 'NONE',  ( -10.97260011637327182, 3.256560822415822454, -6.404599650317903681 ) ) ;
#20223=CARTESIAN_POINT ( 'NONE',  ( 9.304767520285516014, 11.47811317756902660, 7.581012809288346865 ) ) ;
#20233=VERTEX_POINT ( 'NONE', #73585 ) ;
#20235=DIRECTION ( 'NONE',  ( 0.000000000000000000, -1.000000000000000000, -0.000000000000000000 ) ) ;
#20236=CARTESIAN_POINT ( 'NONE',  ( 10.14838338295609077, 13.59592256598955018, 7.283497017817778918 ) ) ;
#20239=ORIENTED_EDGE ( 'NONE', *, *, #76805, .F. ) ;
#20246=EDGE_CURVE ( 'NONE', #112981, #172406, #2561, .T. ) ;
#20249=CARTESIAN_POINT ( 'NONE',  ( -1.797526709181193283, 15.47023744923392385, -11.89807871921767735 ) ) ;
#20280=SURFACE_SIDE_STYLE ('',( #184910 ) ) ;
#20283=MANIFOLD_SOLID_BREP ( 'Fillet1', #32676 ) ;
#20298=STYLED_ITEM ( 'NONE', ( #24560 ), #212553 ) ;
#20303=VERTEX_POINT ( 'NONE', #207842 ) ;
#20312=AXIS2_PLACEMENT_3D ( 'NONE', #72256, #53900, #120036 ) ;
#20329=CARTESIAN_POINT ( 'NONE',  ( 11.33772463945036790, 12.69999999999999929, -3.600000000000000977 ) ) ;
#20354=ORIENTED_EDGE ( 'NONE', *, *, #11240, .T. ) ;
#20367=AXIS2_PLACEMENT_3D ( 'NONE', #165931, #148622, #149685 ) ;
#20380=EDGE_CURVE ( 'NONE', #37994, #72298, #51707, .T. ) ;
#20381=( NAMED_UNIT ( * ) PLANE_ANGLE_UNIT ( ) SI_UNIT ( $, .RADIAN. ) );
#20388=DIRECTION ( 'NONE',  ( 1.000000000000000000, -0.000000000000000000, -0.000000000000000000 ) ) ;
#20399=FACE_OUTER_BOUND ( 'NONE', #197140, .T. ) ;
#20418=CARTESIAN_POINT ( 'NONE',  ( 11.48767021851169190, 13.83004227463828784, 3.470194894594622159 ) ) ;
#20492=ORIENTED_EDGE ( 'NONE', *, *, #72514, .F. ) ;
#20496=CARTESIAN_POINT ( 'NONE',  ( -10.19097401674926395, 4.476076320095182304, 5.708917106338025960 ) ) ;
#20518=B_SPLINE_CURVE_WITH_KNOTS ( 'NONE', 3,
 ( #79233, #111807, #98686, #130195, #97637, #163694 ),
 .UNSPECIFIED., .F., .F.,
 ( 4, 2, 4 ),
 ( 0.0006378314054480077946, 0.0009584618939205538689, 0.001279092382393099943 ),
 .UNSPECIFIED. ) ;
#20544=ORIENTED_EDGE ( 'NONE', *, *, #60132, .F. ) ;
#20563=CARTESIAN_POINT ( 'NONE',  ( -11.97929049433705551, 11.37999999999999901, 0.7046979865771804130 ) ) ;
#20575=CARTESIAN_POINT ( 'NONE',  ( -11.80248046418316044, 13.79999999999999893, -1.695421849633145017 ) ) ;
#20579=DIRECTION ( 'NONE',  ( 0.000000000000000000, 7.254698431490414842E-17, -1.000000000000000000 ) ) ;
#20590=CARTESIAN_POINT ( 'NONE',  ( -11.86145016429273014, 10.19999999999999929, -1.180000000000002158 ) ) ;
#20600=CARTESIAN_POINT ( 'NONE',  ( 0.000000000000000000, 13.87999999999998302, 0.000000000000000000 ) ) ;
#20635=CARTESIAN_POINT ( 'NONE',  ( -10.82994025801865590, 5.589394046361075397, 6.507174183487985708 ) ) ;
#20636=EDGE_LOOP ( 'NONE', ( #39828, #2259, #46682, #114349 ) ) ;
#20649=CARTESIAN_POINT ( 'NONE',  ( -11.84668730067608422, 10.90000000000000036, -1.320000000000001616 ) ) ;
#20656=CARTESIAN_POINT ( 'NONE',  ( -0.001697653062873135657, 15.43814226012838375, 11.93887736635299213 ) ) ;
#20671=SURFACE_STYLE_USAGE ( .BOTH. , #3349 ) ;
#20673=ORIENTED_EDGE ( 'NONE', *, *, #99741, .F. ) ;
#20674=LINE ( 'NONE', #66211, #64268 ) ;
#20687=CARTESIAN_POINT ( 'NONE',  ( -10.62808266865025608, 4.100636420088800804, -5.574739771788820519 ) ) ;
#20693=CARTESIAN_POINT ( 'NONE',  ( -11.92619526913699879, 12.69999999999999929, -1.328859060402686199 ) ) ;
#20726=EDGE_CURVE ( 'NONE', #23505, #163825, #26798, .T. ) ;
#20731=CARTESIAN_POINT ( 'NONE',  ( 1.369155121446740960E-15, 19.00000000000000000, -11.18000000000000149 ) ) ;
#20737=FILL_AREA_STYLE_COLOUR ( '', #184176 ) ;
#20754=( BOUNDED_SURFACE ( )  B_SPLINE_SURFACE ( 3, 2, ( 
 ( #24953, #121488, #91055 ),
 ( #56404, #4413, #72638 ),
 ( #54274, #187460, #39088 ),
 ( #70484, #154973, #136600 ),
 ( #40158, #156038, #106272 ),
 ( #172293, #23881, #7627 ) ),
 .UNSPECIFIED., .F., .F., .T. ) 
 B_SPLINE_SURFACE_WITH_KNOTS ( ( 4, 2, 4 ),
 ( 3, 3 ),
 ( 0.000000000000000000, 0.0003754691837024765901, 0.0007509383674049531802 ),
 ( 0.000000000000000000, 1.000000000000000000 ),
 .UNSPECIFIED. ) 
 GEOMETRIC_REPRESENTATION_ITEM ( )  RATIONAL_B_SPLINE_SURFACE ( (
 ( 1.000000000000000000, 0.6711954675835395401, 1.000000000000000000),
 ( 1.000000000000000000, 0.6709646295273183902, 1.000000000000000000),
 ( 1.000000000000000000, 0.6771840716651685854, 1.000000000000000000),
 ( 1.000000000000000000, 0.6927481755874828062, 1.000000000000000000),
 ( 1.000000000000000000, 0.7017972101304553734, 1.000000000000000000),
 ( 1.000000000000000000, 0.7071067811865399122, 1.000000000000000000) ) ) 
 REPRESENTATION_ITEM ( '' )  SURFACE ( )  );
#20756=ORIENTED_EDGE ( 'NONE', *, *, #151575, .F. ) ;
#20784=EDGE_LOOP ( 'NONE', ( #10984, #122377, #4421, #39009 ) ) ;
#20795=DIRECTION ( 'NONE',  ( 1.000000000000000000, -0.000000000000000000, -0.000000000000000000 ) ) ;
#20809=AXIS2_PLACEMENT_3D ( 'NONE', #45714, #93400, #79258 ) ;
#20829=DIRECTION ( 'NONE',  ( 0.000000000000000000, 0.000000000000000000, -1.000000000000000000 ) ) ;
#20830=CARTESIAN_POINT ( 'NONE',  ( -10.44369227015510049, 5.112964020592959180, 5.232143560358710310 ) ) ;
#20875=DIRECTION ( 'NONE',  ( 0.000000000000000000, 1.000000000000000000, 0.000000000000000000 ) ) ;
#20881=ORIENTED_EDGE ( 'NONE', *, *, #103751, .F. ) ;
#20907=EDGE_CURVE ( 'NONE', #77951, #55386, #170621, .T. ) ;
#20910=CARTESIAN_POINT ( 'NONE',  ( 8.946219267268480380, 14.55181358891489296, -7.930791147577251898 ) ) ;
#20927=EDGE_LOOP ( 'NONE', ( #137637, #58230, #5190, #199214 ) ) ;
#20931=FACE_OUTER_BOUND ( 'NONE', #23964, .T. ) ;
#20933=DIRECTION ( 'NONE',  ( 0.000000000000000000, 0.000000000000000000, 1.000000000000000000 ) ) ;
#20963=AXIS2_PLACEMENT_3D ( 'NONE', #135698, #132530, #36038 ) ;
#20993=DIRECTION ( 'NONE',  ( -0.000000000000000000, 1.000000000000000000, -0.000000000000000000 ) ) ;
#20996=PLANE ( 'NONE',  #206305 ) ;
#20997=CARTESIAN_POINT ( 'NONE',  ( -9.604686356149274573, 4.518459255872632419, 7.193747284969079558 ) ) ;
#21012=ADVANCED_FACE ( 'NONE', ( #114736 ), #98425, .F. ) ;
#21032=ORIENTED_EDGE ( 'NONE', *, *, #189421, .F. ) ;
#21046=FACE_OUTER_BOUND ( 'NONE', #168599, .T. ) ;
#21081=DIRECTION ( 'NONE',  ( 0.000000000000000000, -1.000000000000000000, 0.000000000000000000 ) ) ;
#21093=FILL_AREA_STYLE ('',( #135958 ) ) ;
#21096=VECTOR ( 'NONE', #76115, 1000.000000000000000 ) ;
#21125=UNCERTAINTY_MEASURE_WITH_UNIT (LENGTH_MEASURE( 1.000000000000000082E-05 ), #138828, 'distance_accuracy_value', 'NONE');
#21126=CARTESIAN_POINT ( 'NONE',  ( -10.62873463776380056, 11.29999999999998117, 3.199999999999997957 ) ) ;
#21153=CARTESIAN_POINT ( 'NONE',  ( -9.979842676043658045, 5.589819607760295739, 5.978770845575332338 ) ) ;
#21155=EDGE_CURVE ( 'NONE', #49028, #118348, #172523, .T. ) ;
#21173=CARTESIAN_POINT ( 'NONE',  ( -10.27770456272603461, 4.830393611244395480, 6.108565810605171897 ) ) ;
#21195=( LENGTH_UNIT ( ) NAMED_UNIT ( * ) SI_UNIT ( .MILLI., .METRE. ) );
#21198=AXIS2_PLACEMENT_3D ( 'NONE', #136303, #20388, #156823 ) ;
#21226=EDGE_CURVE ( 'NONE', #181635, #139784, #79116, .T. ) ;
#21253=EDGE_LOOP ( 'NONE', ( #177585, #92321, #90498, #136120 ) ) ;
#21255=VERTEX_POINT ( 'NONE', #156796 ) ;
#21261=CARTESIAN_POINT ( 'NONE',  ( -10.28140399934106242, 4.005782094233665269, -7.421933058660648008 ) ) ;
#21278=CARTESIAN_POINT ( 'NONE',  ( 12.00010846780092066, 6.571259622882246632, -0.4985838157269280035 ) ) ;
#21288=ORIENTED_EDGE ( 'NONE', *, *, #19563, .F. ) ;
#21290=FACE_OUTER_BOUND ( 'NONE', #155097, .T. ) ;
#21303=CARTESIAN_POINT ( 'NONE',  ( -8.171065180669568662, 15.47018273137357802, -8.834024877852263202 ) ) ;
#21308=CARTESIAN_POINT ( 'NONE',  ( 10.50000000000000000, 10.09290055818100740, 3.599999999999996536 ) ) ;
#21332=CARTESIAN_POINT ( 'NONE',  ( -15.75000000000000000, 13.40000000000000036, -3.600000000000002309 ) ) ;
#21349=MECHANICAL_DESIGN_GEOMETRIC_PRESENTATION_REPRESENTATION('',(#142334),#152961);
#21381=DIRECTION ( 'NONE',  ( 1.000000000000000000, -0.000000000000000000, -0.000000000000000000 ) ) ;
#21397=AXIS2_PLACEMENT_3D ( 'NONE', #97011, #79662, #131661 ) ;
#21413=CARTESIAN_POINT ( 'NONE',  ( 11.41381676900476805, 12.56958039977607733, 3.704697931490188889 ) ) ;
#21429=SURFACE_STYLE_FILL_AREA ( #139503 ) ;
#21450=CARTESIAN_POINT ( 'NONE',  ( -10.19171921354153554, 3.593199521514539807, -6.350946922499482561 ) ) ;
#21480=CARTESIAN_POINT ( 'NONE',  ( 9.649519181572159710, 4.269047846895349885, -7.134145857028189042 ) ) ;
#21503=CARTESIAN_POINT ( 'NONE',  ( -9.345711740228626496, 15.44303320414337222, -7.452166123625171501 ) ) ;
#21524=( BOUNDED_SURFACE ( )  B_SPLINE_SURFACE ( 3, 2, ( 
 ( #118024, #115886, #48708 ),
 ( #182951, #84390, #162460 ),
 ( #15108, #2037, #14036 ),
 ( #166714, #81197, #68107 ),
 ( #164578, #16163, #180820 ),
 ( #51902, #49760, #82248 ),
 ( #148339, #150477, #31390 ),
 ( #163521, #147275, #47659 ),
 ( #197071, #134243, #32447 ),
 ( #199179, #96410, #213307 ),
 ( #64932, #200250, #97465 ),
 ( #131082, #198128, #181871 ),
 ( #80122, #98516, #34566 ),
 ( #113770, #100637, #146227 ) ),
 .UNSPECIFIED., .F., .F., .T. ) 
 B_SPLINE_SURFACE_WITH_KNOTS ( ( 4, 2, 2, 2, 2, 2, 4 ),
 ( 3, 3 ),
 ( 5.529431079676072613E-18, 0.0003635382096235338103, 0.0007270764192470620911, 0.001090614628870590318, 0.001454152838494118761, 0.002181229257741175431, 0.002908305676988231885 ),
 ( 0.000000000000000000, 1.000000000000000000 ),
 .UNSPECIFIED. ) 
 GEOMETRIC_REPRESENTATION_ITEM ( )  RATIONAL_B_SPLINE_SURFACE ( (
 ( 1.000000000000000000, 0.8435419936913700623, 1.000000000000000000),
 ( 1.000000000000000000, 0.8440768467786702312, 1.000000000000000000),
 ( 1.000000000000000000, 0.8446657806964728010, 1.000000000000000000),
 ( 1.000000000000000000, 0.8458791039628983377, 1.000000000000000000),
 ( 1.000000000000000000, 0.8464799219268367425, 1.000000000000000000),
 ( 1.000000000000000000, 0.8478096660418573682, 1.000000000000000000),
 ( 1.000000000000000000, 0.8485318165228228349, 1.000000000000000000),
 ( 1.000000000000000000, 0.8497005200740803676, 1.000000000000000000),
 ( 1.000000000000000000, 0.8500955636246768643, 1.000000000000000000),
 ( 1.000000000000000000, 0.8503664178925908201, 1.000000000000000000),
 ( 1.000000000000000000, 0.8504660752369725962, 1.000000000000000000),
 ( 1.000000000000000000, 0.8507447348240169127, 1.000000000000000000),
 ( 1.000000000000000000, 0.8509461865225793620, 1.000000000000000000),
 ( 1.000000000000000000, 0.8509626965061065640, 1.000000000000000000) ) ) 
 REPRESENTATION_ITEM ( '' )  SURFACE ( )  );
#21537=CARTESIAN_POINT ( 'NONE',  ( 11.86239285000045918, 13.87999999999998302, 1.812080536912751283 ) ) ;
#21542=CARTESIAN_POINT ( 'NONE',  ( -9.429696025003076798, 5.003427382976973981, 6.891771494149568689 ) ) ;
#21572=ORIENTED_EDGE ( 'NONE', *, *, #12043, .T. ) ;
#21578=( NAMED_UNIT ( * ) SI_UNIT ( $, .STERADIAN. ) SOLID_ANGLE_UNIT ( ) );
#21587=VERTEX_POINT ( 'NONE', #81414 ) ;
#21590=CARTESIAN_POINT ( 'NONE',  ( -9.540655113774947793, 4.518467169708413778, -7.145788969735951568 ) ) ;
#21647=AXIS2_PLACEMENT_3D ( 'NONE', #164071, #32989, #147820 ) ;
#21651=SURFACE_STYLE_FILL_AREA ( #183122 ) ;
#21665=ORIENTED_EDGE ( 'NONE', *, *, #114498, .T. ) ;
#21685=CARTESIAN_POINT ( 'NONE',  ( -11.69053533621101160, 4.400474013969419396, 5.144636342886200531 ) ) ;
#21695=AXIS2_PLACEMENT_3D ( 'NONE', #156701, #106929, #11492 ) ;
#21715=CARTESIAN_POINT ( 'NONE',  ( -0.9738393980073648537, 15.51858052053983172, 11.99373428513897188 ) ) ;
#21717=STYLED_ITEM ( 'NONE', ( #52924 ), #77868 ) ;
#21739=CARTESIAN_POINT ( 'NONE',  ( -10.29157903258815487, 3.766103264033962450, -6.172328895365623680 ) ) ;
#21802=FILL_AREA_STYLE ('',( #171286 ) ) ;
#21822=CARTESIAN_POINT ( 'NONE',  ( -11.14389002924298566, 7.220603907090449525, 3.549113525960188031 ) ) ;
#21843=CARTESIAN_POINT ( 'NONE',  ( -10.59765138761703085, 13.79999999999998295, 3.303242380465396977 ) ) ;
#21847=ORIENTED_EDGE ( 'NONE', *, *, #168724, .T. ) ;
#21850=CARTESIAN_POINT ( 'NONE',  ( -15.75000000000000000, 9.799999999999998934, -3.200000000000001510 ) ) ;
#21876=PRESENTATION_STYLE_ASSIGNMENT (( #184399 ) ) ;
#21881=ORIENTED_EDGE ( 'NONE', *, *, #13809, .F. ) ;
#21896=DIRECTION ( 'NONE',  ( 0.1510067114093955887, -0.000000000000000000, 0.9885327375000383388 ) ) ;
#21935=CARTESIAN_POINT ( 'NONE',  ( 7.739551183390158684, 13.97472016681189189, -10.04165774006234102 ) ) ;
#21951=CARTESIAN_POINT ( 'NONE',  ( 1.500000000000053291, 7.750000000000000000, 15.74999999999999289 ) ) ;
#21953=ORIENTED_EDGE ( 'NONE', *, *, #59990, .F. ) ;
#21955=( GEOMETRIC_REPRESENTATION_CONTEXT ( 3 ) GLOBAL_UNCERTAINTY_ASSIGNED_CONTEXT ( ( #128101 ) ) GLOBAL_UNIT_ASSIGNED_CONTEXT ( ( #8072, #126185, #62179 ) ) REPRESENTATION_CONTEXT ( 'NONE', 'WORKASPACE' ) );
#21958=CIRCLE ( 'NONE', #101621, 12.00000000000000178 ) ;
#21974=EDGE_CURVE ( 'NONE', #177833, #46648, #142735, .T. ) ;
#21981=EDGE_CURVE ( 'NONE', #174627, #103981, #82774, .T. ) ;
#21986=DIRECTION ( 'NONE',  ( 1.224643483124940471E-16, 0.002327115863039739760, 0.9999972922622140103 ) ) ;
#21991=DIRECTION ( 'NONE',  ( 0.1828377250218585215, -0.9633937422820121332, -0.1960685177194217976 ) ) ;
#21992=( NAMED_UNIT ( * ) SI_UNIT ( $, .STERADIAN. ) SOLID_ANGLE_UNIT ( ) );
#21998=FACE_OUTER_BOUND ( 'NONE', #37368, .T. ) ;
#22043=CARTESIAN_POINT ( 'NONE',  ( -11.13927487678572525, 5.784125462700367315, -4.477470366402338087 ) ) ;
#22052=CARTESIAN_POINT ( 'NONE',  ( -11.45846087878769559, 11.09311600781452434, -3.566076377698187194 ) ) ;
#22058=ORIENTED_EDGE ( 'NONE', *, *, #195648, .T. ) ;
#22082=CARTESIAN_POINT ( 'NONE',  ( 0.000000000000000000, 14.48154074412737202, -12.00000000000000178 ) ) ;
#22094=DIRECTION ( 'NONE',  ( -0.000000000000000000, -1.000000000000000000, -0.000000000000000000 ) ) ;
#22104=CARTESIAN_POINT ( 'NONE',  ( -11.06955610715284166, 7.104274754441156858, 4.637919682314346481 ) ) ;
#22113=COLOUR_RGB ( '', 0.40784314, 0.44705882, 0.49803922) ;
#22143=CARTESIAN_POINT ( 'NONE',  ( 11.04536101718726293, 0.000000000000000000, 1.099999999999996758 ) ) ;
#22155=DIRECTION ( 'NONE',  ( 0.000000000000000000, 0.000000000000000000, 1.000000000000000000 ) ) ;
#22160=ORIENTED_EDGE ( 'NONE', *, *, #214308, .T. ) ;
#22164=( LENGTH_UNIT ( ) NAMED_UNIT ( * ) SI_UNIT ( .MILLI., .METRE. ) );
#22184=CARTESIAN_POINT ( 'NONE',  ( 9.262488864310135739, 13.63671387857608508, 6.830742452943137089 ) ) ;
#22194=DIRECTION ( 'NONE',  ( 0.000000000000000000, 0.1992968566527040242, 0.9799391628710180102 ) ) ;
#22219=CARTESIAN_POINT ( 'NONE',  ( -10.78237064342727791, 6.270194388237658956, -4.501389708959286473 ) ) ;
#22228=SURFACE_SIDE_STYLE ('',( #74226 ) ) ;
#22230=EDGE_CURVE ( 'NONE', #130986, #24518, #209809, .T. ) ;
#22245=ORIENTED_EDGE ( 'NONE', *, *, #57679, .F. ) ;
#22253=CARTESIAN_POINT ( 'NONE',  ( -15.75000000000000000, 13.40000000000000036, -3.200000000000001510 ) ) ;
#22259=ADVANCED_FACE ( 'NONE', ( #112398 ), #16934, .T. ) ;
#22278=DIRECTION ( 'NONE',  ( 7.993605777301127091E-15, 0.000000000000000000, 1.000000000000000000 ) ) ;
#22295=DIRECTION ( 'NONE',  ( -0.2150645590070936197, 0.8781765503997437383, 0.4272624273056206401 ) ) ;
#22330=CARTESIAN_POINT ( 'NONE',  ( -10.30104275384242740, 4.689840931292195592, -5.506867539468097483 ) ) ;
#22341=DIRECTION ( 'NONE',  ( 0.000000000000000000, -1.000000000000000000, -0.000000000000000000 ) ) ;
#22349=CARTESIAN_POINT ( 'NONE',  ( 10.88471284811786077, 8.294291839072673866, 4.944671277826161671 ) ) ;
#22361=DIRECTION ( 'NONE',  ( 0.000000000000000000, 0.000000000000000000, -1.000000000000000000 ) ) ;
#22372=CARTESIAN_POINT ( 'NONE',  ( -7.116787994678793972, 15.51980677385493124, -9.672274627470516251 ) ) ;
#22374=EDGE_LOOP ( 'NONE', ( #47204, #11456 ) ) ;
#22375=ADVANCED_FACE ( 'NONE', ( #32146 ), #182852, .F. ) ;
#22421=CARTESIAN_POINT ( 'NONE',  ( -11.60136562008509387, 4.149718911762417584, -5.313756115068398067 ) ) ;
#22427=VERTEX_POINT ( 'NONE', #177338 ) ;
#22437=ORIENTED_EDGE ( 'NONE', *, *, #152281, .F. ) ;
#22522=PRESENTATION_STYLE_ASSIGNMENT (( #70201 ) ) ;
#22538=CARTESIAN_POINT ( 'NONE',  ( 9.355700869302610911, 13.88187516316259895, -7.515225910968625023 ) ) ;
#22573=CARTESIAN_POINT ( 'NONE',  ( -11.84668730067608600, 10.19999999999998153, 1.399999999999998579 ) ) ;
#22607=CARTESIAN_POINT ( 'NONE',  ( -11.89839339040395139, 9.771225315960876401, 1.560885614203548100 ) ) ;
#22622=CARTESIAN_POINT ( 'NONE',  ( -10.81659190237994395, 5.544392656652913587, 6.534142543513654644 ) ) ;
#22628=FACE_OUTER_BOUND ( 'NONE', #194163, .T. ) ;
#22650=CARTESIAN_POINT ( 'NONE',  ( -9.086228366407658186, 14.48154074263858604, 7.851304407759048587 ) ) ;
#22658=CARTESIAN_POINT ( 'NONE',  ( 10.56514123924917392, 9.841080455211937306, -3.404988257269842222 ) ) ;
#22668=DIRECTION ( 'NONE',  ( -0.000000000000000000, -1.000000000000000000, 0.000000000000000000 ) ) ;
#22686=CARTESIAN_POINT ( 'NONE',  ( -11.89942855770814134, 11.29999999999999893, 0.6999999999999992895 ) ) ;
#22717=CARTESIAN_POINT ( 'NONE',  ( -4.750201942159842261, 15.44698457193027785, 10.98078241047744186 ) ) ;
#22726=CARTESIAN_POINT ( 'NONE',  ( -11.78331023100045627, 12.21999999999998288, 1.799999999999999600 ) ) ;
#22750=FILL_AREA_STYLE_COLOUR ( '', #185503 ) ;
#22761=CARTESIAN_POINT ( 'NONE',  ( -9.569358774149643310, 3.553052365627049625, 7.167287524840453727 ) ) ;
#22762=CARTESIAN_POINT ( 'NONE',  ( -10.96276904610368597, 4.385383195573210102, 6.374211443005175504 ) ) ;
#22794=EDGE_CURVE ( 'NONE', #117081, #56620, #133947, .T. ) ;
#22818=CARTESIAN_POINT ( 'NONE',  ( -11.35605497252127094, 9.985818540483544226, -3.553547709190210124 ) ) ;
#22848=VECTOR ( 'NONE', #31488, 1000.000000000000000 ) ;
#22858=AXIS2_PLACEMENT_3D ( 'NONE', #5638, #25119, #202787 ) ;
#22863=FACE_BOUND ( 'NONE', #69702, .T. ) ;
#22884=DIRECTION ( 'NONE',  ( 0.000000000000000000, 0.4225363771131893098, 0.9063459659622591369 ) ) ;
#22885=ORIENTED_EDGE ( 'NONE', *, *, #144093, .T. ) ;
#22899=CARTESIAN_POINT ( 'NONE',  ( -11.37834099079384487, 6.126291437673294205, 3.408052918099385931 ) ) ;
#22912=CARTESIAN_POINT ( 'NONE',  ( 11.94651559118242190, 12.44869344121029009, 1.135242698369639980 ) ) ;
#22918=DIRECTION ( 'NONE',  ( 1.000000000000000000, -0.000000000000000000, -0.000000000000000000 ) ) ;
#22937=EDGE_CURVE ( 'NONE', #174805, #131565, #116647, .T. ) ;
#22947=ADVANCED_FACE ( 'NONE', ( #199955 ), #53723, .F. ) ;
#22959=ORIENTED_EDGE ( 'NONE', *, *, #110772, .T. ) ;
#22965=CARTESIAN_POINT ( 'NONE',  ( -1.249999999999964695, 8.500000000000000000, -10.97907099895069294 ) ) ;
#22986=SURFACE_STYLE_USAGE ( .BOTH. , #27269 ) ;
#22994=CARTESIAN_POINT ( 'NONE',  ( -11.89942855770813956, 12.22000000000000064, -0.7000000000000009548 ) ) ;
#23010=ORIENTED_EDGE ( 'NONE', *, *, #135967, .T. ) ;
#23023=UNCERTAINTY_MEASURE_WITH_UNIT (LENGTH_MEASURE( 1.000000000000000082E-05 ), #88293, 'distance_accuracy_value', 'NONE');
#23071=CARTESIAN_POINT ( 'NONE',  ( 10.50000000000000178, 0.000000000000000000, -3.600000000000002309 ) ) ;
#23105=STYLED_ITEM ( 'NONE', ( #52011 ), #197622 ) ;
#23120=CARTESIAN_POINT ( 'NONE',  ( -11.89942855770813956, 12.30000000000000071, 0.6999999999999992895 ) ) ;
#23138=EDGE_CURVE ( 'NONE', #168364, #78193, #214187, .T. ) ;
#23143=ADVANCED_FACE ( 'NONE', ( #73146 ), #201678, .T. ) ;
#23152=VERTEX_POINT ( 'NONE', #82762 ) ;
#23157=EDGE_CURVE ( 'NONE', #14896, #157191, #75824, .T. ) ;
#23163=CARTESIAN_POINT ( 'NONE',  ( -8.150368799117956087, 14.48038083418904698, -8.818837747985245556 ) ) ;
#23184=CARTESIAN_POINT ( 'NONE',  ( -15.75000000000000000, 10.89999999999998259, 1.399999999999998579 ) ) ;
#23193=( BOUNDED_CURVE ( )  B_SPLINE_CURVE ( 3, ( #6321, #138495, #201314, #106034 ),
 .UNSPECIFIED., .F., .T. ) 
 B_SPLINE_CURVE_WITH_KNOTS ( ( 4, 4 ),
 ( 1.430804639040423654, 1.438015327900961982 ),
 .UNSPECIFIED. ) 
 CURVE ( )  GEOMETRIC_REPRESENTATION_ITEM ( )  RATIONAL_B_SPLINE_CURVE ( ( 1.000000000000000000, 0.9999956671685397147, 0.9999956671685397147, 1.000000000000000000 ) ) 
 REPRESENTATION_ITEM ( '' )  );
#23212=CYLINDRICAL_SURFACE ( 'NONE', #175138, 0.08000000000000020983 ) ;
#23219=CARTESIAN_POINT ( 'NONE',  ( -10.62873463776380056, 11.29999999999999893, -3.200000000000001510 ) ) ;
#23221=( BOUNDED_SURFACE ( )  B_SPLINE_SURFACE ( 3, 2, ( 
 ( #199504, #51147, #117271 ),
 ( #184326, #19698, #189667 ),
 ( #106347, #25031, #172369 ),
 ( #39164, #42388, #59671 ),
 ( #7706, #91131, #107426 ),
 ( #143105, #76979, #23959 ) ),
 .UNSPECIFIED., .F., .F., .F. ) 
 B_SPLINE_SURFACE_WITH_KNOTS ( ( 4, 2, 4 ),
 ( 3, 3 ),
 ( 0.000000000000000000, 0.0003831327362561333209, 0.0007662654725122666419 ),
 ( 0.000000000000000000, 1.000000000000000000 ),
 .UNSPECIFIED. ) 
 GEOMETRIC_REPRESENTATION_ITEM ( )  RATIONAL_B_SPLINE_SURFACE ( (
 ( 1.000000000000000000, 0.5879095031487548972, 1.000000000000000000),
 ( 1.000000000000000000, 0.5873691247580630215, 1.000000000000000000),
 ( 1.000000000000000000, 0.6054349545494872586, 1.000000000000000000),
 ( 1.000000000000000000, 0.6533334602768978705, 1.000000000000000000),
 ( 1.000000000000000000, 0.6828746263149312323, 1.000000000000000000),
 ( 1.000000000000000000, 0.7071067811865475727, 1.000000000000000000) ) ) 
 REPRESENTATION_ITEM ( '' )  SURFACE ( )  );
#23243=ORIENTED_EDGE ( 'NONE', *, *, #127684, .T. ) ;
#23247=CARTESIAN_POINT ( 'NONE',  ( -11.33772463945037146, 10.89999999999998259, 3.599999999999999201 ) ) ;
#23257=CARTESIAN_POINT ( 'NONE',  ( 9.412584077552686779, 11.54679772643938307, 7.460083846873735602 ) ) ;
#23262=CARTESIAN_POINT ( 'NONE',  ( 8.305220197644215929, 14.86737089724833893, -9.585679967850639471 ) ) ;
#23264=CARTESIAN_POINT ( 'NONE',  ( 9.216403166322994167, 13.91905933883010249, 6.904314279704210300 ) ) ;
#23272=UNCERTAINTY_MEASURE_WITH_UNIT (LENGTH_MEASURE( 1.000000000000000082E-05 ), #80900, 'distance_accuracy_value', 'NONE');
#23285=DIRECTION ( 'NONE',  ( 0.000000000000000000, 1.000000000000000000, 0.000000000000000000 ) ) ;
#23300=CARTESIAN_POINT ( 'NONE',  ( -10.85762644215163775, 5.701980886241464042, -6.452002860825420960 ) ) ;
#23309=PRESENTATION_STYLE_ASSIGNMENT (( #55831 ) ) ;
#23312=AXIS2_PLACEMENT_3D ( 'NONE', #29126, #129909, #179649 ) ;
#23340=FACE_BOUND ( 'NONE', #173290, .T. ) ;
#23372=ORIENTED_EDGE ( 'NONE', *, *, #33483, .T. ) ;
#23408=( GEOMETRIC_REPRESENTATION_CONTEXT ( 3 ) GLOBAL_UNCERTAINTY_ASSIGNED_CONTEXT ( ( #183658 ) ) GLOBAL_UNIT_ASSIGNED_CONTEXT ( ( #205447, #70095, #204360 ) ) REPRESENTATION_CONTEXT ( 'NONE', 'WORKASPACE' ) );
#23419=CARTESIAN_POINT ( 'NONE',  ( -11.24554764128284035, 7.016280722987462859, -5.611469924715791535 ) ) ;
#23425=CARTESIAN_POINT ( 'NONE',  ( 8.790098660144254339, 13.29414747594431923, 8.101455065885637907 ) ) ;
#23427=ORIENTED_EDGE ( 'NONE', *, *, #93121, .F. ) ;
#23449=AXIS2_PLACEMENT_3D ( 'NONE', #61813, #127981, #193934 ) ;
#23462=CARTESIAN_POINT ( 'NONE',  ( -15.75000000000000000, 13.39999999999998259, 1.399999999999998579 ) ) ;
#23468=EDGE_CURVE ( 'NONE', #76787, #29424, #13554, .T. ) ;
#23499=CARTESIAN_POINT ( 'NONE',  ( -9.917242840447775265, 4.174869238508773783, -6.172972641688763140 ) ) ;
#23505=VERTEX_POINT ( 'NONE', #107621 ) ;
#23509=CARTESIAN_POINT ( 'NONE',  ( 11.48243876534946217, 11.29999999999998117, 3.199999999999997957 ) ) ;
#23547=EDGE_CURVE ( 'NONE', #182455, #155586, #17079, .T. ) ;
#23554=ORIENTED_EDGE ( 'NONE', *, *, #196415, .F. ) ;
#23586=ORIENTED_EDGE ( 'NONE', *, *, #50194, .T. ) ;
#23589=( LENGTH_UNIT ( ) NAMED_UNIT ( * ) SI_UNIT ( .MILLI., .METRE. ) );
#23598=FILL_AREA_STYLE_COLOUR ( '', #192762 ) ;
#23616=CARTESIAN_POINT ( 'NONE',  ( 11.41381675112453387, 13.39999999999998259, 3.704697986577180746 ) ) ;
#23618=CARTESIAN_POINT ( 'NONE',  ( 11.48243876534946217, 12.30000000000000071, -3.200000000000001510 ) ) ;
#23629=PRESENTATION_STYLE_ASSIGNMENT (( #188265 ) ) ;
#23649=CARTESIAN_POINT ( 'NONE',  ( -11.80248046418316044, 9.799999999999982947, 1.695421849633139466 ) ) ;
#23661=CARTESIAN_POINT ( 'NONE',  ( 0.000000000000000000, 12.30000000000000071, 0.000000000000000000 ) ) ;
#23671=DIRECTION ( 'NONE',  ( 0.000000000000000000, 0.000000000000000000, 1.000000000000000000 ) ) ;
#23674=DIRECTION ( 'NONE',  ( 0.000000000000000000, -1.000000000000000000, -1.804652791718263484E-16 ) ) ;
#23681=EDGE_CURVE ( 'NONE', #83914, #204424, #109762, .T. ) ;
#23682=CARTESIAN_POINT ( 'NONE',  ( 11.43204722947019825, 13.65592754026173594, -3.649275849833183649 ) ) ;
#23699=CARTESIAN_POINT ( 'NONE',  ( 0.008622031262369225790, 14.55347103577515000, 11.95585889282743253 ) ) ;
#23701=CARTESIAN_POINT ( 'NONE',  ( -10.97061778408437505, 3.255139717175850933, 6.407648009301818881 ) ) ;
#23730=CARTESIAN_POINT ( 'NONE',  ( -7.116787983951523344, 15.51980677384556984, -9.672274635395138986 ) ) ;
#23738=PLANE ( 'NONE',  #185521 ) ;
#23797=CARTESIAN_POINT ( 'NONE',  ( -7.105996805615566458, 15.47012406969961518, 9.680156245089420963 ) ) ;
#23811=VECTOR ( 'NONE', #173429, 1000.000000000000000 ) ;
#23812=CARTESIAN_POINT ( 'NONE',  ( 0.000000000000000000, 11.29999999999999893, 0.000000000000000000 ) ) ;
#23833=CYLINDRICAL_SURFACE ( 'NONE', #150451, 0.3999999999999997446 ) ;
#23841=CARTESIAN_POINT ( 'NONE',  ( -11.30310531956832598, 5.150576456239967627, 5.742040133384030298 ) ) ;
#23842=ORIENTED_EDGE ( 'NONE', *, *, #214308, .F. ) ;
#23850=ORIENTED_EDGE ( 'NONE', *, *, #121129, .T. ) ;
#23869=EDGE_CURVE ( 'NONE', #198793, #28237, #30901, .T. ) ;
#23878=LINE ( 'NONE', #140886, #202616 ) ;
#23881=CARTESIAN_POINT ( 'NONE',  ( 11.97929049433705551, 13.80000000000000071, 0.7046979865771805240 ) ) ;
#23891=CARTESIAN_POINT ( 'NONE',  ( -8.148189797612232610, 14.48010055955566244, 8.855677698438045198 ) ) ;
#23903=VECTOR ( 'NONE', #134997, 1000.000000000000000 ) ;
#23923=CARTESIAN_POINT ( 'NONE',  ( 11.86239285000045918, 11.29999999999998472, 1.812080536912751283 ) ) ;
#23957=DIRECTION ( 'NONE',  ( 0.5773487058764860125, 0.002327115863041261980, 0.8164943700690817652 ) ) ;
#23959=CARTESIAN_POINT ( 'NONE',  ( 11.55950211276791428, 9.719999999999998863, -3.221476510067115662 ) ) ;
#23964=EDGE_LOOP ( 'NONE', ( #87412, #197204, #57427, #3292 ) ) ;
#23978=CARTESIAN_POINT ( 'NONE',  ( -10.93359526636954193, 4.740328704497578372, 4.433404364989353752 ) ) ;
#23980=CARTESIAN_POINT ( 'NONE',  ( 9.672792005750940447, 13.47495944640959920, 8.176450814826708324 ) ) ;
#23985=CARTESIAN_POINT ( 'NONE',  ( 11.86686399458719521, 12.49071270224662555, -1.056461745586973588 ) ) ;
#24032=DIRECTION ( 'NONE',  ( 0.000000000000000000, 0.000000000000000000, 1.000000000000000000 ) ) ;
#24073=( GEOMETRIC_REPRESENTATION_CONTEXT ( 3 ) GLOBAL_UNCERTAINTY_ASSIGNED_CONTEXT ( ( #211888 ) ) GLOBAL_UNIT_ASSIGNED_CONTEXT ( ( #161440, #47699, #27148 ) ) REPRESENTATION_CONTEXT ( 'NONE', 'WORKASPACE' ) );
#24088=CARTESIAN_POINT ( 'NONE',  ( 7.501149153046521967, 15.44179335589286062, 9.372933691065389539 ) ) ;
#24091=FACE_OUTER_BOUND ( 'NONE', #120558, .T. ) ;
#24092=DIRECTION ( 'NONE',  ( -0.000000000000000000, 1.000000000000000000, 9.023263958591317418E-17 ) ) ;
#24096=ADVANCED_BREP_SHAPE_REPRESENTATION ( '', ( #20283, #19400, #200407 ), #110829 ) ;
#24132=CARTESIAN_POINT ( 'NONE',  ( -10.79305576557562318, 4.699117409047659955, 5.142361589734059990 ) ) ;
#24148=CARTESIAN_POINT ( 'NONE',  ( -8.165975823559877611, 14.52981782405839262, -8.838012710010978878 ) ) ;
#24156=ORIENTED_EDGE ( 'NONE', *, *, #88143, .F. ) ;
#24176=ADVANCED_FACE ( 'NONE', ( #85975 ), #121098, .F. ) ;
#24191=CARTESIAN_POINT ( 'NONE',  ( -11.97929049433705551, 12.30000000000000071, 0.7046979865771804130 ) ) ;
#24208=SURFACE_STYLE_FILL_AREA ( #58866 ) ;
#24229=CARTESIAN_POINT ( 'NONE',  ( 11.38290105699531196, 7.490053980982428250, 5.034049216093361423 ) ) ;
#24233=CARTESIAN_POINT ( 'NONE',  ( -11.41126283316785361, 9.841253930915410564, -3.405403429622882783 ) ) ;
#24243=ORIENTED_EDGE ( 'NONE', *, *, #58229, .F. ) ;
#24255=DIRECTION ( 'NONE',  ( -0.000000000000000000, 0.000000000000000000, -1.000000000000000000 ) ) ;
#24258=DIRECTION ( 'NONE',  ( 0.000000000000000000, -1.000000000000000000, 0.000000000000000000 ) ) ;
#24263=B_SPLINE_CURVE_WITH_KNOTS ( 'NONE', 3,
 ( #198987, #65778, #101517, #52765, #97275, #50632 ),
 .UNSPECIFIED., .F., .F.,
 ( 4, 2, 4 ),
 ( 0.000000000000000000, 0.0003168911866439334617, 0.0006337823732878669234 ),
 .UNSPECIFIED. ) ;
#24284=CARTESIAN_POINT ( 'NONE',  ( 0.7124089920922619390, 15.00000000000000355, 12.66466791154580207 ) ) ;
#24290=DIRECTION ( 'NONE',  ( 0.000000000000000000, -1.000000000000000000, 0.000000000000000000 ) ) ;
#24326=CARTESIAN_POINT ( 'NONE',  ( 6.928203230275520319, 15.00000000000000000, 9.797958971132713302 ) ) ;
#24333=CARTESIAN_POINT ( 'NONE',  ( 9.644012019580303630, 13.59213021077435535, 8.211487644058824031 ) ) ;
#24365=CARTESIAN_POINT ( 'NONE',  ( -10.84554942614793127, 5.653270432668692891, -6.476099931950408006 ) ) ;
#24376=EDGE_CURVE ( 'NONE', #61984, #18470, #4822, .T. ) ;
#24390=VERTEX_POINT ( 'NONE', #116400 ) ;
#24392=CARTESIAN_POINT ( 'NONE',  ( 9.817133948775492058, 11.89457090661458238, 6.904171386027695867 ) ) ;
#24402=CARTESIAN_POINT ( 'NONE',  ( 0.000000000000000000, 8.500000000000000000, 0.000000000000000000 ) ) ;
#24428=CARTESIAN_POINT ( 'NONE',  ( -15.75000000000000000, 9.799999999999998934, -3.200000000000001510 ) ) ;
#24430=PLANE ( 'NONE',  #27052 ) ;
#24444=CARTESIAN_POINT ( 'NONE',  ( -9.356506676016463686, 14.56575457568656340, -7.432410969268996581 ) ) ;
#24461=ORIENTED_EDGE ( 'NONE', *, *, #88143, .T. ) ;
#24462=VECTOR ( 'NONE', #57227, 1000.000000000000000 ) ;
#24485=CARTESIAN_POINT ( 'NONE',  ( -9.979823206198361163, 5.589814398814587193, -5.978750339097102184 ) ) ;
#24492=CARTESIAN_POINT ( 'NONE',  ( 8.208643724399392383, 14.14623621761441363, 8.753817594573789052 ) ) ;
#24504=ORIENTED_EDGE ( 'NONE', *, *, #195285, .F. ) ;
#24515=CARTESIAN_POINT ( 'NONE',  ( -11.43204722947019825, 11.15592754026171463, 3.649275849833181429 ) ) ;
#24518=VERTEX_POINT ( 'NONE', #183465 ) ;
#24524=VECTOR ( 'NONE', #74998, 1000.000000000000000 ) ;
#24560=PRESENTATION_STYLE_ASSIGNMENT (( #39766 ) ) ;
#24565=CARTESIAN_POINT ( 'NONE',  ( -9.813523197712067159, 5.212597839642568509, -6.298667959258508198 ) ) ;
#24591=( NAMED_UNIT ( * ) SI_UNIT ( $, .STERADIAN. ) SOLID_ANGLE_UNIT ( ) );
#24621=AXIS2_PLACEMENT_3D ( 'NONE', #104067, #121462, #187432 ) ;
#24638=CARTESIAN_POINT ( 'NONE',  ( 0.000000000000000000, 4.446955548196618757, 0.000000000000000000 ) ) ;
#24643=ORIENTED_EDGE ( 'NONE', *, *, #61688, .T. ) ;
#24656=FILL_AREA_STYLE_COLOUR ( '', #47616 ) ;
#24660=ORIENTED_EDGE ( 'NONE', *, *, #21981, .F. ) ;
#24682=CARTESIAN_POINT ( 'NONE',  ( 8.397938042107668366, 15.16470181921706306, -8.573252516252733102 ) ) ;
#24684=DIRECTION ( 'NONE',  ( 0.000000000000000000, -1.000000000000000000, 0.000000000000000000 ) ) ;
#24695=CARTESIAN_POINT ( 'NONE',  ( 11.41381675112459959, 10.19999999999997087, 3.704697986577257129 ) ) ;
#24698=EDGE_CURVE ( 'NONE', #93151, #94599, #210836, .T. ) ;
#24726=DIRECTION ( 'NONE',  ( 0.000000000000000000, 1.000000000000000000, 0.000000000000000000 ) ) ;
#24727=CARTESIAN_POINT ( 'NONE',  ( -9.333041836226904309, 15.44694763438996077, -7.472413793095822321 ) ) ;
#24731=TOROIDAL_SURFACE ( 'NONE', #204683, 11.92000000000000171, 0.08000000000000000167 ) ;
#24739=FILL_AREA_STYLE_COLOUR ( '', #177964 ) ;
#24750=CARTESIAN_POINT ( 'NONE',  ( -11.92619526248521034, 10.07255386085831894, 1.328859120100916558 ) ) ;
#24765=CARTESIAN_POINT ( 'NONE',  ( -11.97929049433705551, 13.88000000000000078, 0.7046979865771804130 ) ) ;
#24766=CARTESIAN_POINT ( 'NONE',  ( -10.32184838934336213, 3.007359993651753438, 7.367400555339857604 ) ) ;
#24772=AXIS2_PLACEMENT_3D ( 'NONE', #154002, #122660, #74882 ) ;
#24803=CARTESIAN_POINT ( 'NONE',  ( 11.86239285000045740, 11.37999999999998302, 1.812080536912751061 ) ) ;
#24813=EDGE_CURVE ( 'NONE', #57689, #142717, #48371, .T. ) ;
#24819=CARTESIAN_POINT ( 'NONE',  ( -5.580332384298489323, 14.55306937873557338, 10.58301128396242419 ) ) ;
#24821=FILL_AREA_STYLE ('',( #8576 ) ) ;
#24860=AXIS2_PLACEMENT_3D ( 'NONE', #182044, #32614, #152764 ) ;
#24863=LINE ( 'NONE', #72546, #184406 ) ;
#24872=ORIENTED_EDGE ( 'NONE', *, *, #12835, .F. ) ;
#24875=FILL_AREA_STYLE ('',( #9698 ) ) ;
#24897=( NAMED_UNIT ( * ) SI_UNIT ( $, .STERADIAN. ) SOLID_ANGLE_UNIT ( ) );
#24908=CARTESIAN_POINT ( 'NONE',  ( -11.19490907666120272, 4.805655862119510680, 5.952061394947645745 ) ) ;
#24926=( NAMED_UNIT ( * ) SI_UNIT ( $, .STERADIAN. ) SOLID_ANGLE_UNIT ( ) );
#24953=CARTESIAN_POINT ( 'NONE',  ( 11.86145016429273191, 13.40000000000000036, 1.099999999999996980 ) ) ;
#24963=CARTESIAN_POINT ( 'NONE',  ( -5.940857138655644576, 14.48120657956202351, 10.43616353783158957 ) ) ;
#24970=DIRECTION ( 'NONE',  ( 0.9982742078614211811, 0.000000000000000000, -0.05872483221476467591 ) ) ;
#24999=STYLED_ITEM ( 'NONE', ( #113199 ), #76119 ) ;
#25028=STYLED_ITEM ( 'NONE', ( #212408 ), #175193 ) ;
#25031=CARTESIAN_POINT ( 'NONE',  ( 11.45846087878779329, 10.00688399218553570, -3.566076377698155664 ) ) ;
#25038=ORIENTED_EDGE ( 'NONE', *, *, #101745, .T. ) ;
#25059=DIRECTION ( 'NONE',  ( 0.8164965809277251463, 0.000000000000000000, 0.5773502691896270633 ) ) ;
#25078=CARTESIAN_POINT ( 'NONE',  ( -10.56511880488638333, 12.34113476418481170, -3.405056808716381944 ) ) ;
#25088=EDGE_CURVE ( 'NONE', #93416, #139784, #123908, .T. ) ;
#25097=CARTESIAN_POINT ( 'NONE',  ( 6.902720145097993587, 14.55347103577521217, 9.761920446463554057 ) ) ;
#25102=CARTESIAN_POINT ( 'NONE',  ( -15.75000000000000000, 12.69999999999999929, -3.200000000000001510 ) ) ;
#25119=DIRECTION ( 'NONE',  ( -0.2684563758389304500, -0.000000000000000000, -0.9632918427306581544 ) ) ;
#25162=ORIENTED_EDGE ( 'NONE', *, *, #134538, .T. ) ;
#25166=( LENGTH_UNIT ( ) NAMED_UNIT ( * ) SI_UNIT ( .MILLI., .METRE. ) );
#25174=ORIENTED_EDGE ( 'NONE', *, *, #198514, .T. ) ;
#25223=CARTESIAN_POINT ( 'NONE',  ( -10.60630082101195804, 5.715768461961713953, -4.896526734066639186 ) ) ;
#25235=ORIENTED_EDGE ( 'NONE', *, *, #131603, .T. ) ;
#25237=CIRCLE ( 'NONE', #135944, 0.5000000000000013323 ) ;
#25255=CARTESIAN_POINT ( 'NONE',  ( -1.249999999999964695, 8.500000000000000000, 11.02939254900287303 ) ) ;
#25266=CARTESIAN_POINT ( 'NONE',  ( -1.499999999999946709, 7.750000000000000000, 15.75000000000000711 ) ) ;
#25275=CARTESIAN_POINT ( 'NONE',  ( -11.89197816957260123, 12.30000000000000071, 0.8055420615339489165 ) ) ;
#25288=ORIENTED_EDGE ( 'NONE', *, *, #139797, .T. ) ;
#25291=VERTEX_POINT ( 'NONE', #160054 ) ;
#25296=EDGE_LOOP ( 'NONE', ( #55223, #94245, #153883, #175868 ) ) ;
#25313=CARTESIAN_POINT ( 'NONE',  ( 10.24318454578369852, 9.275991984790607603, -5.779941430892880483 ) ) ;
#25317=CARTESIAN_POINT ( 'NONE',  ( -11.52483635780544624, 9.720000086424647634, -3.345866325258088914 ) ) ;
#25319=ORIENTED_EDGE ( 'NONE', *, *, #47376, .F. ) ;
#25328=AXIS2_PLACEMENT_3D ( 'NONE', #121110, #73320, #158859 ) ;
#25330=CARTESIAN_POINT ( 'NONE',  ( 9.444297818689598500, 3.530917896769790065, -7.404075800243193228 ) ) ;
#25342=ADVANCED_FACE ( 'NONE', ( #143853 ), #205587, .F. ) ;
#25362=( BOUNDED_SURFACE ( )  B_SPLINE_SURFACE ( 3, 2, ( 
 ( #156128, #73793, #139888 ),
 ( #140974, #74868, #126900 ),
 ( #27168, #159307, #91134 ),
 ( #161461, #125832, #124767 ),
 ( #129032, #174523, #45581 ),
 ( #206983, #58612, #190727 ) ),
 .UNSPECIFIED., .F., .F., .T. ) 
 B_SPLINE_SURFACE_WITH_KNOTS ( ( 4, 2, 4 ),
 ( 3, 3 ),
 ( 0.000000000000000000, 0.0003766405729503173702, 0.0007532811459006347405 ),
 ( 0.000000000000000000, 1.000000000000000000 ),
 .UNSPECIFIED. ) 
 GEOMETRIC_REPRESENTATION_ITEM ( )  RATIONAL_B_SPLINE_SURFACE ( (
 ( 1.000000000000000000, 0.7071067811865474617, 1.000000000000000000),
 ( 1.000000000000000000, 0.7211294902955810437, 1.000000000000000000),
 ( 1.000000000000000000, 0.7311181975227820651, 1.000000000000000000),
 ( 1.000000000000000000, 0.7429553055063957689, 1.000000000000000000),
 ( 1.000000000000000000, 0.7451698531056420993, 1.000000000000000000),
 ( 1.000000000000000000, 0.7452309222762957264, 1.000000000000000000) ) ) 
 REPRESENTATION_ITEM ( '' )  SURFACE ( )  );
#25367=DIRECTION ( 'NONE',  ( -0.000000000000000000, -1.000000000000000000, -0.000000000000000000 ) ) ;
#25370=CARTESIAN_POINT ( 'NONE',  ( -1.878313713276878127, 14.99999999999692157, 12.68000002627078082 ) ) ;
#25416=CARTESIAN_POINT ( 'NONE',  ( 8.542663007067599068, 15.39167316688947018, 7.880542118333895729 ) ) ;
#25448=CARTESIAN_POINT ( 'NONE',  ( -12.00288634729131232, 5.507422065878898820, 4.496070577805427959 ) ) ;
#25450=VECTOR ( 'NONE', #147537, 1000.000000000000000 ) ;
#25471=EDGE_LOOP ( 'NONE', ( #210146, #172802, #118346, #135873 ) ) ;
#25478=CARTESIAN_POINT ( 'NONE',  ( 10.26598409777793464, 10.85580239508950307, 6.219453420784894604 ) ) ;
#25480=EDGE_CURVE ( 'NONE', #132967, #180190, #165376, .T. ) ;
#25534=CARTESIAN_POINT ( 'NONE',  ( 11.94105721237522921, 11.02740390989733044, 1.187919463087248273 ) ) ;
#25555=CARTESIAN_POINT ( 'NONE',  ( -9.645406396194509568, 4.042443384815813445, -6.587269312116742270 ) ) ;
#25565=CARTESIAN_POINT ( 'NONE',  ( -10.84558554699185784, 5.653278704827924273, 6.476092148523931336 ) ) ;
#25606=FACE_OUTER_BOUND ( 'NONE', #54529, .T. ) ;
#25636=CARTESIAN_POINT ( 'NONE',  ( -11.73097396203126763, 4.534521666694462105, -5.066462175338618756 ) ) ;
#25664=EDGE_CURVE ( 'NONE', #137788, #204338, #113506, .T. ) ;
#25704=CARTESIAN_POINT ( 'NONE',  ( 11.08642519832315543, 7.950771188443131798, 4.613362863501950351 ) ) ;
#25720=ORIENTED_EDGE ( 'NONE', *, *, #151802, .F. ) ;
#25728=CARTESIAN_POINT ( 'NONE',  ( 11.89942855770813956, 9.719999999999998863, -0.7000000000000009548 ) ) ;
#25745=ORIENTED_EDGE ( 'NONE', *, *, #151879, .F. ) ;
#25776=AXIS2_PLACEMENT_3D ( 'NONE', #124553, #25879, #75712 ) ;
#25793=AXIS2_PLACEMENT_3D ( 'NONE', #106055, #7412, #23671 ) ;
#25830=FACE_OUTER_BOUND ( 'NONE', #14130, .T. ) ;
#25831=CARTESIAN_POINT ( 'NONE',  ( -11.55001508359621987, 4.031797291955615314, 5.408777164504234847 ) ) ;
#25874=VECTOR ( 'NONE', #170169, 1000.000000000000000 ) ;
#25879=DIRECTION ( 'NONE',  ( 0.000000000000000000, -1.000000000000000000, -1.804652791718263484E-16 ) ) ;
#25880=CARTESIAN_POINT ( 'NONE',  ( -11.07131503167114772, 12.30000000000000071, 0.8043049353970799231 ) ) ;
#25886=CARTESIAN_POINT ( 'NONE',  ( 10.62873463776380056, 11.29999999999999893, -3.200000000000001510 ) ) ;
#25890=SURFACE_STYLE_FILL_AREA ( #11773 ) ;
#25895=CIRCLE ( 'NONE', #174689, 0.08000000000000040412 ) ;
#25896=FACE_OUTER_BOUND ( 'NONE', #182085, .T. ) ;
#25899=FACE_OUTER_BOUND ( 'NONE', #53283, .T. ) ;
#25903=EDGE_LOOP ( 'NONE', ( #170392, #57169, #22058, #203320 ) ) ;
#25910=B_SPLINE_CURVE_WITH_KNOTS ( 'NONE', 3,
 ( #76817, #157031, #141873, #140804, #58449, #62696 ),
 .UNSPECIFIED., .F., .F.,
 ( 4, 2, 4 ),
 ( 0.000000000000000000, 0.0003778774010236166992, 0.0007557548020472333985 ),
 .UNSPECIFIED. ) ;
#25932=CARTESIAN_POINT ( 'NONE',  ( 11.01135777277262306, 13.40000000000000036, -1.400000000000001910 ) ) ;
#25945=PRESENTATION_STYLE_ASSIGNMENT (( #206827 ) ) ;
#25946=CARTESIAN_POINT ( 'NONE',  ( -11.00592705432737972, 9.989806926531038300, 1.444010445236424856 ) ) ;
#25947=CARTESIAN_POINT ( 'NONE',  ( 11.57874831553684380, 8.190333010158946436, -2.985585545478492975 ) ) ;
#25955=COLOUR_RGB ( '', 0.72549020, 0.75294118, 0.79215686) ;
#25979=ORIENTED_EDGE ( 'NONE', *, *, #71412, .T. ) ;
#25996=ORIENTED_EDGE ( 'NONE', *, *, #23468, .T. ) ;
#26027=CARTESIAN_POINT ( 'NONE',  ( -4.723283533108845411, 14.53085706694251478, 11.04060857866791956 ) ) ;
#26030=CARTESIAN_POINT ( 'NONE',  ( -11.41176686791169104, 9.840491965131459295, -3.404018756831829418 ) ) ;
#26065=ORIENTED_EDGE ( 'NONE', *, *, #89674, .F. ) ;
#26095=CARTESIAN_POINT ( 'NONE',  ( -15.75000000000000000, 13.40000000000000036, -1.100000000000002087 ) ) ;
#26097=CARTESIAN_POINT ( 'NONE',  ( -11.84668730067608777, 10.09365272245204714, -1.400000000000002132 ) ) ;
#26103=AXIS2_PLACEMENT_3D ( 'NONE', #216, #98839, #95661 ) ;
#26115=CARTESIAN_POINT ( 'NONE',  ( -10.84253909858433218, 4.919570308430900596, -5.035411995924089723 ) ) ;
#26118=CARTESIAN_POINT ( 'NONE',  ( -11.55950211276791251, 9.799999999999982947, 3.221476510067111665 ) ) ;
#26137=ORIENTED_EDGE ( 'NONE', *, *, #210187, .F. ) ;
#26142=CARTESIAN_POINT ( 'NONE',  ( -11.35573736746281348, 13.61270414413282204, -3.554362808847921773 ) ) ;
#26178=ORIENTED_EDGE ( 'NONE', *, *, #94349, .T. ) ;
#26183=CARTESIAN_POINT ( 'NONE',  ( -11.97181073603049661, 12.22000000000000064, 0.8318477717169575625 ) ) ;
#26212=FILL_AREA_STYLE_COLOUR ( '', #35211 ) ;
#26217=AXIS2_PLACEMENT_3D ( 'NONE', #195633, #31009, #163136 ) ;
#26218=EDGE_LOOP ( 'NONE', ( #51288, #181700, #30938, #61134 ) ) ;
#26226=CARTESIAN_POINT ( 'NONE',  ( 7.505683250481794744, 15.49109367268993154, 9.369457576475557659 ) ) ;
#26241=CARTESIAN_POINT ( 'NONE',  ( -3.796053574490222626, 14.00000000000128964, -12.24940615670150557 ) ) ;
#26264=COLOUR_RGB ( '', 0.40784314, 0.44705882, 0.49803922) ;
#26272=DIRECTION ( 'NONE',  ( 3.706092522800016599E-15, 0.000000000000000000, 1.000000000000000000 ) ) ;
#26284=EDGE_LOOP ( 'NONE', ( #50992, #90066, #169161, #183469 ) ) ;
#26290=DIRECTION ( 'NONE',  ( -0.000000000000000000, -1.000000000000000000, -0.000000000000000000 ) ) ;
#26339=CARTESIAN_POINT ( 'NONE',  ( -11.94105721237523099, 12.69999999999999929, 1.187919463087245386 ) ) ;
#26357=CARTESIAN_POINT ( 'NONE',  ( 10.42254519813228697, 10.51899034650841358, 5.955849994509172518 ) ) ;
#26378=CARTESIAN_POINT ( 'NONE',  ( 9.868838213939689297, 9.992711175144377123, 6.338997305163716511 ) ) ;
#26395=CARTESIAN_POINT ( 'NONE',  ( 9.534369015033231420, 4.462424917548963421, -7.287319680779428488 ) ) ;
#26406=FACE_OUTER_BOUND ( 'NONE', #15395, .T. ) ;
#26426=EDGE_CURVE ( 'NONE', #45318, #123196, #55143, .T. ) ;
#26439=CARTESIAN_POINT ( 'NONE',  ( 0.3554123170488062700, 16.00000000000058265, 12.67999999502907649 ) ) ;
#26444=CARTESIAN_POINT ( 'NONE',  ( -11.84668730067608422, 12.69999999999999929, -1.320000000000001616 ) ) ;
#26455=EDGE_LOOP ( 'NONE', ( #122832, #113672, #148969, #80222 ) ) ;
#26479=( NAMED_UNIT ( * ) SI_UNIT ( $, .STERADIAN. ) SOLID_ANGLE_UNIT ( ) );
#26483=CARTESIAN_POINT ( 'NONE',  ( 7.449797558097145611, 15.00000000000000000, -10.26196259744787653 ) ) ;
#26485=CARTESIAN_POINT ( 'NONE',  ( 8.302289836269501677, 14.87052365979419655, 9.588395110663297416 ) ) ;
#26519=CARTESIAN_POINT ( 'NONE',  ( -11.24554764128284035, 7.016280722987462859, -5.611469924715791535 ) ) ;
#26532=SURFACE_STYLE_FILL_AREA ( #28681 ) ;
#26544=CARTESIAN_POINT ( 'NONE',  ( 9.954141305008279872, 11.52356260170056679, 6.707419562446313321 ) ) ;
#26555=AXIS2_PLACEMENT_3D ( 'NONE', #96198, #94068, #162247 ) ;
#26572=B_SPLINE_CURVE_WITH_KNOTS ( 'NONE', 3,
 ( #64419, #96949, #80675, #146765, #196553, #114309 ),
 .UNSPECIFIED., .F., .F.,
 ( 4, 2, 4 ),
 ( 0.000000000000000000, 0.0003144386176887254184, 0.0006288772353774508368 ),
 .UNSPECIFIED. ) ;
#26583=AXIS2_PLACEMENT_3D ( 'NONE', #210551, #47017, #62187 ) ;
#26596=CARTESIAN_POINT ( 'NONE',  ( -10.84254087577847869, 4.919568073182957413, 5.035408296252060545 ) ) ;
#26600=CARTESIAN_POINT ( 'NONE',  ( -11.86239285000045918, 9.719999999999982876, 1.812080536912751061 ) ) ;
#26601=CARTESIAN_POINT ( 'NONE',  ( 1.500000000000037748, 7.000000000000000000, 10.64483442802188051 ) ) ;
#26612=ORIENTED_EDGE ( 'NONE', *, *, #154830, .F. ) ;
#26625=SURFACE_STYLE_USAGE ( .BOTH. , #42911 ) ;
#26634=CARTESIAN_POINT ( 'NONE',  ( -10.61922739175395236, 7.618143447610075114, 4.514851702475597861 ) ) ;
#26635=( BOUNDED_SURFACE ( )  B_SPLINE_SURFACE ( 3, 2, ( 
 ( #79744, #213975, #130711 ),
 ( #145861, #113392, #80824 ),
 ( #146914, #64568, #65595 ),
 ( #44073, #101315, #99209 ),
 ( #68795, #51516, #2723 ),
 ( #35240, #167396, #182558 ) ),
 .UNSPECIFIED., .F., .F., .T. ) 
 B_SPLINE_SURFACE_WITH_KNOTS ( ( 4, 2, 4 ),
 ( 3, 3 ),
 ( 0.000000000000000000, 0.0003766365702389427796, 0.0007532731404778855592 ),
 ( 0.000000000000000000, 1.000000000000000000 ),
 .UNSPECIFIED. ) 
 GEOMETRIC_REPRESENTATION_ITEM ( )  RATIONAL_B_SPLINE_SURFACE ( (
 ( 1.000000000000000000, 0.7452309222762957264, 1.000000000000000000),
 ( 1.000000000000000000, 0.7451892422671803073, 1.000000000000000000),
 ( 1.000000000000000000, 0.7429606254238495522, 1.000000000000000000),
 ( 1.000000000000000000, 0.7311462761265991039, 1.000000000000000000),
 ( 1.000000000000000000, 0.7212257702791082803, 1.000000000000000000),
 ( 1.000000000000000000, 0.7071067811865475727, 1.000000000000000000) ) ) 
 REPRESENTATION_ITEM ( '' )  SURFACE ( )  );
#26651=EDGE_LOOP ( 'NONE', ( #132755, #109795, #102613, #71124 ) ) ;
#26670=AXIS2_PLACEMENT_3D ( 'NONE', #94989, #212957, #161035 ) ;
#26676=DIRECTION ( 'NONE',  ( 0.000000000000000000, 0.000000000000000000, -1.000000000000000000 ) ) ;
#26678=DIRECTION ( 'NONE',  ( -1.000000000000000000, 0.000000000000000000, 0.000000000000000000 ) ) ;
#26703=DIRECTION ( 'NONE',  ( -0.000000000000000000, -1.000000000000000000, 0.000000000000000000 ) ) ;
#26708=CARTESIAN_POINT ( 'NONE',  ( -11.30309668167796922, 5.150585336095395483, -5.742054036728553967 ) ) ;
#26725=ORIENTED_EDGE ( 'NONE', *, *, #179909, .T. ) ;
#26736=AXIS2_PLACEMENT_3D ( 'NONE', #99710, #136491, #101841 ) ;
#26760=CARTESIAN_POINT ( 'NONE',  ( 9.364998556596795254, 13.54474674066948481, 7.374496730960012236 ) ) ;
#26798=CIRCLE ( 'NONE', #213554, 11.92000000000000171 ) ;
#26801=TRIMMED_CURVE ( 'NONE', #107431, ( PARAMETER_VALUE ( 0.000000000000000000 ), #41697 ), ( PARAMETER_VALUE ( 0.8956647938578647938 ), #38470 ), .T., .PARAMETER. ) ;
#26803=UNCERTAINTY_MEASURE_WITH_UNIT (LENGTH_MEASURE( 1.000000000000000082E-05 ), #181442, 'distance_accuracy_value', 'NONE');
#26807=CARTESIAN_POINT ( 'NONE',  ( 11.05652804041138282, 8.011784944665652830, -4.552175959553207640 ) ) ;
#26810=CARTESIAN_POINT ( 'NONE',  ( -10.49167311136684688, 5.343773310534623455, 5.730690286876302331 ) ) ;
#26814=CARTESIAN_POINT ( 'NONE',  ( -9.472340321242439742, 14.62753308518765571, -7.367375265402272611 ) ) ;
#26845=CARTESIAN_POINT ( 'NONE',  ( 8.031406801462809497, 15.33901600305085822, -8.917679673117250516 ) ) ;
#26858=CIRCLE ( 'NONE', #199852, 11.92000000000000171 ) ;
#26889=CARTESIAN_POINT ( 'NONE',  ( 9.117697077661663485, 4.000000000000000888, 7.300000000000000711 ) ) ;
#26895=ORIENTED_EDGE ( 'NONE', *, *, #121307, .F. ) ;
#26898=CARTESIAN_POINT ( 'NONE',  ( 11.25411745265349239, 9.324508674553577237, -3.753762932364714811 ) ) ;
#26899=CARTESIAN_POINT ( 'NONE',  ( -10.90754186426655004, 4.636108433425621733, 4.485516275142084730 ) ) ;
#26907=VERTEX_POINT ( 'NONE', #26889 ) ;
#26925=CARTESIAN_POINT ( 'NONE',  ( 11.78331023100045627, 9.799999999999982947, 1.799999999999999600 ) ) ;
#26957=DIRECTION ( 'NONE',  ( 0.5994789404140898892, -1.444427003850258927E-16, 0.8003905296791063995 ) ) ;
#26964=AXIS2_PLACEMENT_3D ( 'NONE', #40550, #91442, #9099 ) ;
#26966=CARTESIAN_POINT ( 'NONE',  ( -10.60720700236483971, 4.242771947286448686, 5.515665583366017977 ) ) ;
#26968=ORIENTED_EDGE ( 'NONE', *, *, #91659, .F. ) ;
#27030=SURFACE_SIDE_STYLE ('',( #108366 ) ) ;
#27035=CARTESIAN_POINT ( 'NONE',  ( 11.48788097203293823, 12.26956945602309723, -3.469500700354831491 ) ) ;
#27042=ORIENTED_EDGE ( 'NONE', *, *, #153343, .T. ) ;
#27045=UNCERTAINTY_MEASURE_WITH_UNIT (LENGTH_MEASURE( 1.000000000000000082E-05 ), #109827, 'distance_accuracy_value', 'NONE');
#27052=AXIS2_PLACEMENT_3D ( 'NONE', #45796, #14313, #28456 ) ;
#27064=VERTEX_POINT ( 'NONE', #94060 ) ;
#27083=CARTESIAN_POINT ( 'NONE',  ( 11.86145016429272836, 10.90000000000000036, -1.100000000000002087 ) ) ;
#27096=CARTESIAN_POINT ( 'NONE',  ( -9.758535016135404305, 3.481548707830503631, -6.988337216065471758 ) ) ;
#27102=CARTESIAN_POINT ( 'NONE',  ( 11.78331023100045272, 12.29999999999998295, 1.799999999999999600 ) ) ;
#27129=CARTESIAN_POINT ( 'NONE',  ( 11.84668729410370602, 11.00620512324527134, 1.399999999999998357 ) ) ;
#27148=( NAMED_UNIT ( * ) SI_UNIT ( $, .STERADIAN. ) SOLID_ANGLE_UNIT ( ) );
#27164=CARTESIAN_POINT ( 'NONE',  ( 0.000000000000000000, 15.51887838114830132, 0.000000000000000000 ) ) ;
#27168=CARTESIAN_POINT ( 'NONE',  ( -11.81907076198602802, 13.75731224596479052, -1.592066415281275349 ) ) ;
#27170=EDGE_LOOP ( 'NONE', ( #149907, #23554, #94920, #47415 ) ) ;
#27178=VECTOR ( 'NONE', #132209, 1000.000000000000000 ) ;
#27185=CARTESIAN_POINT ( 'NONE',  ( -11.33772467203841572, 10.09267152018144209, 3.599999999999999201 ) ) ;
#27198=CARTESIAN_POINT ( 'NONE',  ( 11.88237264505823987, 12.34322961531682239, 0.9087825512662162097 ) ) ;
#27207=CARTESIAN_POINT ( 'NONE',  ( -11.44779963594988814, 13.40000000000000213, -3.600000000000000977 ) ) ;
#27269=SURFACE_SIDE_STYLE ('',( #138921 ) ) ;
#27280=CIRCLE ( 'NONE', #144978, 0.08000000000000020983 ) ;
#27291=CARTESIAN_POINT ( 'NONE',  ( 6.928203230275514990, 15.46950125723224723, 9.797958971132709749 ) ) ;
#27293=CARTESIAN_POINT ( 'NONE',  ( 11.04536101718726293, 10.90000000000000036, -1.100000000000002087 ) ) ;
#27305=UNCERTAINTY_MEASURE_WITH_UNIT (LENGTH_MEASURE( 1.000000000000000082E-05 ), #197918, 'distance_accuracy_value', 'NONE');
#27317=DIRECTION ( 'NONE',  ( -0.000000000000000000, -1.000000000000000000, -0.000000000000000000 ) ) ;
#27336=CARTESIAN_POINT ( 'NONE',  ( 11.86145016429273191, 10.19999999999999929, 1.099999999999996758 ) ) ;
#27360=DIRECTION ( 'NONE',  ( 2.486899575160350966E-14, 0.000000000000000000, -1.000000000000000000 ) ) ;
#27364=CARTESIAN_POINT ( 'NONE',  ( -8.165961478353519709, 14.48012443953052397, -8.838024359600046509 ) ) ;
#27367=MECHANICAL_DESIGN_GEOMETRIC_PRESENTATION_REPRESENTATION('',(#207328),#16979);
#27369=CARTESIAN_POINT ( 'NONE',  ( -11.35610322553117513, 13.61421628929174865, -3.553412924323506861 ) ) ;
#27372=EDGE_CURVE ( 'NONE', #29604, #122503, #99369, .T. ) ;
#27400=EDGE_CURVE ( 'NONE', #102205, #211122, #45931, .T. ) ;
#27403=SURFACE_SIDE_STYLE ('',( #143335 ) ) ;
#27426=ORIENTED_EDGE ( 'NONE', *, *, #4041, .F. ) ;
#27432=CARTESIAN_POINT ( 'NONE',  ( 11.52856953056122791, 8.442533071845224057, -3.352610243527511358 ) ) ;
#27448=CARTESIAN_POINT ( 'NONE',  ( 8.392483990243823300, 12.96120414926864761, -8.512620520037069483 ) ) ;
#27452=CARTESIAN_POINT ( 'NONE',  ( 0.000000000000000000, 9.799999999999998934, 0.000000000000000000 ) ) ;
#27454=ORIENTED_EDGE ( 'NONE', *, *, #102591, .T. ) ;
#27484=CIRCLE ( 'NONE', #72457, 12.00000000000000178 ) ;
#27506=CARTESIAN_POINT ( 'NONE',  ( -11.63061636551515043, 7.359134869736937645, 2.774776728778091783 ) ) ;
#27509=CARTESIAN_POINT ( 'NONE',  ( -11.33772463945037146, 13.39999999999998259, 3.599999999999999201 ) ) ;
#27512=ADVANCED_FACE ( 'NONE', ( #146009 ), #193484, .T. ) ;
#27514=LINE ( 'NONE', #64292, #132646 ) ;
#27540=CARTESIAN_POINT ( 'NONE',  ( -11.48243876534946040, 12.30000000000000071, -3.200000000000001510 ) ) ;
#27542=FACE_OUTER_BOUND ( 'NONE', #14392, .T. ) ;
#27551=SURFACE_SIDE_STYLE ('',( #43830 ) ) ;
#27555=CARTESIAN_POINT ( 'NONE',  ( 7.577342237528466029, 14.99429123645997919, -10.16790800466224987 ) ) ;
#27558=CARTESIAN_POINT ( 'NONE',  ( 9.188757668294085690, 13.26368734670581340, 9.042387243776373040 ) ) ;
#27591=CARTESIAN_POINT ( 'NONE',  ( -11.03396297008821847, 6.349565552376400746, 6.086320354413141231 ) ) ;
#27602=( NAMED_UNIT ( * ) PLANE_ANGLE_UNIT ( ) SI_UNIT ( $, .RADIAN. ) );
#27605=EDGE_CURVE ( 'NONE', #132967, #87946, #90720, .T. ) ;
#27609=ORIENTED_EDGE ( 'NONE', *, *, #30193, .F. ) ;
#27615=CARTESIAN_POINT ( 'NONE',  ( 11.92546669328318565, 7.608715049294008992, 0.8935118259774108562 ) ) ;
#27652=EDGE_CURVE ( 'NONE', #27064, #34845, #63936, .T. ) ;
#27680=SURFACE_STYLE_FILL_AREA ( #78559 ) ;
#27695=ADVANCED_FACE ( 'NONE', ( #208574 ), #60207, .F. ) ;
#27699=CARTESIAN_POINT ( 'NONE',  ( -10.10707714348148301, 4.359868340440408829, -5.857196085253971063 ) ) ;
#27710=CARTESIAN_POINT ( 'NONE',  ( -10.85768919388902809, 5.702095803505641491, 6.451939001899068771 ) ) ;
#27713=ORIENTED_EDGE ( 'NONE', *, *, #202741, .T. ) ;
#27715=( NAMED_UNIT ( * ) PLANE_ANGLE_UNIT ( ) SI_UNIT ( $, .RADIAN. ) );
#27741=CARTESIAN_POINT ( 'NONE',  ( -5.583800452342470244, 15.44693297529254394, 10.58116637897097156 ) ) ;
#27761=ORIENTED_EDGE ( 'NONE', *, *, #74029, .F. ) ;
#27782=CARTESIAN_POINT ( 'NONE',  ( -9.812680342707254866, 4.108039100808300148, -6.337802944732694677 ) ) ;
#27803=LINE ( 'NONE', #110192, #137156 ) ;
#27847=CYLINDRICAL_SURFACE ( 'NONE', #212136, 0.08000000000000020983 ) ;
#27849=CARTESIAN_POINT ( 'NONE',  ( 11.39332173424661754, 7.468513200851135458, 3.792645573777906343 ) ) ;
#27868=ADVANCED_FACE ( 'NONE', ( #95944 ), #13588, .F. ) ;
#27888=CARTESIAN_POINT ( 'NONE',  ( -9.608223705539561621, 15.11771569533321724, -7.189021993664028720 ) ) ;
#27923=CARTESIAN_POINT ( 'NONE',  ( 9.176494415247189451, 14.33413921510887334, -7.733462363332296086 ) ) ;
#27950=SURFACE_SIDE_STYLE ('',( #123419 ) ) ;
#27975=CARTESIAN_POINT ( 'NONE',  ( 12.13020669054560408, 8.043700598764450760, -3.170917236059372257 ) ) ;
#27982=CARTESIAN_POINT ( 'NONE',  ( -11.89839339040395316, 11.32877468403921561, -1.560885614203537219 ) ) ;
#28000=CYLINDRICAL_SURFACE ( 'NONE', #71035, 0.3999999999999996891 ) ;
#28016=DIRECTION ( 'NONE',  ( 0.000000000000000000, 0.000000000000000000, -1.000000000000000000 ) ) ;
#28030=CARTESIAN_POINT ( 'NONE',  ( -11.80248046418316044, 11.29999999999999893, -1.695421849633145017 ) ) ;
#28049=CARTESIAN_POINT ( 'NONE',  ( -10.46840923150435643, 4.018901537134061286, 5.775382485202497307 ) ) ;
#28078=DIRECTION ( 'NONE',  ( 0.000000000000000000, 1.485208455481716197E-16, -1.000000000000000000 ) ) ;
#28086=CARTESIAN_POINT ( 'NONE',  ( 1.500000000000035971, 8.500000000000000000, 9.886859966642587594 ) ) ;
#28124=CARTESIAN_POINT ( 'NONE',  ( -10.89402507593495351, 4.580915115640823210, 4.512369680550198936 ) ) ;
#28181=LINE ( 'NONE', #128965, #74335 ) ;
#28195=AXIS2_PLACEMENT_3D ( 'NONE', #52231, #16504, #82585 ) ;
#28196=DIRECTION ( 'NONE',  ( 0.000000000000000000, 0.000000000000000000, -1.000000000000000000 ) ) ;
#28202=ORIENTED_EDGE ( 'NONE', *, *, #58359, .F. ) ;
#28209=CARTESIAN_POINT ( 'NONE',  ( 1.423205080756849483, 7.980384757729337863, -10.65537363484302524 ) ) ;
#28219=CARTESIAN_POINT ( 'NONE',  ( 11.94105721237523277, 13.40000000000000036, 1.187919463087248273 ) ) ;
#28221=DIRECTION ( 'NONE',  ( 0.2684563758389248433, 0.000000000000000000, 0.9632918427306597087 ) ) ;
#28225=FILL_AREA_STYLE_COLOUR ( '', #13720 ) ;
#28231=DIRECTION ( 'NONE',  ( 1.000000000000000000, -0.000000000000000000, -0.000000000000000000 ) ) ;
#28237=VERTEX_POINT ( 'NONE', #3700 ) ;
#28240=CARTESIAN_POINT ( 'NONE',  ( 7.032125997333287692, 15.00041888085534758, 9.944927957745147040 ) ) ;
#28261=CARTESIAN_POINT ( 'NONE',  ( -10.14058302375764420, 3.661560415210057151, -6.348512455255221454 ) ) ;
#28262=VECTOR ( 'NONE', #105485, 1000.000000000000000 ) ;
#28269=DIRECTION ( 'NONE',  ( -0.9982742078614211811, 0.000000000000000000, 0.05872483221476467591 ) ) ;
#28289=CIRCLE ( 'NONE', #149351, 0.5000000000000011102 ) ;
#28291=DIRECTION ( 'NONE',  ( -0.000000000000000000, -1.000000000000000000, -0.000000000000000000 ) ) ;
#28337=CARTESIAN_POINT ( 'NONE',  ( -11.43195036480940452, 12.44475503714751596, 3.649565797774462883 ) ) ;
#28347=ORIENTED_EDGE ( 'NONE', *, *, #2148, .F. ) ;
#28351=CYLINDRICAL_SURFACE ( 'NONE', #7604, 0.3999999999999997446 ) ;
#28356=DIRECTION ( 'NONE',  ( 1.000000000000000000, -0.000000000000000000, -0.000000000000000000 ) ) ;
#28369=EDGE_CURVE ( 'NONE', #97972, #102205, #156576, .T. ) ;
#28370=CARTESIAN_POINT ( 'NONE',  ( 11.86239285000045740, 12.22000000000000064, -1.812080536912752837 ) ) ;
#28371=UNCERTAINTY_MEASURE_WITH_UNIT (LENGTH_MEASURE( 1.000000000000000082E-05 ), #141855, 'distance_accuracy_value', 'NONE');
#28373=DIRECTION ( 'NONE',  ( 1.000000000000000000, 0.000000000000000000, -0.000000000000000000 ) ) ;
#28378=CARTESIAN_POINT ( 'NONE',  ( 11.55950211276791251, 9.719999999999998863, -3.221476510067114329 ) ) ;
#28387=CARTESIAN_POINT ( 'NONE',  ( 0.7124089920921370389, 15.00000000000000711, -12.66466791154696558 ) ) ;
#28391=STYLED_ITEM ( 'NONE', ( #128509 ), #27868 ) ;
#28415=TOROIDAL_SURFACE ( 'NONE', #149470, 11.91999999999999993, 0.08000000000000000167 ) ;
#28456=DIRECTION ( 'NONE',  ( 1.000000000000000000, 0.000000000000000000, -0.000000000000000000 ) ) ;
#28463=B_SPLINE_CURVE_WITH_KNOTS ( 'NONE', 3,
 ( #65616, #113415, #99232, #33151, #14755, #128617 ),
 .UNSPECIFIED., .F., .F.,
 ( 4, 2, 4 ),
 ( 0.000000000000000000, 0.0003129200374289441730, 0.0006258400748578883460 ),
 .UNSPECIFIED. ) ;
#28495=CARTESIAN_POINT ( 'NONE',  ( 10.95308175811721085, 12.30000000000000071, -1.800000000000001155 ) ) ;
#28496=DIRECTION ( 'NONE',  ( -3.491481338843133750E-15, -0.000000000000000000, -1.000000000000000000 ) ) ;
#28507=CARTESIAN_POINT ( 'NONE',  ( 11.08477547810399244, 9.249705336231610175, 4.599939534163192789 ) ) ;
#28516=FACE_OUTER_BOUND ( 'NONE', #112147, .T. ) ;
#28519=ORIENTED_EDGE ( 'NONE', *, *, #74682, .F. ) ;
#28529=CARTESIAN_POINT ( 'NONE',  ( 11.62511067571025336, 6.983149424372863123, -1.890548432371299103 ) ) ;
#28542=ADVANCED_FACE ( 'NONE', ( #154267 ), #207394, .T. ) ;
#28562=CIRCLE ( 'NONE', #149630, 11.92000000000000171 ) ;
#28586=CARTESIAN_POINT ( 'NONE',  ( -11.45712800319830116, 6.924314249384663889, 3.420032739606327699 ) ) ;
#28589=CARTESIAN_POINT ( 'NONE',  ( 1.000000047849766815, 15.00000000000000355, 11.64874984998672325 ) ) ;
#28616=SURFACE_SIDE_STYLE ('',( #179139 ) ) ;
#28629=CARTESIAN_POINT ( 'NONE',  ( -9.857709926548130497, 3.999999999999961808, -6.855924459378331726 ) ) ;
#28633=CARTESIAN_POINT ( 'NONE',  ( 7.434378667490904924, 15.94454736155378960, -9.015675578808581392 ) ) ;
#28636=CARTESIAN_POINT ( 'NONE',  ( 8.794449440816208607, 13.45178754580079072, 7.697256810998330145 ) ) ;
#28655=EDGE_CURVE ( 'NONE', #205382, #97972, #102687, .T. ) ;
#28670=CARTESIAN_POINT ( 'NONE',  ( -11.52114515671133610, 8.081606464056415362, 2.192706985476595261 ) ) ;
#28681=FILL_AREA_STYLE ('',( #60105 ) ) ;
#28686=CARTESIAN_POINT ( 'NONE',  ( -9.568429106646000548, 14.89599861206369624, 7.242208005429680462 ) ) ;
#28687=EDGE_LOOP ( 'NONE', ( #51695, #113319, #178825, #29932, #103092, #33792, #156090, #136382, #84750, #99321, #107421, #155337, #172513, #53558, #151860, #52043, #120980, #70054 ) ) ;
#28693=CARTESIAN_POINT ( 'NONE',  ( 11.57559917528478799, 8.195707862866003168, 2.997126751995791594 ) ) ;
#28697=CARTESIAN_POINT ( 'NONE',  ( -1.423205080756851260, 7.980384757729337863, 10.65537363484302524 ) ) ;
#28699=AXIS2_PLACEMENT_3D ( 'NONE', #206231, #76243, #42709 ) ;
#28742=CARTESIAN_POINT ( 'NONE',  ( -11.80247861663003484, 13.79999999999998295, 1.695431928471866190 ) ) ;
#28743=CARTESIAN_POINT ( 'NONE',  ( -11.68274454005080365, 7.296694540733708934, -2.750247670129647215 ) ) ;
#28747=CIRCLE ( 'NONE', #25328, 0.08000000000000040412 ) ;
#28752=CARTESIAN_POINT ( 'NONE',  ( -11.40651083548348765, 7.885881328724557271, -3.736393980786399283 ) ) ;
#28764=EDGE_LOOP ( 'NONE', ( #199786, #68534, #184604, #14199 ) ) ;
#28776=CARTESIAN_POINT ( 'NONE',  ( 11.86145016429273191, 13.40000000000000036, -1.100000000000002087 ) ) ;
#28783=CARTESIAN_POINT ( 'NONE',  ( -11.65676533170044138, 6.358709890710655621, 4.978123860300238235 ) ) ;
#28791=VERTEX_POINT ( 'NONE', #1063 ) ;
#28798=EDGE_LOOP ( 'NONE', ( #124667, #158765, #166217, #77754 ) ) ;
#28802=CARTESIAN_POINT ( 'NONE',  ( -11.80235830595197655, 12.29999999999998295, 1.696088231482817399 ) ) ;
#28840=DIRECTION ( 'NONE',  ( 1.000000000000000000, -0.000000000000000000, -0.000000000000000000 ) ) ;
#28849=DIRECTION ( 'NONE',  ( 0.000000000000000000, 0.000000000000000000, 1.000000000000000000 ) ) ;
#28923=CARTESIAN_POINT ( 'NONE',  ( 10.95308175811721085, 9.799999999999998934, -1.800000000000001155 ) ) ;
#28930=( NAMED_UNIT ( * ) SI_UNIT ( $, .STERADIAN. ) SOLID_ANGLE_UNIT ( ) );
#28961=( GEOMETRIC_REPRESENTATION_CONTEXT ( 3 ) GLOBAL_UNCERTAINTY_ASSIGNED_CONTEXT ( ( #177832 ) ) GLOBAL_UNIT_ASSIGNED_CONTEXT ( ( #82587, #242, #184350 ) ) REPRESENTATION_CONTEXT ( 'NONE', 'WORKASPACE' ) );
#28965=CIRCLE ( 'NONE', #156990, 0.5000000000000006661 ) ;
#28983=CARTESIAN_POINT ( 'NONE',  ( -11.84668730067608777, 11.00634727754793651, 1.399999999999998579 ) ) ;
#28994=FACE_OUTER_BOUND ( 'NONE', #42507, .T. ) ;
#29019=AXIS2_PLACEMENT_3D ( 'NONE', #11012, #106455, #90169 ) ;
#29024=CARTESIAN_POINT ( 'NONE',  ( 9.648753602328147494, 3.729558873908992211, 7.135166886579831669 ) ) ;
#29043=CARTESIAN_POINT ( 'NONE',  ( 11.84103413958623818, 13.61004478473146229, 1.443924719788817423 ) ) ;
#29048=CARTESIAN_POINT ( 'NONE',  ( 9.780965096007749437, 12.99495041104594861, 8.039825270927440926 ) ) ;
#29049=CARTESIAN_POINT ( 'NONE',  ( -10.19097401674926395, 4.476076320095182304, 5.708917106338025960 ) ) ;
#29054=CARTESIAN_POINT ( 'NONE',  ( -11.92619526913699879, 10.90000000000000036, -1.328859060402686199 ) ) ;
#29081=CARTESIAN_POINT ( 'NONE',  ( 11.33772463945036790, 10.19999999999999929, -3.680000000000001048 ) ) ;
#29097=DIRECTION ( 'NONE',  ( 1.000000000000000000, -0.000000000000000000, -0.000000000000000000 ) ) ;
#29126=CARTESIAN_POINT ( 'NONE',  ( -11.84668730067608600, 19.00000000000000000, -1.320000000000001616 ) ) ;
#29138=EDGE_CURVE ( 'NONE', #8789, #46947, #97828, .T. ) ;
#29163=CARTESIAN_POINT ( 'NONE',  ( 11.84668730067608777, 12.59365272245202938, 1.399999999999998579 ) ) ;
#29177=MECHANICAL_DESIGN_GEOMETRIC_PRESENTATION_REPRESENTATION('',(#133108),#50056);
#29194=CARTESIAN_POINT ( 'NONE',  ( 0.0004021782957080999310, 14.56829811979804923, 11.92774320584193859 ) ) ;
#29255=CARTESIAN_POINT ( 'NONE',  ( -11.01135777277262129, 10.90000000000000036, -1.400000000000001910 ) ) ;
#29273=ORIENTED_EDGE ( 'NONE', *, *, #3092, .F. ) ;
#29310=CARTESIAN_POINT ( 'NONE',  ( 10.98546216864998826, 12.34258621008987866, 1.592236800091190396 ) ) ;
#29327=VERTEX_POINT ( 'NONE', #203521 ) ;
#29383=SURFACE_SIDE_STYLE ('',( #142097 ) ) ;
#29394=ORIENTED_EDGE ( 'NONE', *, *, #2690, .T. ) ;
#29397=ORIENTED_EDGE ( 'NONE', *, *, #125755, .F. ) ;
#29399=DIRECTION ( 'NONE',  ( -0.000000000000000000, -1.000000000000000000, -0.000000000000000000 ) ) ;
#29404=DIRECTION ( 'NONE',  ( 0.000000000000000000, 0.000000000000000000, 1.000000000000000000 ) ) ;
#29416=CARTESIAN_POINT ( 'NONE',  ( -11.41108574530292863, 12.34163144622367270, 3.405883542057530633 ) ) ;
#29424=VERTEX_POINT ( 'NONE', #122400 ) ;
#29439=ORIENTED_EDGE ( 'NONE', *, *, #139829, .F. ) ;
#29470=ORIENTED_EDGE ( 'NONE', *, *, #202242, .F. ) ;
#29504=CARTESIAN_POINT ( 'NONE',  ( 11.41381678389397614, 11.02879418241070830, 3.704697885617693753 ) ) ;
#29510=DIRECTION ( 'NONE',  ( 1.000000000000000000, -0.000000000000000000, -0.000000000000000000 ) ) ;
#29531=SURFACE_STYLE_USAGE ( .BOTH. , #77196 ) ;
#29569=DIRECTION ( 'NONE',  ( 0.000000000000000000, 1.000000000000000000, 0.000000000000000000 ) ) ;
#29588=VECTOR ( 'NONE', #186120, 1000.000000000000000 ) ;
#29603=CARTESIAN_POINT ( 'NONE',  ( 9.241773570968582874, 13.11902652889326504, 9.006041125820061666 ) ) ;
#29604=VERTEX_POINT ( 'NONE', #162273 ) ;
#29609=EDGE_LOOP ( 'NONE', ( #76178, #210081, #51408, #197019 ) ) ;
#29633=FACE_OUTER_BOUND ( 'NONE', #152879, .T. ) ;
#29648=DIRECTION ( 'NONE',  ( 0.000000000000000000, 1.000000000000000000, 0.000000000000000000 ) ) ;
#29658=CARTESIAN_POINT ( 'NONE',  ( -10.84253909858433218, 4.919570308430900596, -5.035411995924089723 ) ) ;
#29661=CARTESIAN_POINT ( 'NONE',  ( -9.117697077659110860, 16.00000000000574829, 7.299999999990590460 ) ) ;
#29682=CARTESIAN_POINT ( 'NONE',  ( 0.000000000000000000, 11.29999999999998117, 0.000000000000000000 ) ) ;
#29701=MECHANICAL_DESIGN_GEOMETRIC_PRESENTATION_REPRESENTATION('',(#123175),#133479);
#29703=CARTESIAN_POINT ( 'NONE',  ( -11.30167226555126980, 6.973387911292391550, 4.148494114740727490 ) ) ;
#29707=CARTESIAN_POINT ( 'NONE',  ( 8.541839355669758049, 15.38782976336730357, -7.875440542426230373 ) ) ;
#29710=CARTESIAN_POINT ( 'NONE',  ( 7.538246871973172780, 13.99683876731212884, 10.19897525888958789 ) ) ;
#29718=CARTESIAN_POINT ( 'NONE',  ( -11.35610322553117513, 11.11421628929174865, -3.553412924323506861 ) ) ;
#29740=CARTESIAN_POINT ( 'NONE',  ( -10.57232898948313604, 5.599354254162436817, 4.968808419985093039 ) ) ;
#29758=CARTESIAN_POINT ( 'NONE',  ( -9.494457024078482021, 15.33445319465660717, 7.338830937051257663 ) ) ;
#29766=CARTESIAN_POINT ( 'NONE',  ( 11.99956024306423785, 7.587643445255384478, 0.4561022673488305812 ) ) ;
#29782=EDGE_CURVE ( 'NONE', #127758, #53890, #101193, .T. ) ;
#29819=CARTESIAN_POINT ( 'NONE',  ( -11.99966943091182259, 8.028188729005464097, 0.5386726004062643014 ) ) ;
#29827=CARTESIAN_POINT ( 'NONE',  ( -12.00000782161162682, 9.022963770432253838, 0.3066704378487656868 ) ) ;
#29830=CARTESIAN_POINT ( 'NONE',  ( 11.89942855770814312, 13.79999999999999893, -0.7000000000000009548 ) ) ;
#29842=COLOUR_RGB ( '', 0.08235294, 0.09019608, 0.10196078) ;
#29846=CARTESIAN_POINT ( 'NONE',  ( -11.94105721237523099, 10.19999999999999929, 1.187919463087248273 ) ) ;
#29852=VECTOR ( 'NONE', #140530, 1000.000000000000000 ) ;
#29854=EDGE_CURVE ( 'NONE', #78193, #116248, #210753, .T. ) ;
#29858=CARTESIAN_POINT ( 'NONE',  ( -11.31901822352654641, 5.215070234333009758, -5.710337001866061968 ) ) ;
#29911=B_SPLINE_CURVE_WITH_KNOTS ( 'NONE', 3,
 ( #64250, #130392, #196383, #48024, #180132, #117319 ),
 .UNSPECIFIED., .F., .F.,
 ( 4, 2, 4 ),
 ( 0.000000000000000000, 0.0003778774010236168619, 0.0007557548020472337237 ),
 .UNSPECIFIED. ) ;
#29927=CARTESIAN_POINT ( 'NONE',  ( -10.44369633504468631, 5.112959841837462882, -5.232137017608346596 ) ) ;
#29932=ORIENTED_EDGE ( 'NONE', *, *, #37327, .T. ) ;
#29935=PRESENTATION_STYLE_ASSIGNMENT (( #13661 ) ) ;
#29942=AXIS2_PLACEMENT_3D ( 'NONE', #184411, #84790, #52296 ) ;
#29943=EDGE_LOOP ( 'NONE', ( #126753, #49101, #153179, #58864, #57822, #128190, #148822, #178631 ) ) ;
#29947=FACE_BOUND ( 'NONE', #103987, .T. ) ;
#29991=VECTOR ( 'NONE', #207709, 1000.000000000000000 ) ;
#30004=CIRCLE ( 'NONE', #99271, 0.08000000000000014044 ) ;
#30006=CARTESIAN_POINT ( 'NONE',  ( 11.89844258446855285, 9.771473106700369726, 1.560502987793273233 ) ) ;
#30017=ORIENTED_EDGE ( 'NONE', *, *, #12435, .T. ) ;
#30061=VECTOR ( 'NONE', #153985, 1000.000000000000000 ) ;
#30072=ADVANCED_FACE ( 'NONE', ( #161205 ), #82067, .F. ) ;
#30085=CARTESIAN_POINT ( 'NONE',  ( -10.82855876678636520, 5.585670971531701667, -6.509986581443756748 ) ) ;
#30099=CARTESIAN_POINT ( 'NONE',  ( 7.127284358736648784, 14.48154074412736669, -9.657187355191572564 ) ) ;
#30105=ORIENTED_EDGE ( 'NONE', *, *, #144093, .F. ) ;
#30108=CARTESIAN_POINT ( 'NONE',  ( 11.49537292513043951, 8.930514822958286913, -3.071439876058613461 ) ) ;
#30112=COLOUR_RGB ( '', 0.66274510, 0.83137255, 0.94901961) ;
#30117=FACE_OUTER_BOUND ( 'NONE', #223, .T. ) ;
#30119=ORIENTED_EDGE ( 'NONE', *, *, #47376, .T. ) ;
#30123=CARTESIAN_POINT ( 'NONE',  ( -9.367496997608917297, 14.57669131241553728, -7.413898975919227752 ) ) ;
#30136=( LENGTH_UNIT ( ) NAMED_UNIT ( * ) SI_UNIT ( .MILLI., .METRE. ) );
#30142=CARTESIAN_POINT ( 'NONE',  ( -9.367496997608871112, 15.42330868759649043, 7.413898975919298806 ) ) ;
#30144=ORIENTED_EDGE ( 'NONE', *, *, #183770, .T. ) ;
#30184=ORIENTED_EDGE ( 'NONE', *, *, #105724, .F. ) ;
#30193=EDGE_CURVE ( 'NONE', #4671, #59479, #119987, .T. ) ;
#30217=CARTESIAN_POINT ( 'NONE',  ( 11.89942855770814312, 9.799999999999998934, -0.7000000000000009548 ) ) ;
#30236=LINE ( 'NONE', #129948, #52822 ) ;
#30243=VERTEX_POINT ( 'NONE', #37596 ) ;
#30254=CARTESIAN_POINT ( 'NONE',  ( -9.437721056244807727, 14.51368701454513221, 7.411487925289132583 ) ) ;
#30259=DIRECTION ( 'NONE',  ( 0.000000000000000000, -1.000000000000000000, 0.000000000000000000 ) ) ;
#30261=CARTESIAN_POINT ( 'NONE',  ( 11.94105721237523277, 12.69999999999999929, -1.187919463087249827 ) ) ;
#30271=B_SPLINE_CURVE_WITH_KNOTS ( 'NONE', 3,
 ( #130584, #87079, #3660, #153149, #35115, #2602 ),
 .UNSPECIFIED., .F., .F.,
 ( 4, 2, 4 ),
 ( 0.000000000000000000, 0.0003157158648874029564, 0.0006314317297748059127 ),
 .UNSPECIFIED. ) ;
#30292=VECTOR ( 'NONE', #183455, 1000.000000000000000 ) ;
#30293=CARTESIAN_POINT ( 'NONE',  ( 11.07790593930098311, 12.30000000000000071, -0.7000000000000009548 ) ) ;
#30350=CARTESIAN_POINT ( 'NONE',  ( 11.55950211276791251, 12.30000000000000071, -3.221476510067115662 ) ) ;
#30374=ADVANCED_FACE ( 'NONE', ( #3998 ), #121070, .F. ) ;
#30384=CARTESIAN_POINT ( 'NONE',  ( 1.734723475976807094E-15, 15.00041888085534758, 12.17999951260719982 ) ) ;
#30389=CARTESIAN_POINT ( 'NONE',  ( 1.500000000000065503, 6.071532165918824830E-15, -10.99818166789400919 ) ) ;
#30393=VECTOR ( 'NONE', #7755, 1000.000000000000000 ) ;
#30396=ORIENTED_EDGE ( 'NONE', *, *, #34941, .T. ) ;
#30415=CARTESIAN_POINT ( 'NONE',  ( -11.88237264505823987, 9.843229615316904102, -0.9087825512663008087 ) ) ;
#30424=ORIENTED_EDGE ( 'NONE', *, *, #16302, .F. ) ;
#30448=VECTOR ( 'NONE', #196087, 1000.000000000000000 ) ;
#30462=CARTESIAN_POINT ( 'NONE',  ( -10.06346916285073334, 4.651885711879500285, -6.538199818904806726 ) ) ;
#30470=( BOUNDED_SURFACE ( )  B_SPLINE_SURFACE ( 3, 2, ( 
 ( #158301, #27207, #176671 ),
 ( #45621, #126942, #173498 ),
 ( #26142, #90102, #9892 ),
 ( #91176, #190767, #78095 ),
 ( #8830, #174566, #207023 ),
 ( #142072, #208086, #110671 ) ),
 .UNSPECIFIED., .F., .F., .F. ) 
 B_SPLINE_SURFACE_WITH_KNOTS ( ( 4, 2, 4 ),
 ( 3, 3 ),
 ( 0.000000000000000000, 0.0003831327362561331041, 0.0007662654725122662082 ),
 ( 0.000000000000000000, 1.000000000000000000 ),
 .UNSPECIFIED. ) 
 GEOMETRIC_REPRESENTATION_ITEM ( )  RATIONAL_B_SPLINE_SURFACE ( (
 ( 1.000000000000000000, 0.5879095031487548972, 1.000000000000000000),
 ( 1.000000000000000000, 0.5873691247577063068, 1.000000000000000000),
 ( 1.000000000000000000, 0.6054349545499626561, 1.000000000000000000),
 ( 1.000000000000000000, 0.6533334602764224730, 1.000000000000000000),
 ( 1.000000000000000000, 0.6828746263152883911, 1.000000000000000000),
 ( 1.000000000000000000, 0.7071067811865399122, 1.000000000000000000) ) ) 
 REPRESENTATION_ITEM ( '' )  SURFACE ( )  );
#30480=CIRCLE ( 'NONE', #58145, 0.08000000000000020983 ) ;
#30484=CARTESIAN_POINT ( 'NONE',  ( -11.97178994924802353, 13.87999993797205356, -0.8322011300497247355 ) ) ;
#30497=( NAMED_UNIT ( * ) SI_UNIT ( $, .STERADIAN. ) SOLID_ANGLE_UNIT ( ) );
#30509=VERTEX_POINT ( 'NONE', #140478 ) ;
#30520=CARTESIAN_POINT ( 'NONE',  ( -11.86145016429273191, 13.40000000000000036, 1.099999999999996758 ) ) ;
#30529=DIRECTION ( 'NONE',  ( 1.000000000000000000, -0.000000000000000000, -0.000000000000000000 ) ) ;
#30531=ORIENTED_EDGE ( 'NONE', *, *, #125943, .T. ) ;
#30537=VERTEX_POINT ( 'NONE', #159886 ) ;
#30560=EDGE_LOOP ( 'NONE', ( #104714, #73690, #186209, #82054, #77047, #114590, #137810, #55593 ) ) ;
#30603=VECTOR ( 'NONE', #88207, 1000.000000000000000 ) ;
#30607=EDGE_LOOP ( 'NONE', ( #67891, #183800, #202705, #93886 ) ) ;
#30633=EDGE_CURVE ( 'NONE', #197667, #19630, #91025, .T. ) ;
#30656=COLOUR_RGB ( '', 0.40784314, 0.44705882, 0.49803922) ;
#30657=CARTESIAN_POINT ( 'NONE',  ( 11.52676144591142915, 8.443953938884890320, 3.358931424421359502 ) ) ;
#30665=( LENGTH_UNIT ( ) NAMED_UNIT ( * ) SI_UNIT ( .MILLI., .METRE. ) );
#30675=CARTESIAN_POINT ( 'NONE',  ( 9.231319260696198015, 13.16052827424349303, 9.015053781678833644 ) ) ;
#30691=LINE ( 'NONE', #42685, #119560 ) ;
#30694=CARTESIAN_POINT ( 'NONE',  ( 11.04536101718726293, 12.69999999999999929, -1.100000000000000311 ) ) ;
#30706=LINE ( 'NONE', #144486, #93436 ) ;
#30729=DIRECTION ( 'NONE',  ( 0.000000000000000000, 0.000000000000000000, 1.000000000000000000 ) ) ;
#30732=CARTESIAN_POINT ( 'NONE',  ( -7.247736482492992849, 15.00000000000182077, 10.57961706324680584 ) ) ;
#30775=CARTESIAN_POINT ( 'NONE',  ( -9.604686356149278126, 3.999999999999997335, -7.193747284969076894 ) ) ;
#30779=CARTESIAN_POINT ( 'NONE',  ( 9.573135803333604699, 13.80976963840737248, -8.295511852730781399 ) ) ;
#30782=CARTESIAN_POINT ( 'NONE',  ( 8.745502095769714046, 13.65234029860456388, 7.751384471964883893 ) ) ;
#30811=STYLED_ITEM ( 'NONE', ( #8520 ), #36249 ) ;
#30814=CARTESIAN_POINT ( 'NONE',  ( -10.45142682343936791, 5.144546645612242841, 5.216777551074719632 ) ) ;
#30824=B_SPLINE_CURVE_WITH_KNOTS ( 'NONE', 3,
 ( #103868, #203460, #156892, #21503, #55114, #24727 ),
 .UNSPECIFIED., .F., .F.,
 ( 4, 2, 4 ),
 ( 0.001105973075985145371, 0.001142139074170123950, 0.001178305072355102529 ),
 .UNSPECIFIED. ) ;
#30835=VERTEX_POINT ( 'NONE', #39736 ) ;
#30842=CARTESIAN_POINT ( 'NONE',  ( 11.80883292463478185, 7.903546609398427236, -2.174370349999172891 ) ) ;
#30892=CARTESIAN_POINT ( 'NONE',  ( -11.77663116055808601, 7.701210053843842829, -2.069426955518140598 ) ) ;
#30901=CIRCLE ( 'NONE', #58555, 0.07999999999999998779 ) ;
#30902=CARTESIAN_POINT ( 'NONE',  ( -11.81513045596701694, 8.669530242206672455, -2.119415056513991313 ) ) ;
#30906=DIRECTION ( 'NONE',  ( 0.000000000000000000, -0.000000000000000000, 1.000000000000000000 ) ) ;
#30931=CARTESIAN_POINT ( 'NONE',  ( -12.00295043402534212, 5.507662538472692049, -4.496421502479775789 ) ) ;
#30934=EDGE_LOOP ( 'NONE', ( #179790, #143357, #27609, #78222 ) ) ;
#30938=ORIENTED_EDGE ( 'NONE', *, *, #47755, .F. ) ;
#30951=DIRECTION ( 'NONE',  ( 0.1510067114093955887, 0.000000000000000000, -0.9885327375000383388 ) ) ;
#30980=EDGE_LOOP ( 'NONE', ( #52826, #137642, #9492, #213325 ) ) ;
#31000=CARTESIAN_POINT ( 'NONE',  ( -10.37923916842784422, 4.890109552615133026, -5.358306740738790097 ) ) ;
#31009=DIRECTION ( 'NONE',  ( 0.000000000000000000, 0.000000000000000000, 1.000000000000000000 ) ) ;
#31013=ADVANCED_FACE ( 'NONE', ( #25606 ), #135307, .T. ) ;
#31068=AXIS2_PLACEMENT_3D ( 'NONE', #83764, #20875, #170350 ) ;
#31134=( NAMED_UNIT ( * ) SI_UNIT ( $, .STERADIAN. ) SOLID_ANGLE_UNIT ( ) );
#31136=CARTESIAN_POINT ( 'NONE',  ( 9.150980377513773689, 14.30259500125689698, -7.763699605349790644 ) ) ;
#31140=DIRECTION ( 'NONE',  ( 1.000000000000000000, -0.000000000000000000, -0.000000000000000000 ) ) ;
#31143=EDGE_CURVE ( 'NONE', #144257, #101488, #142832, .T. ) ;
#31161=CARTESIAN_POINT ( 'NONE',  ( -10.37923916842784422, 4.890109552615133026, -5.358306740738790097 ) ) ;
#31184=CARTESIAN_POINT ( 'NONE',  ( 9.680359324772695118, 13.43752487939448947, 8.167046318416051776 ) ) ;
#31192=( LENGTH_UNIT ( ) NAMED_UNIT ( * ) SI_UNIT ( .MILLI., .METRE. ) );
#31193=CARTESIAN_POINT ( 'NONE',  ( 7.321368706613687216, 14.46581668038550994, -9.510808679899710683 ) ) ;
#31210=CARTESIAN_POINT ( 'NONE',  ( -11.92619526913700057, 11.02781666661243243, -1.328859060402685976 ) ) ;
#31214=CARTESIAN_POINT ( 'NONE',  ( 1.271070482942026292, 8.436788551174032591, 10.93994114196923029 ) ) ;
#31217=CARTESIAN_POINT ( 'NONE',  ( -9.495441445486425991, 14.82923372934912365, 7.231220947886405348 ) ) ;
#31223=CARTESIAN_POINT ( 'NONE',  ( -11.33772463945037146, 10.89999999999998259, 3.599999999999999201 ) ) ;
#31226=CARTESIAN_POINT ( 'NONE',  ( -9.437721055127425984, 15.48631298644891352, -7.411487926712346130 ) ) ;
#31250=CARTESIAN_POINT ( 'NONE',  ( -10.44369227015510049, 5.112964020592959180, 5.232143560358710310 ) ) ;
#31255=SURFACE_STYLE_USAGE ( .BOTH. , #109370 ) ;
#31288=DIRECTION ( 'NONE',  ( 0.9982742078614211811, 0.000000000000000000, 0.05872483221476467591 ) ) ;
#31298=CARTESIAN_POINT ( 'NONE',  ( 0.000000000000000000, 11.37999999999998302, 0.000000000000000000 ) ) ;
#31340=B_SPLINE_CURVE_WITH_KNOTS ( 'NONE', 3,
 ( #75644, #188310, #155831, #7415, #65740, #12743, #29024, #130847, #63649, #195784 ),
 .UNSPECIFIED., .F., .F.,
 ( 4, 2, 2, 2, 4 ),
 ( 0.000000000000000000, 0.0004096327454563874798, 0.0008192654909127749597, 0.001228898236369162494, 0.001638530981825549919 ),
 .UNSPECIFIED. ) ;
#31390=CARTESIAN_POINT ( 'NONE',  ( 8.362811809344231406, 14.02572535640353735, 8.606655576677448849 ) ) ;
#31394=VECTOR ( 'NONE', #110129, 1000.000000000000000 ) ;
#31414=CARTESIAN_POINT ( 'NONE',  ( 11.84668730067608600, 10.89999999999998259, 1.399999999999998357 ) ) ;
#31449=CARTESIAN_POINT ( 'NONE',  ( -9.367496997601190145, 14.57669131240758276, 7.413898975931879853 ) ) ;
#31453=LINE ( 'NONE', #30389, #30448 ) ;
#31488=DIRECTION ( 'NONE',  ( 1.000000000000000000, -0.000000000000000000, -0.000000000000000000 ) ) ;
#31500=CARTESIAN_POINT ( 'NONE',  ( -11.78331023100045627, 11.37999999999999901, -1.800000000000001155 ) ) ;
#31572=EDGE_LOOP ( 'NONE', ( #72075, #180227, #89538, #7713 ) ) ;
#31613=ORIENTED_EDGE ( 'NONE', *, *, #198798, .T. ) ;
#31625=ORIENTED_EDGE ( 'NONE', *, *, #187512, .T. ) ;
#31644=VERTEX_POINT ( 'NONE', #213676 ) ;
#31668=SURFACE_STYLE_FILL_AREA ( #106829 ) ;
#31671=ORIENTED_EDGE ( 'NONE', *, *, #168035, .T. ) ;
#31680=VECTOR ( 'NONE', #29510, 1000.000000000000000 ) ;
#31691=VERTEX_POINT ( 'NONE', #182260 ) ;
#31694=CARTESIAN_POINT ( 'NONE',  ( 0.08011315927822239280, 14.48238172885137587, 11.99973258290723699 ) ) ;
#31701=DIRECTION ( 'NONE',  ( 1.000000000000000000, -0.000000000000000000, -0.000000000000000000 ) ) ;
#31711=CARTESIAN_POINT ( 'NONE',  ( 11.97181073603049306, 9.719999999999998863, -0.8318477717169578955 ) ) ;
#31714=ORIENTED_EDGE ( 'NONE', *, *, #150811, .F. ) ;
#31723=VERTEX_POINT ( 'NONE', #200631 ) ;
#31730=CARTESIAN_POINT ( 'NONE',  ( -15.75000000000000000, 13.40000000000000036, 1.099999999999996758 ) ) ;
#31741=CARTESIAN_POINT ( 'NONE',  ( 9.687436728043250511, 13.40831512142563042, -8.157569025435085663 ) ) ;
#31750=B_SPLINE_CURVE_WITH_KNOTS ( 'NONE', 3,
 ( #86868, #203788, #185420, #23985, #122669, #91161 ),
 .UNSPECIFIED., .F., .F.,
 ( 4, 2, 4 ),
 ( 0.000000000000000000, 0.0003155923098472861849, 0.0006311846196945723698 ),
 .UNSPECIFIED. ) ;
#31765=DIRECTION ( 'NONE',  ( 0.000000000000000000, 0.000000000000000000, 1.000000000000000000 ) ) ;
#31794=CARTESIAN_POINT ( 'NONE',  ( -11.68373919224753266, 7.485257342004228320, -2.542923528616539919 ) ) ;
#31802=CARTESIAN_POINT ( 'NONE',  ( -1.499999999999963141, 7.750000000000000000, 10.99818166789402341 ) ) ;
#31840=CARTESIAN_POINT ( 'NONE',  ( 9.149559100784346199, 14.18285160050866445, -6.998392133554209416 ) ) ;
#31874=CARTESIAN_POINT ( 'NONE',  ( -11.97711842482174305, 7.451475930019106464, -0.9249707317075172019 ) ) ;
#31880=EDGE_CURVE ( 'NONE', #173258, #28237, #16999, .T. ) ;
#31893=FACE_OUTER_BOUND ( 'NONE', #113563, .T. ) ;
#31894=CARTESIAN_POINT ( 'NONE',  ( -9.383668910090971593, 14.59391485664907151, 7.388226147404734157 ) ) ;
#31914=CARTESIAN_POINT ( 'NONE',  ( 11.80248046418316044, 9.800000000000000711, -1.695421849633145017 ) ) ;
#31935=CARTESIAN_POINT ( 'NONE',  ( -8.752381174298911048, 14.55265199826961364, -8.156849355156190029 ) ) ;
#31947=CARTESIAN_POINT ( 'NONE',  ( -11.93088452921365139, 7.924368216754111849, -1.311419307916881216 ) ) ;
#31956=CARTESIAN_POINT ( 'NONE',  ( -11.86159218342442756, 8.823409521868983418, 1.516044442424843153 ) ) ;
#31959=( LENGTH_UNIT ( ) NAMED_UNIT ( * ) SI_UNIT ( .MILLI., .METRE. ) );
#31967=ORIENTED_EDGE ( 'NONE', *, *, #209339, .T. ) ;
#31981=DIRECTION ( 'NONE',  ( 0.000000000000000000, 0.000000000000000000, 1.000000000000000000 ) ) ;
#32004=CARTESIAN_POINT ( 'NONE',  ( -11.01135777277262129, 12.69999999999998153, 1.399999999999998579 ) ) ;
#32022=CARTESIAN_POINT ( 'NONE',  ( 9.475937985776960559, 4.398642190548692987, 7.290290962746384551 ) ) ;
#32053=ORIENTED_EDGE ( 'NONE', *, *, #13361, .F. ) ;
#32063=( BOUNDED_SURFACE ( )  B_SPLINE_SURFACE ( 3, 2, ( 
 ( #193736, #157001, #41122 ),
 ( #110435, #191594, #42189 ),
 ( #59476, #173255, #44313 ),
 ( #108304, #92010, #158068 ),
 ( #28049, #7510, #9656 ),
 ( #75732, #43255, #109374 ),
 ( #26966, #93072, #159114 ),
 ( #142906, #177504, #127781 ),
 ( #208906, #60539, #160181 ),
 ( #77855, #45382, #111498 ) ),
 .UNSPECIFIED., .F., .F., .T. ) 
 B_SPLINE_SURFACE_WITH_KNOTS ( ( 4, 2, 2, 2, 4 ),
 ( 3, 3 ),
 ( -2.385244779468109755E-18, 0.001523370301547610686, 0.001904212876934514116, 0.002285055452321417546, 0.003046740603095223973 ),
 ( 0.000000000000000000, 1.000000000000000000 ),
 .UNSPECIFIED. ) 
 GEOMETRIC_REPRESENTATION_ITEM ( )  RATIONAL_B_SPLINE_SURFACE ( (
 ( 1.000000000000000000, 0.8509629433967623724, 1.000000000000000000),
 ( 1.000000000000000000, 0.8506945359964187547, 1.000000000000000000),
 ( 1.000000000000000000, 0.8506364743628531677, 1.000000000000000000),
 ( 1.000000000000000000, 0.8494736702895108182, 1.000000000000000000),
 ( 1.000000000000000000, 0.8491834653876565442, 1.000000000000000000),
 ( 1.000000000000000000, 0.8486037118729093942, 1.000000000000000000),
 ( 1.000000000000000000, 0.8483092994974581469, 1.000000000000000000),
 ( 1.000000000000000000, 0.8474113007901487027, 1.000000000000000000),
 ( 1.000000000000000000, 0.8467927356708078168, 1.000000000000000000),
 ( 1.000000000000000000, 0.8462409035376579070, 1.000000000000000000) ) ) 
 REPRESENTATION_ITEM ( '' )  SURFACE ( )  );
#32069=DIRECTION ( 'NONE',  ( -0.000000000000000000, -1.000000000000000000, -0.000000000000000000 ) ) ;
#32091=UNCERTAINTY_MEASURE_WITH_UNIT (LENGTH_MEASURE( 1.000000000000000082E-05 ), #209041, 'distance_accuracy_value', 'NONE');
#32124=ADVANCED_FACE ( 'NONE', ( #108991 ), #95465, .T. ) ;
#32129=DIRECTION ( 'NONE',  ( 0.000000000000000000, 0.000000000000000000, 1.000000000000000000 ) ) ;
#32138=CIRCLE ( 'NONE', #201561, 11.95586206896558146 ) ;
#32146=FACE_OUTER_BOUND ( 'NONE', #97014, .T. ) ;
#32200=AXIS2_PLACEMENT_3D ( 'NONE', #176607, #78028, #75902 ) ;
#32213=CARTESIAN_POINT ( 'NONE',  ( -9.470156251935129887, 4.005132839944305800, -6.837168546664702085 ) ) ;
#32215=B_SPLINE_CURVE_WITH_KNOTS ( 'NONE', 3,
 ( #142858, #75689, #208861, #154812, #176395, #144988, #213126, #65788, #194759, #112512 ),
 .UNSPECIFIED., .F., .F.,
 ( 4, 2, 2, 2, 4 ),
 ( 0.000000000000000000, 0.0003519860449266724498, 0.0007039720898533448996, 0.001055958134780017295, 0.001407944179706689799 ),
 .UNSPECIFIED. ) ;
#32229=CARTESIAN_POINT ( 'NONE',  ( 8.125020845233269284, 14.19599321528319891, -8.831577418034537885 ) ) ;
#32235=EDGE_LOOP ( 'NONE', ( #117717, #170910, #146245, #42548, #35236 ) ) ;
#32237=CARTESIAN_POINT ( 'NONE',  ( 10.16812126801399607, 13.45311586547773963, 7.234909159705820159 ) ) ;
#32248=CARTESIAN_POINT ( 'NONE',  ( -11.86145016429273191, 12.69999999999999929, 1.099999999999996758 ) ) ;
#32256=CARTESIAN_POINT ( 'NONE',  ( 0.02465192458550417853, 14.53714098577670910, 11.97749476893806353 ) ) ;
#32275=DIRECTION ( 'NONE',  ( -0.000000000000000000, 1.000000000000000000, 0.000000000000000000 ) ) ;
#32340=UNCERTAINTY_MEASURE_WITH_UNIT (LENGTH_MEASURE( 1.000000000000000082E-05 ), #87568, 'distance_accuracy_value', 'NONE');
#32347=DIRECTION ( 'NONE',  ( 0.000000000000000000, -1.000000000000000000, -1.804652791718263484E-16 ) ) ;
#32374=ORIENTED_EDGE ( 'NONE', *, *, #73951, .F. ) ;
#32386=CARTESIAN_POINT ( 'NONE',  ( -9.608224291022223085, 14.88196956744644872, 7.189021211163121983 ) ) ;
#32447=CARTESIAN_POINT ( 'NONE',  ( 8.128354040209304188, 14.19343821084924961, 8.828530592764916918 ) ) ;
#32449=FACE_OUTER_BOUND ( 'NONE', #179560, .T. ) ;
#32512=DIRECTION ( 'NONE',  ( 0.000000000000000000, 0.000000000000000000, -1.000000000000000000 ) ) ;
#32513=CARTESIAN_POINT ( 'NONE',  ( -11.48784849554592924, 11.33049527181932348, 3.469614872287846374 ) ) ;
#32522=CARTESIAN_POINT ( 'NONE',  ( -11.52460864928264961, 11.37999999999998302, 3.346683403123524858 ) ) ;
#32532=FILL_AREA_STYLE ('',( #14122 ) ) ;
#32553=CARTESIAN_POINT ( 'NONE',  ( 11.41381675112453387, 10.19999999999999929, -3.704697986577184299 ) ) ;
#32558=CARTESIAN_POINT ( 'NONE',  ( 1.423205080756849483, 7.980384757729337863, -10.65537363484302524 ) ) ;
#32578=CARTESIAN_POINT ( 'NONE',  ( -10.07315204383574070, 4.605425058967329122, -6.523384448309665906 ) ) ;
#32596=CARTESIAN_POINT ( 'NONE',  ( -11.33772463945036968, 12.69999999999999929, -3.600000000000000977 ) ) ;
#32599=CARTESIAN_POINT ( 'NONE',  ( 11.33772463945037146, 10.89999999999998259, 3.679999999999999272 ) ) ;
#32614=DIRECTION ( 'NONE',  ( 0.000000000000000000, 1.000000000000000000, 0.000000000000000000 ) ) ;
#32621=ORIENTED_EDGE ( 'NONE', *, *, #134538, .F. ) ;
#32642=PRESENTATION_STYLE_ASSIGNMENT (( #83513 ) ) ;
#32670=ADVANCED_FACE ( 'NONE', ( #40483 ), #139726, .T. ) ;
#32674=CARTESIAN_POINT ( 'NONE',  ( -9.404345922919858936, 15.50976053221675599, -7.453791880891735389 ) ) ;
#32676=CLOSED_SHELL ( 'NONE', ( #134755, #169434, #75205, #197107, #33036, #66139, #173474, #206242, #14385, #198198, #46146, #81158, #94222, #214049, #24176, #10376, #135408, #152018, #143141, #192819, #35568, #21012, #175193, #157787, #101103, #145317, #55827, #163490, #86239, #36249, #125288, #55927, #74771, #133060, #169204, #197622, #77868, #116367, #141351, #169296, #143536, #7720, #186074, #46551, #115007, #105592, #198182, #86694, #149381, #98352, #60652, #30072, #185816, #95835, #61220, #16025, #10478, #120967, #189006, #48566, #87889, #86095, #7322, #136503, #185241, #162075, #154563, #55200, #146262, #150547, #135185, #143583, #39677, #101631, #40567, #146365, #202610, #1037, #151177, #34286, #76119, #213132, #60799, #43714, #190216, #9062, #2404, #111806, #15532, #98770, #147970, #99019, #145158, #114086, #136888, #22947, #15900, #113029, #70312, #100155, #25342, #146775, #212553, #172902, #163756, #105052, #191869, #60737, #196848, #121375, #106360, #72370, #111664, #65706, #171225, #196354, #50792, #186082, #128748, #27695, #39092, #173118, #180544, #50933, #140161, #66312, #40584, #170192, #69155, #30374, #47427, #27868, #165716, #143840, #146923, #175851, #10427, #12269, #36362, #121529, #22375, #68069, #138807, #126979, #209951, #93174, #181100, #150077, #87990, #120289, #133288, #208777, #93262, #189039, #72107, #96551, #70585, #144802, #31013, #83439, #22259, #177060, #203686, #155273, #32124, #203276, #73844, #73824, #44794, #49779, #59695, #67434, #64700, #173700, #18346, #700, #47594, #67615, #83397, #130489, #143171, #16928, #131070, #154453, #93398, #64653, #149288, #10546, #44536, #149471, #166168, #85012, #166422, #145987, #190768, #164824, #97191, #195777, #81120, #28542, #92742, #138008, #78549, #104042, #4062, #143974, #33077, #123133, #152840, #174852, #100264, #83027, #134672, #6508, #12661, #129857, #34373, #110536, #212203, #122460, #14322, #121705, #162137, #149566, #203343, #162916, #167196, #131555, #160853, #133311, #42805, #168286, #148360, #7162, #147303, #39361, #92686, #195279, #116428, #101222, #105167, #180011, #53360, #121612, #104148, #202720, #138556, #79919, #209118, #103616, #203116, #36680, #81679, #54371, #114357, #38413, #36230, #112278, #38177, #32670, #130424, #69419, #79880, #68434, #156833, #55407, #74008, #102261, #124045, #76215, #130902, #183529, #40612, #27512, #95314, #187021, #182283, #169250, #23143, #44223, #57608, #43267, #97754, #176115, #57047, #91304 ) ) ;
#32698=DIRECTION ( 'NONE',  ( -0.1510067114093955887, 0.000000000000000000, 0.9885327375000383388 ) ) ;
#32733=AXIS2_PLACEMENT_3D ( 'NONE', #80411, #68396, #199466 ) ;
#32743=CARTESIAN_POINT ( 'NONE',  ( 0.06970559732634250272, 14.49275370307429078, 11.99964040566942636 ) ) ;
#32769=ORIENTED_EDGE ( 'NONE', *, *, #168266, .T. ) ;
#32774=CARTESIAN_POINT ( 'NONE',  ( -11.84668730067608422, 10.19999999999999929, -1.400000000000001688 ) ) ;
#32796=CARTESIAN_POINT ( 'NONE',  ( 8.350859280846272270, 13.12796858787615406, 8.536646826506961716 ) ) ;
#32799=ORIENTED_EDGE ( 'NONE', *, *, #197971, .T. ) ;
#32811=DIRECTION ( 'NONE',  ( 0.000000000000000000, 1.000000000000000000, 0.000000000000000000 ) ) ;
#32817=CARTESIAN_POINT ( 'NONE',  ( 11.33772463945036790, 11.00911576511426304, -3.600000000000000089 ) ) ;
#32837=DIRECTION ( 'NONE',  ( 1.598721155460225418E-14, 0.000000000000000000, 1.000000000000000000 ) ) ;
#32839=ORIENTED_EDGE ( 'NONE', *, *, #117837, .F. ) ;
#32845=FACE_OUTER_BOUND ( 'NONE', #147880, .T. ) ;
#32879=VECTOR ( 'NONE', #140731, 1000.000000000000000 ) ;
#32892=CARTESIAN_POINT ( 'NONE',  ( 7.322014706700720410, 14.95386301424541031, -9.100409427799018403 ) ) ;
#32909=EDGE_CURVE ( 'NONE', #181928, #174805, #205362, .T. ) ;
#32913=CARTESIAN_POINT ( 'NONE',  ( 11.86239285000046095, 13.80000000000000249, -1.812080536912752837 ) ) ;
#32925=CARTESIAN_POINT ( 'NONE',  ( -10.45911201557330195, 5.175391108250987138, -5.201428006079835242 ) ) ;
#32930=CARTESIAN_POINT ( 'NONE',  ( 9.319695500903007357, 13.69389061776176142, -7.486440698825377105 ) ) ;
#32948=CARTESIAN_POINT ( 'NONE',  ( -9.380156870162490890, 14.53091807600370622, 7.484187822888271668 ) ) ;
#32956=CARTESIAN_POINT ( 'NONE',  ( 9.818094122049513928, 11.89513723134471590, -6.902820345984630457 ) ) ;
#32963=DIRECTION ( 'NONE',  ( -1.124869321039521280E-29, -7.437565543542506798E-15, 1.000000000000000000 ) ) ;
#32968=CARTESIAN_POINT ( 'NONE',  ( 11.84668730067608244, 12.69999999999999929, -1.400000000000001688 ) ) ;
#32989=DIRECTION ( 'NONE',  ( -0.000000000000000000, 1.000000000000000000, 9.023263958591317418E-17 ) ) ;
#33004=CARTESIAN_POINT ( 'NONE',  ( -11.50317709352769313, 6.904469223105409448, -3.423499370531426056 ) ) ;
#33012=CARTESIAN_POINT ( 'NONE',  ( -11.81385154090469847, 8.719572692708162265, 2.126314287815780357 ) ) ;
#33030=CARTESIAN_POINT ( 'NONE',  ( -15.75000000000000000, 12.69999999999999929, 0.6999999999999992895 ) ) ;
#33036=ADVANCED_FACE ( 'NONE', ( #177905 ), #85985, .F. ) ;
#33058=VERTEX_POINT ( 'NONE', #132384 ) ;
#33064=CARTESIAN_POINT ( 'NONE',  ( 11.35569630219380777, 13.61268439291370314, -3.554478010595023107 ) ) ;
#33077=ADVANCED_FACE ( 'NONE', ( #114042 ), #65248, .T. ) ;
#33114=ORIENTED_EDGE ( 'NONE', *, *, #14697, .F. ) ;
#33151=CARTESIAN_POINT ( 'NONE',  ( 11.04986610412592363, 11.10944100431282600, 1.056385672146459953 ) ) ;
#33177=CARTESIAN_POINT ( 'NONE',  ( -10.45911050446410506, 5.175404930453152197, 5.201426885097844455 ) ) ;
#33178=EDGE_CURVE ( 'NONE', #83814, #10371, #103305, .T. ) ;
#33197=ORIENTED_EDGE ( 'NONE', *, *, #19314, .F. ) ;
#33203=UNCERTAINTY_MEASURE_WITH_UNIT (LENGTH_MEASURE( 1.000000000000000082E-05 ), #161297, 'distance_accuracy_value', 'NONE');
#33214=CARTESIAN_POINT ( 'NONE',  ( -11.89197415570408900, 9.800000000000000711, 0.8055989572471843330 ) ) ;
#33216=STYLED_ITEM ( 'NONE', ( #190387 ), #95835 ) ;
#33226=AXIS2_PLACEMENT_3D ( 'NONE', #139668, #107204, #9628 ) ;
#33269=CARTESIAN_POINT ( 'NONE',  ( -10.81659741420782872, 5.544487526538591560, -6.534070432124610583 ) ) ;
#33284=CARTESIAN_POINT ( 'NONE',  ( 9.310341921297071721, 11.46515425228529494, -7.574253667434096116 ) ) ;
#33294=CARTESIAN_POINT ( 'NONE',  ( 9.262911828397729863, 13.60048340123860200, -6.822320103072770259 ) ) ;
#33304=CARTESIAN_POINT ( 'NONE',  ( 7.859932111734047488, 14.38583806649917918, -9.009653343056649888 ) ) ;
#33306=ORIENTED_EDGE ( 'NONE', *, *, #151300, .F. ) ;
#33307=CARTESIAN_POINT ( 'NONE',  ( 11.86239285000045740, 9.719999999999982876, 1.812080536912751061 ) ) ;
#33310=VECTOR ( 'NONE', #6600, 1000.000000000000000 ) ;
#33354=CARTESIAN_POINT ( 'NONE',  ( -10.33433454857960321, 4.766519530047388820, -5.444264161973041638 ) ) ;
#33452=CARTESIAN_POINT ( 'NONE',  ( -0.008622031262367491067, 15.44736672593548299, 11.95585889282746450 ) ) ;
#33454=VERTEX_POINT ( 'NONE', #3376 ) ;
#33478=CARTESIAN_POINT ( 'NONE',  ( 11.41108574530281672, 11.25836855377622392, 3.405883542057599911 ) ) ;
#33483=EDGE_CURVE ( 'NONE', #22427, #19657, #213960, .T. ) ;
#33501=DIRECTION ( 'NONE',  ( -0.5994789404140901112, 2.055006554627987857E-15, 0.8003905296791060664 ) ) ;
#33545=CARTESIAN_POINT ( 'NONE',  ( 11.86239285000045918, 9.799999999999997158, -1.812080536912752837 ) ) ;
#33561=CARTESIAN_POINT ( 'NONE',  ( 9.242769546185929386, 14.19339224059835658, 7.653689390903365641 ) ) ;
#33563=CARTESIAN_POINT ( 'NONE',  ( -9.857181934075960328, 5.275265258315555705, 6.218892358987248237 ) ) ;
#33588=CARTESIAN_POINT ( 'NONE',  ( -11.29661021673627097, 7.648989264017080458, 3.919569178588850455 ) ) ;
#33608=FILL_AREA_STYLE_COLOUR ( '', #181507 ) ;
#33638=ORIENTED_EDGE ( 'NONE', *, *, #130663, .T. ) ;
#33645=CARTESIAN_POINT ( 'NONE',  ( -11.33772465723282785, 12.59131699265171989, -3.600000000000076472 ) ) ;
#33665=DIRECTION ( 'NONE',  ( 0.000000000000000000, 1.000000000000000000, 0.000000000000000000 ) ) ;
#33670=VECTOR ( 'NONE', #155016, 1000.000000000000000 ) ;
#33689=MECHANICAL_DESIGN_GEOMETRIC_PRESENTATION_REPRESENTATION('',(#168516),#147821);
#33703=CARTESIAN_POINT ( 'NONE',  ( -11.48243876534946217, 11.29999999999998117, 3.199999999999997957 ) ) ;
#33704=CARTESIAN_POINT ( 'NONE',  ( -10.56511880488638333, 9.841134764184808148, -3.405056808716381944 ) ) ;
#33716=EDGE_LOOP ( 'NONE', ( #196977, #98721, #198718, #150334 ) ) ;
#33757=CARTESIAN_POINT ( 'NONE',  ( 11.78331023100045627, 12.30000000000000071, -1.800000000000001155 ) ) ;
#33788=CARTESIAN_POINT ( 'NONE',  ( -2.224029779570270815, 15.44821792883578127, -11.75514780501742962 ) ) ;
#33792=ORIENTED_EDGE ( 'NONE', *, *, #28655, .T. ) ;
#33821=CARTESIAN_POINT ( 'NONE',  ( -9.367496997601305608, 14.48154074412967596, 7.499999999995371702 ) ) ;
#33826=ORIENTED_EDGE ( 'NONE', *, *, #67738, .T. ) ;
#33849=CARTESIAN_POINT ( 'NONE',  ( 10.16268612673838234, 10.86226847457346167, 8.132478767492923311 ) ) ;
#33851=VERTEX_POINT ( 'NONE', #93214 ) ;
#33862=CARTESIAN_POINT ( 'NONE',  ( -7.119749541375154145, 14.48019291653405105, 9.669933605396591858 ) ) ;
#33901=CARTESIAN_POINT ( 'NONE',  ( -9.410012541129075814, 4.000000000000001776, 6.919867902370715917 ) ) ;
#33905=CARTESIAN_POINT ( 'NONE',  ( 0.000000000000000000, 12.22000000000000064, 0.000000000000000000 ) ) ;
#33931=DIRECTION ( 'NONE',  ( 0.000000000000000000, 1.000000000000000000, 0.000000000000000000 ) ) ;
#33952=CARTESIAN_POINT ( 'NONE',  ( 9.215575659530927055, 13.21669868873661358, -9.027657081567449282 ) ) ;
#33971=COLOUR_RGB ( '', 0.31764706, 0.68627451, 0.89019608) ;
#33991=EDGE_CURVE ( 'NONE', #47282, #75373, #166636, .T. ) ;
#34002=CARTESIAN_POINT ( 'NONE',  ( -9.372156330296117943, 15.41898192430145365, 7.405769077363409281 ) ) ;
#34013=CARTESIAN_POINT ( 'NONE',  ( 11.92619526913699524, 13.52780024161489969, -1.328859060402685976 ) ) ;
#34021=( BOUNDED_SURFACE ( )  B_SPLINE_SURFACE ( 3, 2, ( 
 ( #139609, #137469, #203483 ),
 ( #103892, #169940, #205631 ),
 ( #8505, #171010, #22607 ),
 ( #155840, #55136, #7425 ),
 ( #121281, #88715, #24750 ),
 ( #90852, #72427, #138529 ) ),
 .UNSPECIFIED., .F., .F., .T. ) 
 B_SPLINE_SURFACE_WITH_KNOTS ( ( 4, 2, 4 ),
 ( 3, 3 ),
 ( 0.000000000000000000, 0.0003766405729503175871, 0.0007532811459006351741 ),
 ( 0.000000000000000000, 1.000000000000000000 ),
 .UNSPECIFIED. ) 
 GEOMETRIC_REPRESENTATION_ITEM ( )  RATIONAL_B_SPLINE_SURFACE ( (
 ( 1.000000000000000000, 0.7071067811865551223, 1.000000000000000000),
 ( 1.000000000000000000, 0.7211294902953088171, 1.000000000000000000),
 ( 1.000000000000000000, 0.7311181975231312302, 1.000000000000000000),
 ( 1.000000000000000000, 0.7429553055060466038, 1.000000000000000000),
 ( 1.000000000000000000, 0.7451698531058997821, 1.000000000000000000),
 ( 1.000000000000000000, 0.7452309222763021657, 1.000000000000000000) ) ) 
 REPRESENTATION_ITEM ( '' )  SURFACE ( )  );
#34025=CARTESIAN_POINT ( 'NONE',  ( 11.91826848676359596, 12.59166292761250538, -1.400000051401918855 ) ) ;
#34049=CARTESIAN_POINT ( 'NONE',  ( -0.8947579783427154210, 14.55305220401379174, -11.95586206112747085 ) ) ;
#34072=CARTESIAN_POINT ( 'NONE',  ( -1.500000000000038636, 8.500000000000000000, -10.64483442802187874 ) ) ;
#34074=CIRCLE ( 'NONE', #141278, 0.07999999999999961309 ) ;
#34083=ORIENTED_EDGE ( 'NONE', *, *, #167754, .T. ) ;
#34088=SURFACE_STYLE_FILL_AREA ( #136940 ) ;
#34127=FILL_AREA_STYLE ('',( #203005 ) ) ;
#34157=AXIS2_PLACEMENT_3D ( 'NONE', #164852, #99857, #34832 ) ;
#34178=EDGE_LOOP ( 'NONE', ( #104709, #183409, #164864, #163847 ) ) ;
#34198=SURFACE_STYLE_FILL_AREA ( #198816 ) ;
#34234=CARTESIAN_POINT ( 'NONE',  ( -10.16827420574893814, 6.288608293322982767, 5.589418380748610637 ) ) ;
#34241=B_SPLINE_CURVE_WITH_KNOTS ( 'NONE', 3,
 ( #112670, #180793, #178679, #47628, #144085, #45489 ),
 .UNSPECIFIED., .F., .F.,
 ( 4, 2, 4 ),
 ( 0.000000000000000000, 0.0003155923098472858596, 0.0006311846196945720446 ),
 .UNSPECIFIED. ) ;
#34267=ORIENTED_EDGE ( 'NONE', *, *, #63494, .T. ) ;
#34274=CARTESIAN_POINT ( 'NONE',  ( -15.75000000000000000, 9.799999999999998934, 0.6999999999999992895 ) ) ;
#34275=CARTESIAN_POINT ( 'NONE',  ( 0.000000000000000000, 11.29999999999999893, 0.000000000000000000 ) ) ;
#34286=ADVANCED_FACE ( 'NONE', ( #123652 ), #107370, .F. ) ;
#34331=CARTESIAN_POINT ( 'NONE',  ( -11.60136562008509387, 4.149718911762417584, -5.313756115068398067 ) ) ;
#34332=DIRECTION ( 'NONE',  ( -0.000000000000000000, 1.000000000000000000, 0.000000000000000000 ) ) ;
#34342=CARTESIAN_POINT ( 'NONE',  ( -10.71030397718323890, 6.055815897892919075, -4.668189396100475008 ) ) ;
#34348=CARTESIAN_POINT ( 'NONE',  ( 9.469529551615751828, 11.05767297274606342, 7.376832519613734540 ) ) ;
#34360=CARTESIAN_POINT ( 'NONE',  ( 10.28154365687120908, 8.975950743582902902, -4.140073266697262611 ) ) ;
#34370=CARTESIAN_POINT ( 'NONE',  ( 8.200258344473377647, 14.21219199450433202, -8.700760588951361285 ) ) ;
#34373=ADVANCED_FACE ( 'NONE', ( #2846 ), #56819, .T. ) ;
#34376=CARTESIAN_POINT ( 'NONE',  ( 0.01291932979524827718, 14.54879296676368128, 11.96434918891997157 ) ) ;
#34387=CARTESIAN_POINT ( 'NONE',  ( 1.292128843000387883, 8.373613470998947150, 10.90074592850030122 ) ) ;
#34437=ORIENTED_EDGE ( 'NONE', *, *, #150934, .F. ) ;
#34459=TRIMMED_CURVE ( 'NONE', #166111, ( PARAMETER_VALUE ( 2.245927859731927878 ), #113145 ), ( PARAMETER_VALUE ( 3.141592653589793116 ), #179151 ), .T., .PARAMETER. ) ;
#34470=CARTESIAN_POINT ( 'NONE',  ( -11.95359438121989548, 9.995781002913005864, 1.059536798430472437 ) ) ;
#34503=DIRECTION ( 'NONE',  ( 0.000000000000000000, 0.000000000000000000, -1.000000000000000000 ) ) ;
#34525=CARTESIAN_POINT ( 'NONE',  ( -9.406910906341037659, 15.38274361496693210, -7.349368793364722485 ) ) ;
#34561=SURFACE_STYLE_FILL_AREA ( #54023 ) ;
#34566=CARTESIAN_POINT ( 'NONE',  ( 7.128288838256305660, 14.48195940547645044, 9.656477080921417766 ) ) ;
#34569=CARTESIAN_POINT ( 'NONE',  ( 11.33772463945037146, 19.00000000000000000, 3.679999999999999272 ) ) ;
#34607=CARTESIAN_POINT ( 'NONE',  ( 11.91826848676359241, 10.09166292761251071, -1.400000051401918855 ) ) ;
#34624=CARTESIAN_POINT ( 'NONE',  ( -10.98545788874447915, 13.75743779547922863, 1.592267205258850460 ) ) ;
#34625=CARTESIAN_POINT ( 'NONE',  ( -9.968679514594425584, 5.546356146656833630, 6.001058933476985935 ) ) ;
#34637=ORIENTED_EDGE ( 'NONE', *, *, #85583, .F. ) ;
#34650=CARTESIAN_POINT ( 'NONE',  ( -10.79642412263275908, 6.372378903489562596, 5.136797334115418501 ) ) ;
#34659=ORIENTED_EDGE ( 'NONE', *, *, #178287, .T. ) ;
#34673=DIRECTION ( 'NONE',  ( 0.6249999999999992228, 1.778438476333678106E-14, -0.7806247497998005658 ) ) ;
#34697=( NAMED_UNIT ( * ) PLANE_ANGLE_UNIT ( ) SI_UNIT ( $, .RADIAN. ) );
#34698=CARTESIAN_POINT ( 'NONE',  ( -10.30353590654652862, 3.711604710691488673, 6.155358625546677231 ) ) ;
#34725=FACE_OUTER_BOUND ( 'NONE', #129231, .T. ) ;
#34727=PLANE ( 'NONE',  #201418 ) ;
#34728=PRESENTATION_STYLE_ASSIGNMENT (( #37946 ) ) ;
#34733=FILL_AREA_STYLE_COLOUR ( '', #42214 ) ;
#34739=ORIENTED_EDGE ( 'NONE', *, *, #67181, .T. ) ;
#34758=CARTESIAN_POINT ( 'NONE',  ( -15.75000000000000000, 10.19999999999999929, -0.7000000000000009548 ) ) ;
#34761=CARTESIAN_POINT ( 'NONE',  ( -10.50000000000000000, 10.19999999999999929, -3.600000000000000977 ) ) ;
#34791=CARTESIAN_POINT ( 'NONE',  ( -9.453683584225196057, 15.47105875301949851, -7.391106286260058944 ) ) ;
#34815=FACE_OUTER_BOUND ( 'NONE', #134036, .T. ) ;
#34832=DIRECTION ( 'NONE',  ( 0.000000000000000000, 0.000000000000000000, -1.000000000000000000 ) ) ;
#34842=CARTESIAN_POINT ( 'NONE',  ( -8.749942580429538097, 15.44732705574467779, -8.150331060152165463 ) ) ;
#34843=CARTESIAN_POINT ( 'NONE',  ( -11.41381675112453564, 19.00000000000000000, 3.704697986577180746 ) ) ;
#34845=VERTEX_POINT ( 'NONE', #179012 ) ;
#34858=( BOUNDED_SURFACE ( )  B_SPLINE_SURFACE ( 3, 2, ( 
 ( #105986, #172007, #155757 ),
 ( #139522, #7342, #73419 ),
 ( #189314, #174164, #141678 ),
 ( #46283, #195720, #77692 ),
 ( #177339, #75569, #9497 ),
 ( #191429, #157903, #76623 ) ),
 .UNSPECIFIED., .F., .F., .T. ) 
 B_SPLINE_SURFACE_WITH_KNOTS ( ( 4, 2, 4 ),
 ( 3, 3 ),
 ( 0.000000000000000000, 0.0003754691837024765901, 0.0007509383674049531802 ),
 ( 0.000000000000000000, 1.000000000000000000 ),
 .UNSPECIFIED. ) 
 GEOMETRIC_REPRESENTATION_ITEM ( )  RATIONAL_B_SPLINE_SURFACE ( (
 ( 1.000000000000000000, 0.6711954675835395401, 1.000000000000000000),
 ( 1.000000000000000000, 0.6709646295267452931, 1.000000000000000000),
 ( 1.000000000000000000, 0.6771840716659260906, 1.000000000000000000),
 ( 1.000000000000000000, 0.6927481755867372915, 1.000000000000000000),
 ( 1.000000000000000000, 0.7017972101309932764, 1.000000000000000000),
 ( 1.000000000000000000, 0.7071067811865475727, 1.000000000000000000) ) ) 
 REPRESENTATION_ITEM ( '' )  SURFACE ( )  );
#34871=CARTESIAN_POINT ( 'NONE',  ( 0.000000000000000000, 14.48154074412737202, -12.00000000000000178 ) ) ;
#34878=ORIENTED_EDGE ( 'NONE', *, *, #181087, .T. ) ;
#34892=CARTESIAN_POINT ( 'NONE',  ( -12.76460961864369814, 7.407083900356914441, 2.164514475593080078 ) ) ;
#34894=DIRECTION ( 'NONE',  ( -0.2684563758389253985, 0.000000000000000000, 0.9632918427306595976 ) ) ;
#34921=CARTESIAN_POINT ( 'NONE',  ( 11.94650005372638013, 12.44897299662361867, -1.135399707157281890 ) ) ;
#34941=EDGE_CURVE ( 'NONE', #139957, #91093, #93248, .T. ) ;
#34957=CARTESIAN_POINT ( 'NONE',  ( -9.420111044277531320, 2.999985932080179829, -6.906458289183190047 ) ) ;
#34963=CARTESIAN_POINT ( 'NONE',  ( -11.86580791720155226, 7.723834678533566311, 1.807467791464186346 ) ) ;
#34980=CIRCLE ( 'NONE', #156071, 0.07999999999999998779 ) ;
#35007=CARTESIAN_POINT ( 'NONE',  ( 8.329933198152533080, 13.18708556817446009, -8.542943463288903416 ) ) ;
#35015=EDGE_CURVE ( 'NONE', #74053, #47282, #210605, .T. ) ;
#35024=CARTESIAN_POINT ( 'NONE',  ( 11.84668729035180590, 13.50518580017410564, -1.400000000000001688 ) ) ;
#35037=EDGE_CURVE ( 'NONE', #105457, #168364, #86454, .T. ) ;
#35041=( GEOMETRIC_REPRESENTATION_CONTEXT ( 3 ) GLOBAL_UNCERTAINTY_ASSIGNED_CONTEXT ( ( #62997 ) ) GLOBAL_UNIT_ASSIGNED_CONTEXT ( ( #177344, #196782, #21992 ) ) REPRESENTATION_CONTEXT ( 'NONE', 'WORKASPACE' ) );
#35067=CARTESIAN_POINT ( 'NONE',  ( 11.92619526913699879, 13.40000000000000036, -1.328859060402686199 ) ) ;
#35070=CIRCLE ( 'NONE', #3972, 0.07999999999999933553 ) ;
#35072=CARTESIAN_POINT ( 'NONE',  ( -9.367496997601300279, 15.00000000000599343, 7.499999999995378808 ) ) ;
#35088=EDGE_CURVE ( 'NONE', #128985, #116165, #35956, .T. ) ;
#35112=CARTESIAN_POINT ( 'NONE',  ( 11.04536101718726293, 10.19999999999999929, -1.100000000000000311 ) ) ;
#35115=CARTESIAN_POINT ( 'NONE',  ( -11.89197369110779867, 11.30000000000000071, 0.8056055387119849254 ) ) ;
#35130=VERTEX_POINT ( 'NONE', #108475 ) ;
#35131=COLOUR_RGB ( '', 0.09019608, 0.27058824, 0.51372549) ;
#35147=EDGE_CURVE ( 'NONE', #197638, #75373, #158811, .T. ) ;
#35165=EDGE_LOOP ( 'NONE', ( #60632, #106617, #172327, #38721 ) ) ;
#35170=DIRECTION ( 'NONE',  ( -0.000000000000000000, 1.000000000000000000, -0.000000000000000000 ) ) ;
#35207=DIRECTION ( 'NONE',  ( 0.000000000000000000, 0.000000000000000000, 1.000000000000000000 ) ) ;
#35211=COLOUR_RGB ( '', 0.09019608, 0.27058824, 0.51372549) ;
#35236=ORIENTED_EDGE ( 'NONE', *, *, #84119, .F. ) ;
#35240=CARTESIAN_POINT ( 'NONE',  ( -11.78331023100045449, 13.79999999999998295, 1.799999999999999600 ) ) ;
#35242=CARTESIAN_POINT ( 'NONE',  ( -11.00595142344305444, 13.60990418661507739, -1.443824005414911182 ) ) ;
#35287=COLOUR_RGB ( '', 0.09019608, 0.27058824, 0.51372549) ;
#35293=CARTESIAN_POINT ( 'NONE',  ( -10.01593736600300311, 5.734280347462529015, 5.906528988732270058 ) ) ;
#35320=ORIENTED_EDGE ( 'NONE', *, *, #64280, .F. ) ;
#35321=UNCERTAINTY_MEASURE_WITH_UNIT (LENGTH_MEASURE( 1.000000000000000082E-05 ), #119191, 'distance_accuracy_value', 'NONE');
#35328=VECTOR ( 'NONE', #184060, 1000.000000000000000 ) ;
#35333=SURFACE_SIDE_STYLE ('',( #144884 ) ) ;
#35345=EDGE_CURVE ( 'NONE', #40498, #19959, #197696, .T. ) ;
#35349=TOROIDAL_SURFACE ( 'NONE', #212232, 11.92000000000000171, 0.08000000000000000167 ) ;
#35395=CARTESIAN_POINT ( 'NONE',  ( -11.16206481669071415, 4.728763190537430994, -6.013947724923736082 ) ) ;
#35406=DIRECTION ( 'NONE',  ( 0.000000000000000000, 0.000000000000000000, -1.000000000000000000 ) ) ;
#35413=CARTESIAN_POINT ( 'NONE',  ( 9.443127104094640956, 11.07005408922290002, 7.334139569562794669 ) ) ;
#35425=CARTESIAN_POINT ( 'NONE',  ( 10.74389548477261691, 10.91622383494151549, 5.684367872889470874 ) ) ;
#35433=VECTOR ( 'NONE', #193073, 1000.000000000000000 ) ;
#35437=CARTESIAN_POINT ( 'NONE',  ( 7.958945746774230834, 14.27980018522660188, -8.981532223576218499 ) ) ;
#35438=CARTESIAN_POINT ( 'NONE',  ( -7.116813477139661615, 15.47012847482234221, -9.672254489698197233 ) ) ;
#35452=DIRECTION ( 'NONE',  ( 1.000000000000000000, -0.000000000000000000, -0.000000000000000000 ) ) ;
#35480=FACE_OUTER_BOUND ( 'NONE', #91276, .T. ) ;
#35498=AXIS2_PLACEMENT_3D ( 'NONE', #142902, #107229, #40039 ) ;
#35499=LINE ( 'NONE', #184939, #134482 ) ;
#35534=CARTESIAN_POINT ( 'NONE',  ( -11.97178994924802353, 9.720000062027946086, 0.8322011300497191844 ) ) ;
#35548=CARTESIAN_POINT ( 'NONE',  ( 11.45842088241076340, 12.50693529122958481, 3.566211699757793063 ) ) ;
#35568=ADVANCED_FACE ( 'NONE', ( #145231 ), #63932, .F. ) ;
#35591=AXIS2_PLACEMENT_3D ( 'NONE', #3408, #120465, #102004 ) ;
#35605=CARTESIAN_POINT ( 'NONE',  ( 11.33772463945037146, 13.39999999999998259, 3.599999999999999201 ) ) ;
#35683=ORIENTED_EDGE ( 'NONE', *, *, #4802, .F. ) ;
#35686=CARTESIAN_POINT ( 'NONE',  ( 7.903135977162644821, 15.38542563725095746, 9.031658180448362216 ) ) ;
#35688=CARTESIAN_POINT ( 'NONE',  ( -9.505648412044632067, 5.017053549588888828, 6.783778555801666776 ) ) ;
#35712=CARTESIAN_POINT ( 'NONE',  ( -11.77172135380034490, 8.649151653032827625, -2.103707379449156978 ) ) ;
#35732=SURFACE_STYLE_USAGE ( .BOTH. , #119185 ) ;
#35745=CARTESIAN_POINT ( 'NONE',  ( -11.04536101718726293, 10.19999999999999929, -1.100000000000000311 ) ) ;
#35766=( LENGTH_UNIT ( ) NAMED_UNIT ( * ) SI_UNIT ( .MILLI., .METRE. ) );
#35767=CARTESIAN_POINT ( 'NONE',  ( -10.66822795754452358, 4.187511268866498604, 5.495200216426709083 ) ) ;
#35775=CARTESIAN_POINT ( 'NONE',  ( -11.43190902327450509, 12.44477871742144615, -3.649704988378223991 ) ) ;
#35798=FILL_AREA_STYLE_COLOUR ( '', #38802 ) ;
#35834=CARTESIAN_POINT ( 'NONE',  ( -10.43230948805442893, 5.066484524551064794, 5.254757398418679060 ) ) ;
#35851=ORIENTED_EDGE ( 'NONE', *, *, #57578, .T. ) ;
#35890=DIRECTION ( 'NONE',  ( 1.224646799147343346E-16, 0.000000000000000000, -1.000000000000000000 ) ) ;
#35892=CARTESIAN_POINT ( 'NONE',  ( -11.89321938400721379, 12.33744721639341968, -1.599605898944043147 ) ) ;
#35895=CARTESIAN_POINT ( 'NONE',  ( 0.000000000000000000, 3.553060279300588320, 0.000000000000000000 ) ) ;
#35908=FACE_OUTER_BOUND ( 'NONE', #174816, .T. ) ;
#35945=EDGE_LOOP ( 'NONE', ( #44368, #22160, #30144, #10362 ) ) ;
#35949=CARTESIAN_POINT ( 'NONE',  ( -11.33772463945036968, 12.69999999999999929, -3.600000000000000977 ) ) ;
#35956=( BOUNDED_CURVE ( )  B_SPLINE_CURVE ( 3, ( #10881, #161436, #42364, #43425 ),
 .UNSPECIFIED., .F., .T. ) 
 B_SPLINE_CURVE_WITH_KNOTS ( ( 4, 4 ),
 ( 1.430804639040424098, 1.438015327900962204 ),
 .UNSPECIFIED. ) 
 CURVE ( )  GEOMETRIC_REPRESENTATION_ITEM ( )  RATIONAL_B_SPLINE_CURVE ( ( 1.000000000000000000, 0.9999956671685397147, 0.9999956671685397147, 1.000000000000000000 ) ) 
 REPRESENTATION_ITEM ( '' )  );
#35959=ORIENTED_EDGE ( 'NONE', *, *, #79134, .T. ) ;
#35970=CARTESIAN_POINT ( 'NONE',  ( -11.34342368903357290, 5.311043228906556557, 5.661199053045820051 ) ) ;
#35972=DIRECTION ( 'NONE',  ( 1.000000000000000000, -0.000000000000000000, -0.000000000000000000 ) ) ;
#35998=CARTESIAN_POINT ( 'NONE',  ( -15.75000000000000000, 13.40000000000000036, -3.600000000000002309 ) ) ;
#36024=EDGE_LOOP ( 'NONE', ( #45358, #201417, #178768, #75697 ) ) ;
#36029=CARTESIAN_POINT ( 'NONE',  ( 11.04536101718726293, 12.59537905954598358, 1.099999999999999201 ) ) ;
#36038=DIRECTION ( 'NONE',  ( 0.8003905289055504024, -4.396526966619893387E-05, 0.5994789398347104559 ) ) ;
#36074=CARTESIAN_POINT ( 'NONE',  ( 0.000000000000000000, 13.79999999999998295, 0.000000000000000000 ) ) ;
#36077=CARTESIAN_POINT ( 'NONE',  ( 7.948861177221683505, 14.94981965669310853, -9.879624537148666619 ) ) ;
#36092=CARTESIAN_POINT ( 'NONE',  ( 11.92619525870751573, 13.52622296793681045, -1.328859154004804699 ) ) ;
#36106=EDGE_CURVE ( 'NONE', #123196, #181120, #157024, .T. ) ;
#36112=MECHANICAL_DESIGN_GEOMETRIC_PRESENTATION_REPRESENTATION('',(#198748),#105424);
#36137=CARTESIAN_POINT ( 'NONE',  ( 11.86145016429273014, 11.00587876334730453, -1.100000000000000089 ) ) ;
#36144=DIRECTION ( 'NONE',  ( 0.1959619652057391359, -0.8823239151465414043, -0.4279058505713422278 ) ) ;
#36147=CARTESIAN_POINT ( 'NONE',  ( 11.91292854676703961, 12.48518470326975560, -1.446370920797349635 ) ) ;
#36175=VECTOR ( 'NONE', #149991, 1000.000000000000000 ) ;
#36193=CARTESIAN_POINT ( 'NONE',  ( -10.64390791476601450, 5.929706677703244111, 5.549313566458391911 ) ) ;
#36198=EDGE_LOOP ( 'NONE', ( #49993, #170987, #190985, #200747 ) ) ;
#36221=ORIENTED_EDGE ( 'NONE', *, *, #12435, .F. ) ;
#36225=VERTEX_POINT ( 'NONE', #102836 ) ;
#36230=ADVANCED_FACE ( 'NONE', ( #152645 ), #124604, .T. ) ;
#36238=CARTESIAN_POINT ( 'NONE',  ( -0.02237740007485569671, 15.46059968838234866, 11.97522600859444353 ) ) ;
#36249=ADVANCED_FACE ( 'NONE', ( #139624, #169954 ), #87653, .T. ) ;
#36251=CIRCLE ( 'NONE', #18929, 0.5000000000000016653 ) ;
#36293=ORIENTED_EDGE ( 'NONE', *, *, #8528, .F. ) ;
#36309=SURFACE_SIDE_STYLE ('',( #70927 ) ) ;
#36316=( GEOMETRIC_REPRESENTATION_CONTEXT ( 3 ) GLOBAL_UNCERTAINTY_ASSIGNED_CONTEXT ( ( #55301 ) ) GLOBAL_UNIT_ASSIGNED_CONTEXT ( ( #165748, #63985, #17334 ) ) REPRESENTATION_CONTEXT ( 'NONE', 'WORKASPACE' ) );
#36324=DIRECTION ( 'NONE',  ( 0.000000000000000000, 0.000000000000000000, -1.000000000000000000 ) ) ;
#36332=CARTESIAN_POINT ( 'NONE',  ( -10.50000000000000000, 10.89999999999998259, 3.599999999999999201 ) ) ;
#36357=CARTESIAN_POINT ( 'NONE',  ( 0.3263184169968956772, 16.00000000000087397, -11.67999999558625213 ) ) ;
#36359=CARTESIAN_POINT ( 'NONE',  ( -10.16814981310353616, 6.288261174334121684, -5.589887627215723853 ) ) ;
#36362=ADVANCED_FACE ( 'NONE', ( #25830 ), #85931, .F. ) ;
#36395=VECTOR ( 'NONE', #201583, 1000.000000000000000 ) ;
#36403=CARTESIAN_POINT ( 'NONE',  ( 0.000000000000000000, 13.79999999999999893, 0.000000000000000000 ) ) ;
#36432=ORIENTED_EDGE ( 'NONE', *, *, #149426, .F. ) ;
#36438=CARTESIAN_POINT ( 'NONE',  ( 11.94105721237523277, 10.07259215598211100, 1.187919463087244720 ) ) ;
#36468=CARTESIAN_POINT ( 'NONE',  ( -10.76260246389097297, 4.190717020667873882, -6.707086991120802644 ) ) ;
#36479=CARTESIAN_POINT ( 'NONE',  ( -10.52284260640670688, 5.420240069097000735, -5.071998063130033430 ) ) ;
#36484=CARTESIAN_POINT ( 'NONE',  ( 11.09412727165957691, 8.002531996343789089, 4.594739555395619846 ) ) ;
#36493=ORIENTED_EDGE ( 'NONE', *, *, #69678, .T. ) ;
#36495=CARTESIAN_POINT ( 'NONE',  ( 9.379604873787226182, 12.64221115367513626, 6.544017673515419631 ) ) ;
#36507=CARTESIAN_POINT ( 'NONE',  ( -5.600682685854159182, 15.51843887179352244, -10.62222670599373764 ) ) ;
#36534=CARTESIAN_POINT ( 'NONE',  ( -9.404907904283509978, 14.48154074430288851, -7.453273792521815544 ) ) ;
#36607=EDGE_LOOP ( 'NONE', ( #117413, #46676, #156208, #154426 ) ) ;
#36612=FILL_AREA_STYLE ('',( #151455 ) ) ;
#36620=STYLED_ITEM ( 'NONE', ( #183053 ), #7322 ) ;
#36634=CARTESIAN_POINT ( 'NONE',  ( -11.86145016429273724, 13.50587408513255738, -1.100000000000002531 ) ) ;
#36636=DIRECTION ( 'NONE',  ( -0.000000000000000000, -1.000000000000000000, -0.000000000000000000 ) ) ;
#36646=CARTESIAN_POINT ( 'NONE',  ( 11.94105721237523277, 13.40000000000000036, 1.187919463087248273 ) ) ;
#36664=DIRECTION ( 'NONE',  ( 1.000000000000000000, 0.000000000000000000, -3.706092522800016599E-15 ) ) ;
#36666=CARTESIAN_POINT ( 'NONE',  ( -15.75000000000000000, 10.90000000000000036, 0.6999999999999992895 ) ) ;
#36670=CARTESIAN_POINT ( 'NONE',  ( 11.49966000274946509, 13.74232845564725558, 3.429881629453341851 ) ) ;
#36673=EDGE_CURVE ( 'NONE', #94599, #172216, #169168, .T. ) ;
#36680=ADVANCED_FACE ( 'NONE', ( #156158 ), #101098, .T. ) ;
#36689=CARTESIAN_POINT ( 'NONE',  ( 1.734723475976807094E-15, 15.00041888085534758, 12.17999951260719982 ) ) ;
#36721=CIRCLE ( 'NONE', #157818, 12.00000000000000178 ) ;
#36749=CARTESIAN_POINT ( 'NONE',  ( 9.427850895902817996, 13.54474674066948481, 7.423989997610750180 ) ) ;
#36751=CARTESIAN_POINT ( 'NONE',  ( -9.811677024507259759, 4.107325997343203028, 6.339424533126782002 ) ) ;
#36756=CIRCLE ( 'NONE', #67810, 0.5000000000000013323 ) ;
#36762=ORIENTED_EDGE ( 'NONE', *, *, #151886, .T. ) ;
#36763=( GEOMETRIC_REPRESENTATION_CONTEXT ( 3 ) GLOBAL_UNCERTAINTY_ASSIGNED_CONTEXT ( ( #206865 ) ) GLOBAL_UNIT_ASSIGNED_CONTEXT ( ( #5118, #123279, #104810 ) ) REPRESENTATION_CONTEXT ( 'NONE', 'WORKASPACE' ) );
#36774=DIRECTION ( 'NONE',  ( 0.000000000000000000, -1.000000000000000000, 0.000000000000000000 ) ) ;
#36781=DIRECTION ( 'NONE',  ( 0.000000000000000000, -1.000000000000000000, -9.023263958591317418E-17 ) ) ;
#36790=CARTESIAN_POINT ( 'NONE',  ( 11.89829993707161471, 11.32919228251124366, 1.561606677374347329 ) ) ;
#36799=ORIENTED_EDGE ( 'NONE', *, *, #156430, .T. ) ;
#36802=LINE ( 'NONE', #101814, #200108 ) ;
#36806=CARTESIAN_POINT ( 'NONE',  ( -11.04986227068298277, 9.990600021556637955, -1.056429153205399984 ) ) ;
#36827=SURFACE_STYLE_FILL_AREA ( #148475 ) ;
#36828=CARTESIAN_POINT ( 'NONE',  ( 10.95308175811721085, 13.79999999999998295, 1.799999999999999600 ) ) ;
#36829=DIRECTION ( 'NONE',  ( -0.000000000000000000, -1.000000000000000000, -0.000000000000000000 ) ) ;
#36831=CARTESIAN_POINT ( 'NONE',  ( -11.84668730067608600, 13.40000000000000036, -1.400000000000001910 ) ) ;
#36861=CARTESIAN_POINT ( 'NONE',  ( -15.75000000000000000, 13.40000000000000036, 0.6999999999999992895 ) ) ;
#36873=AXIS2_PLACEMENT_3D ( 'NONE', #131496, #197500, #44891 ) ;
#36898=CARTESIAN_POINT ( 'NONE',  ( -10.20579153398542616, 5.000000000000003553, 7.525503907114123869 ) ) ;
#36899=VERTEX_POINT ( 'NONE', #114916 ) ;
#36911=ORIENTED_EDGE ( 'NONE', *, *, #58073, .F. ) ;
#36927=( GEOMETRIC_REPRESENTATION_CONTEXT ( 3 ) GLOBAL_UNCERTAINTY_ASSIGNED_CONTEXT ( ( #185278 ) ) GLOBAL_UNIT_ASSIGNED_CONTEXT ( ( #107039, #20381, #137366 ) ) REPRESENTATION_CONTEXT ( 'NONE', 'WORKASPACE' ) );
#36950=ORIENTED_EDGE ( 'NONE', *, *, #184582, .T. ) ;
#36960=CARTESIAN_POINT ( 'NONE',  ( -11.92619525870750508, 12.57377703206319808, -1.328859154004902621 ) ) ;
#37032=CARTESIAN_POINT ( 'NONE',  ( -10.45142682343936791, 5.144546645612242841, 5.216777551074719632 ) ) ;
#37035=DIRECTION ( 'NONE',  ( 1.000000000000000000, -0.000000000000000000, -0.000000000000000000 ) ) ;
#37049=ORIENTED_EDGE ( 'NONE', *, *, #123836, .F. ) ;
#37065=VECTOR ( 'NONE', #4372, 1000.000000000000000 ) ;
#37094=ORIENTED_EDGE ( 'NONE', *, *, #207217, .F. ) ;
#37101=DIRECTION ( 'NONE',  ( 1.000000000000000000, -0.000000000000000000, -0.000000000000000000 ) ) ;
#37102=CARTESIAN_POINT ( 'NONE',  ( -10.39320420135713263, 4.932286138528427344, 5.331284845095887626 ) ) ;
#37150=CARTESIAN_POINT ( 'NONE',  ( 8.299603047032746872, 13.24802564661077575, -8.551073489896891644 ) ) ;
#37173=VERTEX_POINT ( 'NONE', #103942 ) ;
#37184=CARTESIAN_POINT ( 'NONE',  ( -10.48266952940149466, 5.268049057482275366, -5.154014898524191146 ) ) ;
#37187=CARTESIAN_POINT ( 'NONE',  ( 8.665224416106017458, 14.86907450242385309, -8.237936485434854461 ) ) ;
#37200=ORIENTED_EDGE ( 'NONE', *, *, #190444, .F. ) ;
#37205=CARTESIAN_POINT ( 'NONE',  ( 9.319154265906131940, 13.69453762107142225, 7.487145396731793134 ) ) ;
#37206=CARTESIAN_POINT ( 'NONE',  ( -11.86239285000045918, 13.87999999999998302, 1.812080536912751061 ) ) ;
#37210=DIRECTION ( 'NONE',  ( -0.000000000000000000, -1.000000000000000000, -0.000000000000000000 ) ) ;
#37228=FACE_OUTER_BOUND ( 'NONE', #69975, .T. ) ;
#37236=AXIS2_PLACEMENT_3D ( 'NONE', #157163, #8754, #127947 ) ;
#37255=CARTESIAN_POINT ( 'NONE',  ( 11.33772463945037146, 10.89999999999998259, 3.599999999999999201 ) ) ;
#37278=ORIENTED_EDGE ( 'NONE', *, *, #137200, .T. ) ;
#37302=DIRECTION ( 'NONE',  ( 0.000000000000000000, 0.000000000000000000, 1.000000000000000000 ) ) ;
#37316=CARTESIAN_POINT ( 'NONE',  ( -0.05740707158673791916, 15.49542554636510339, 11.99731162103223525 ) ) ;
#37325=SURFACE_SIDE_STYLE ('',( #54645 ) ) ;
#37327=EDGE_CURVE ( 'NONE', #155586, #195844, #94874, .T. ) ;
#37334=CIRCLE ( 'NONE', #158420, 0.5000000000000004441 ) ;
#37362=AXIS2_PLACEMENT_3D ( 'NONE', #107032, #173058, #75543 ) ;
#37368=EDGE_LOOP ( 'NONE', ( #47876, #84195, #192, #37905 ) ) ;
#37383=DIRECTION ( 'NONE',  ( 0.000000000000000000, 1.000000000000000000, 0.000000000000000000 ) ) ;
#37434=COLOUR_RGB ( '', 0.31764706, 0.68627451, 0.89019608) ;
#37436=CARTESIAN_POINT ( 'NONE',  ( -10.71030397718323890, 6.055815897892919075, -4.668189396100475008 ) ) ;
#37446=ORIENTED_EDGE ( 'NONE', *, *, #163845, .T. ) ;
#37465=PRESENTATION_STYLE_ASSIGNMENT (( #185834 ) ) ;
#37475=FILL_AREA_STYLE ('',( #119864 ) ) ;
#37534=VERTEX_POINT ( 'NONE', #156958 ) ;
#37542=CARTESIAN_POINT ( 'NONE',  ( -10.12724049293007766, 3.240713040256745003, -5.870485300885818880 ) ) ;
#37543=FACE_OUTER_BOUND ( 'NONE', #206984, .T. ) ;
#37552=CARTESIAN_POINT ( 'NONE',  ( -10.57232898948313604, 5.599354254162436817, 4.968808419985093039 ) ) ;
#37558=CARTESIAN_POINT ( 'NONE',  ( 11.83847906649667436, 6.805419798594589231, -1.976859043548241823 ) ) ;
#37563=VERTEX_POINT ( 'NONE', #26925 ) ;
#37569=CARTESIAN_POINT ( 'NONE',  ( -11.07790593930098311, 13.79999999999999893, -0.7000000000000009548 ) ) ;
#37570=CARTESIAN_POINT ( 'NONE',  ( 8.916922505737264970, 12.80282292485108186, 7.559592800977426919 ) ) ;
#37581=CARTESIAN_POINT ( 'NONE',  ( -4.795807126352183758, 15.46909917608900109, -11.00906995846085223 ) ) ;
#37596=CARTESIAN_POINT ( 'NONE',  ( -10.49167095263961613, 5.343775707538777731, -5.730694126968513658 ) ) ;
#37600=EDGE_CURVE ( 'NONE', #83422, #97605, #136311, .T. ) ;
#37613=( LENGTH_UNIT ( ) NAMED_UNIT ( * ) SI_UNIT ( .MILLI., .METRE. ) );
#37630=( GEOMETRIC_REPRESENTATION_CONTEXT ( 3 ) GLOBAL_UNCERTAINTY_ASSIGNED_CONTEXT ( ( #120084 ) ) GLOBAL_UNIT_ASSIGNED_CONTEXT ( ( #114427, #199847, #133836 ) ) REPRESENTATION_CONTEXT ( 'NONE', 'WORKASPACE' ) );
#37661=EDGE_CURVE ( 'NONE', #76787, #123444, #168841, .T. ) ;
#37690=ORIENTED_EDGE ( 'NONE', *, *, #143656, .T. ) ;
#37703=CIRCLE ( 'NONE', #141498, 11.09999999999999964 ) ;
#37725=DIRECTION ( 'NONE',  ( 0.000000000000000000, 0.000000000000000000, 1.000000000000000000 ) ) ;
#37763=EDGE_CURVE ( 'NONE', #108500, #16927, #79336, .T. ) ;
#37826=VERTEX_POINT ( 'NONE', #139691 ) ;
#37830=CARTESIAN_POINT ( 'NONE',  ( 9.704905176613070950, 13.32621205788646002, -8.135614888031417635 ) ) ;
#37832=CARTESIAN_POINT ( 'NONE',  ( -10.44369227015510404, 5.112964020592959180, 5.232143560358712087 ) ) ;
#37868=VERTEX_POINT ( 'NONE', #140768 ) ;
#37875=DIRECTION ( 'NONE',  ( 0.000000000000000000, 0.000000000000000000, -1.000000000000000000 ) ) ;
#37881=ORIENTED_EDGE ( 'NONE', *, *, #150934, .T. ) ;
#37901=DIRECTION ( 'NONE',  ( 0.000000000000000000, 9.023263958591318651E-17, -1.000000000000000000 ) ) ;
#37905=ORIENTED_EDGE ( 'NONE', *, *, #2431, .F. ) ;
#37912=ORIENTED_EDGE ( 'NONE', *, *, #74682, .T. ) ;
#37923=ORIENTED_EDGE ( 'NONE', *, *, #178754, .F. ) ;
#37932=CARTESIAN_POINT ( 'NONE',  ( -9.333041836230014709, 15.44694763438214302, 7.472413793098208856 ) ) ;
#37942=CARTESIAN_POINT ( 'NONE',  ( 11.92619526913699879, 13.40000000000000036, -1.328859060402686199 ) ) ;
#37946=SURFACE_STYLE_USAGE ( .BOTH. , #166886 ) ;
#37980=CARTESIAN_POINT ( 'NONE',  ( -11.25356361929547688, 4.972433335311166935, 5.839389443199928920 ) ) ;
#37994=VERTEX_POINT ( 'NONE', #42184 ) ;
#37995=ORIENTED_EDGE ( 'NONE', *, *, #204332, .F. ) ;
#38002=CARTESIAN_POINT ( 'NONE',  ( -0.005207807541490402925, 15.44298311167088755, 11.94812393301963915 ) ) ;
#38011=CARTESIAN_POINT ( 'NONE',  ( -9.421119846345563431, 14.56525804660669898, -7.432612890530830185 ) ) ;
#38039=CARTESIAN_POINT ( 'NONE',  ( 11.84668729035180590, 12.59481419982586914, 1.399999999999998357 ) ) ;
#38058=ORIENTED_EDGE ( 'NONE', *, *, #89670, .T. ) ;
#38076=ORIENTED_EDGE ( 'NONE', *, *, #175553, .F. ) ;
#38104=AXIS2_PLACEMENT_3D ( 'NONE', #64329, #195400, #63255 ) ;
#38177=ADVANCED_FACE ( 'NONE', ( #75813 ), #58620, .T. ) ;
#38210=SURFACE_STYLE_USAGE ( .BOTH. , #149836 ) ;
#38227=CARTESIAN_POINT ( 'NONE',  ( 8.255390768298678239, 13.81349006448566996, -9.579378744720992600 ) ) ;
#38234=EDGE_LOOP ( 'NONE', ( #4085, #133702, #206823, #64106 ) ) ;
#38244=CARTESIAN_POINT ( 'NONE',  ( 11.43204722947019825, 9.944072459738245939, 3.649275849833181429 ) ) ;
#38276=CARTESIAN_POINT ( 'NONE',  ( 9.167018891879168407, 14.15818339566316908, 7.673511198540157174 ) ) ;
#38277=CARTESIAN_POINT ( 'NONE',  ( -9.497949338412174924, 15.41976506893289134, 7.334250928090418675 ) ) ;
#38281=FILL_AREA_STYLE_COLOUR ( '', #161727 ) ;
#38287=CARTESIAN_POINT ( 'NONE',  ( 11.97302537858606897, 13.79875989808017778, -0.8111997896467577629 ) ) ;
#38323=LINE ( 'NONE', #37255, #97546 ) ;
#38371=CARTESIAN_POINT ( 'NONE',  ( -11.48784849554596121, 9.769504728180656628, -3.469614872287748231 ) ) ;
#38391=CIRCLE ( 'NONE', #3879, 11.09999999999999964 ) ;
#38395=AXIS2_PLACEMENT_3D ( 'NONE', #70239, #19368, #133173 ) ;
#38396=CARTESIAN_POINT ( 'NONE',  ( -11.56018411499319853, 8.213217331593577697, 3.229764516336100399 ) ) ;
#38413=ADVANCED_FACE ( 'NONE', ( #204753 ), #20754, .T. ) ;
#38430=DIRECTION ( 'NONE',  ( 0.000000000000000000, 0.000000000000000000, -1.000000000000000000 ) ) ;
#38452=EDGE_CURVE ( 'NONE', #31691, #124513, #207343, .T. ) ;
#38470=CARTESIAN_POINT ( 'NONE',  ( 9.367496997597600128, 3.999999999999994671, 7.500000000000004441 ) ) ;
#38477=( LENGTH_UNIT ( ) NAMED_UNIT ( * ) SI_UNIT ( .MILLI., .METRE. ) );
#38510=CARTESIAN_POINT ( 'NONE',  ( -10.48267169704037727, 5.268073273308885973, 5.153989745587932880 ) ) ;
#38533=ORIENTED_EDGE ( 'NONE', *, *, #194571, .T. ) ;
#38617=CARTESIAN_POINT ( 'NONE',  ( -11.19531657929523583, 4.806608400964729633, -5.951317567608690240 ) ) ;
#38621=EDGE_LOOP ( 'NONE', ( #204291, #58740, #185288, #207827 ) ) ;
#38628=CARTESIAN_POINT ( 'NONE',  ( -10.50660484223216606, 5.359830900411396648, 5.105327592218940502 ) ) ;
#38634=CARTESIAN_POINT ( 'NONE',  ( 11.39089125540332148, 7.472230595314081292, 3.799964780113331830 ) ) ;
#38646=MECHANICAL_DESIGN_GEOMETRIC_PRESENTATION_REPRESENTATION('',(#4134),#10952);
#38658=EDGE_LOOP ( 'NONE', ( #52487, #153062, #209789, #9955, #196764, #38533 ) ) ;
#38670=FILL_AREA_STYLE ('',( #84208 ) ) ;
#38679=ORIENTED_EDGE ( 'NONE', *, *, #121920, .F. ) ;
#38703=DIRECTION ( 'NONE',  ( 0.000000000000000000, -9.023263958591316185E-17, 1.000000000000000000 ) ) ;
#38704=CARTESIAN_POINT ( 'NONE',  ( -11.16206481669071415, 4.728763190537430994, -6.013947724923736082 ) ) ;
#38721=ORIENTED_EDGE ( 'NONE', *, *, #59183, .F. ) ;
#38744=B_SPLINE_CURVE_WITH_KNOTS ( 'NONE', 3,
 ( #189860, #158439, #76114, #139003, #8977, #208232 ),
 .UNSPECIFIED., .F., .F.,
 ( 4, 2, 4 ),
 ( 0.000000000000000000, 0.0003172254002810710651, 0.0006344508005621421302 ),
 .UNSPECIFIED. ) ;
#38759=ORIENTED_EDGE ( 'NONE', *, *, #21974, .T. ) ;
#38771=CIRCLE ( 'NONE', #101060, 0.08000000000000020983 ) ;
#38783=SURFACE_STYLE_USAGE ( .BOTH. , #57167 ) ;
#38802=COLOUR_RGB ( '', 0.09019608, 0.27058824, 0.51372549) ;
#38822=CARTESIAN_POINT ( 'NONE',  ( 11.41381678389397614, 13.52879418241072074, 3.704697885617693753 ) ) ;
#38838=CARTESIAN_POINT ( 'NONE',  ( 9.367496997597598352, 4.518459255872631530, -7.500000000000005329 ) ) ;
#38864=ORIENTED_EDGE ( 'NONE', *, *, #171794, .F. ) ;
#38882=DIRECTION ( 'NONE',  ( -0.000000000000000000, -1.000000000000000000, -0.000000000000000000 ) ) ;
#38884=DIRECTION ( 'NONE',  ( -0.000000000000000000, -1.000000000000000000, -0.000000000000000000 ) ) ;
#38896=ORIENTED_EDGE ( 'NONE', *, *, #208458, .T. ) ;
#38899=( NAMED_UNIT ( * ) PLANE_ANGLE_UNIT ( ) SI_UNIT ( $, .RADIAN. ) );
#38901=CARTESIAN_POINT ( 'NONE',  ( -10.82858503610327894, 5.585649091226504659, 6.509997993261127824 ) ) ;
#38930=CARTESIAN_POINT ( 'NONE',  ( -4.385389099566589621, 14.48107117044276571, 11.17888682965734937 ) ) ;
#38932=ORIENTED_EDGE ( 'NONE', *, *, #169477, .F. ) ;
#38949=ORIENTED_EDGE ( 'NONE', *, *, #27652, .T. ) ;
#38956=CARTESIAN_POINT ( 'NONE',  ( 6.902720145097976712, 15.44736672593543148, 9.761920446463514978 ) ) ;
#38967=DIRECTION ( 'NONE',  ( 1.000000000000000000, -0.000000000000000000, 1.224646799147353207E-16 ) ) ;
#38970=CARTESIAN_POINT ( 'NONE',  ( -11.89204169242383102, 11.29999999999999893, 0.8046421800351404308 ) ) ;
#39009=ORIENTED_EDGE ( 'NONE', *, *, #29854, .F. ) ;
#39015=CARTESIAN_POINT ( 'NONE',  ( 11.28604769787390616, 8.703668910516690005, 3.930664473729216901 ) ) ;
#39019=EDGE_CURVE ( 'NONE', #174805, #124865, #30480, .T. ) ;
#39026=EDGE_LOOP ( 'NONE', ( #144721, #36221, #199608, #162500 ) ) ;
#39047=CARTESIAN_POINT ( 'NONE',  ( -10.64985034906098882, 4.117567600086831980, 6.884957259278849051 ) ) ;
#39048=ORIENTED_EDGE ( 'NONE', *, *, #202497, .F. ) ;
#39088=CARTESIAN_POINT ( 'NONE',  ( 11.94650005372637835, 13.65102700337638275, 1.135399707157307203 ) ) ;
#39092=ADVANCED_FACE ( 'NONE', ( #72374 ), #57215, .F. ) ;
#39099=CARTESIAN_POINT ( 'NONE',  ( -9.604686356149274573, 3.481548657788671619, -7.193747284969077782 ) ) ;
#39102=CARTESIAN_POINT ( 'NONE',  ( -11.33772463945036968, 10.19999999999999929, -3.600000000000000977 ) ) ;
#39139=EDGE_CURVE ( 'NONE', #64100, #79124, #82401, .T. ) ;
#39164=CARTESIAN_POINT ( 'NONE',  ( 11.41108574530281494, 9.841631446223743751, -3.405883542057589253 ) ) ;
#39167=ORIENTED_EDGE ( 'NONE', *, *, #168889, .F. ) ;
#39168=AXIS2_PLACEMENT_3D ( 'NONE', #210544, #91493, #124062 ) ;
#39173=MECHANICAL_DESIGN_GEOMETRIC_PRESENTATION_REPRESENTATION('',(#194849),#49514);
#39182=CARTESIAN_POINT ( 'NONE',  ( -10.57232898948313604, 5.599354254162436817, 4.968808419985093039 ) ) ;
#39194=ORIENTED_EDGE ( 'NONE', *, *, #66840, .F. ) ;
#39206=CARTESIAN_POINT ( 'NONE',  ( -15.75000000000000000, 10.19999999999999929, -1.100000000000000311 ) ) ;
#39211=DIRECTION ( 'NONE',  ( 0.000000000000000000, -1.000000000000000000, 0.000000000000000000 ) ) ;
#39221=MECHANICAL_DESIGN_GEOMETRIC_PRESENTATION_REPRESENTATION('',(#143015),#122191);
#39243=DIRECTION ( 'NONE',  ( -0.9885327375000381167, 0.000000000000000000, -0.1510067114093955609 ) ) ;
#39248=CARTESIAN_POINT ( 'NONE',  ( 0.000000000000000000, 8.500000000000000000, 0.000000000000000000 ) ) ;
#39272=EDGE_CURVE ( 'NONE', #73634, #37563, #74535, .T. ) ;
#39287=CARTESIAN_POINT ( 'NONE',  ( 8.398252340528729931, 15.16388421002588593, 8.572949304411110916 ) ) ;
#39312=AXIS2_PLACEMENT_3D ( 'NONE', #20649, #3327, #201527 ) ;
#39340=EDGE_CURVE ( 'NONE', #169237, #136644, #16682, .T. ) ;
#39343=CARTESIAN_POINT ( 'NONE',  ( 9.348381460497192208, 13.52536904890506797, 7.450314784081282227 ) ) ;
#39348=CARTESIAN_POINT ( 'NONE',  ( -10.71030397718323890, 6.055815897892919075, -4.668189396100475008 ) ) ;
#39353=CARTESIAN_POINT ( 'NONE',  ( -4.930951480464074166E-10, 14.48154074412735426, -12.00000000000003553 ) ) ;
#39361=ADVANCED_FACE ( 'NONE', ( #109239 ), #87182, .T. ) ;
#39389=EDGE_CURVE ( 'NONE', #84082, #7772, #172355, .T. ) ;
#39438=CARTESIAN_POINT ( 'NONE',  ( -7.817327168174091234, 14.48014722064626802, -9.115250753896237512 ) ) ;
#39448=EDGE_LOOP ( 'NONE', ( #27454, #140514, #80589, #48999, #161355 ) ) ;
#39461=DIRECTION ( 'NONE',  ( -0.000000000000000000, 1.000000000000000000, 0.000000000000000000 ) ) ;
#39486=LINE ( 'NONE', #206247, #199362 ) ;
#39496=CARTESIAN_POINT ( 'NONE',  ( 0.000000000000000000, 13.87999999999998302, 0.000000000000000000 ) ) ;
#39516=TOROIDAL_SURFACE ( 'NONE', #160596, 11.92000000000000171, 0.08000000000000000167 ) ;
#39525=PLANE ( 'NONE',  #36873 ) ;
#39572=CARTESIAN_POINT ( 'NONE',  ( -11.83624332731381124, 4.942650230196960592, 4.855242260347336192 ) ) ;
#39581=CARTESIAN_POINT ( 'NONE',  ( 9.333041836227126353, 3.553052365627043407, 7.472413793103448221 ) ) ;
#39590=CARTESIAN_POINT ( 'NONE',  ( 0.000000000000000000, 9.799999999999982947, 0.000000000000000000 ) ) ;
#39641=VERTEX_POINT ( 'NONE', #130815 ) ;
#39677=ADVANCED_FACE ( 'NONE', ( #83041 ), #214076, .F. ) ;
#39690=CARTESIAN_POINT ( 'NONE',  ( -12.15542830485202153, 9.245334104615434256, -2.757920875862237775 ) ) ;
#39695=ORIENTED_EDGE ( 'NONE', *, *, #154536, .T. ) ;
#39697=CARTESIAN_POINT ( 'NONE',  ( 8.900812118921299643, 12.80989862106750543, 8.049590783350238254 ) ) ;
#39707=ORIENTED_EDGE ( 'NONE', *, *, #187404, .T. ) ;
#39713=( BOUNDED_SURFACE ( )  B_SPLINE_SURFACE ( 3, 3, ( 
 ( #66028, #133234, #185126, #199238, #186198, #36751, #184069, #49817, #20496, #181932, #117008, #102837, #86581, #70301, #120224, #37832 ),
 ( #103909, #169955, #21542, #35688, #3164, #166772, #69235, #83366, #33563, #118082, #2096, #183008, #136417, #34625, #101764, #18368 ),
 ( #17290, #152646, #149452, #1034, #84445, #19430, #68169, #174259, #175312, #109303, #204570, #121299, #22622, #38901, #57285, #56218 ),
 ( #41052, #9590, #107161, #5291, #7442, #73523, #75666, #171026, #139625, #55152, #43190, #189410, #205648, #123448, #108235, #173186 ),
 ( #206720, #155856, #24766, #91940, #90869, #207781, #23701, #156932, #8521, #25831, #89811, #74602, #140706, #93003, #58348, #39977 ),
 ( #6375, #187273, #124504, #137485, #104985, #190463, #158001, #188338, #141774, #59408, #71369, #42122, #125565, #191525, #106085, #26899 ),
 ( #203499, #72445, #88732, #154788, #138546, #122381, #172108, #46370, #29049, #212031, #77787, #129827, #142833, #79912, #162249, #48504 ) ),
 .UNSPECIFIED., .T., .F., .F. ) 
 B_SPLINE_SURFACE_WITH_KNOTS ( ( 4, 3, 4 ),
 ( 4, 2, 2, 2, 2, 2, 2, 4 ),
 ( 0.000000000000000000, 0.5000000000000000000, 1.000000000000000000 ),
 ( 0.3501333200791456046, 0.3551713324458994903, 0.3602093448126533759, 0.3702853695461611472, 0.3803518226137216351, 0.3853850491475018791, 0.3879016624143920011, 0.3904182756812821231 ),
 .UNSPECIFIED. ) 
 GEOMETRIC_REPRESENTATION_ITEM ( )  RATIONAL_B_SPLINE_SURFACE ( (
 ( 1.000000000000000000, 1.000000000000000000, 1.000000000000000000, 1.000000000000000000, 1.000000000000000000, 1.000000000000000000, 1.000000000000000000, 1.000000000000000000, 1.000000000000000000, 1.000000000000000000, 1.000000000000000000, 1.000000000000000000, 1.000000000000000000, 1.000000000000000000, 1.000000000000000000, 1.000000000000000000),
 ( 0.3333333333333333703, 0.3333333333333333703, 0.3333333333333333703, 0.3333333333333333703, 0.3333333333333333703, 0.3333333333333333703, 0.3333333333333333703, 0.3333333333333333703, 0.3333333333333333703, 0.3333333333333333703, 0.3333333333333333703, 0.3333333333333333703, 0.3333333333333333703, 0.3333333333333333703, 0.3333333333333333703, 0.3333333333333333703),
 ( 0.3333333333333333703, 0.3333333333333333703, 0.3333333333333333703, 0.3333333333333333703, 0.3333333333333333703, 0.3333333333333333703, 0.3333333333333333703, 0.3333333333333333703, 0.3333333333333333703, 0.3333333333333333703, 0.3333333333333333703, 0.3333333333333333703, 0.3333333333333333703, 0.3333333333333333703, 0.3333333333333333703, 0.3333333333333333703),
 ( 1.000000000000000000, 1.000000000000000000, 1.000000000000000000, 1.000000000000000000, 1.000000000000000000, 1.000000000000000000, 1.000000000000000000, 1.000000000000000000, 1.000000000000000000, 1.000000000000000000, 1.000000000000000000, 1.000000000000000000, 1.000000000000000000, 1.000000000000000000, 1.000000000000000000, 1.000000000000000000),
 ( 0.3333333333333333703, 0.3333333333333333703, 0.3333333333333333703, 0.3333333333333333703, 0.3333333333333333703, 0.3333333333333333703, 0.3333333333333333703, 0.3333333333333333703, 0.3333333333333333703, 0.3333333333333333703, 0.3333333333333333703, 0.3333333333333333703, 0.3333333333333333703, 0.3333333333333333703, 0.3333333333333333703, 0.3333333333333333703),
 ( 0.3333333333333333703, 0.3333333333333333703, 0.3333333333333333703, 0.3333333333333333703, 0.3333333333333333703, 0.3333333333333333703, 0.3333333333333333703, 0.3333333333333333703, 0.3333333333333333703, 0.3333333333333333703, 0.3333333333333333703, 0.3333333333333333703, 0.3333333333333333703, 0.3333333333333333703, 0.3333333333333333703, 0.3333333333333333703),
 ( 1.000000000000000000, 1.000000000000000000, 1.000000000000000000, 1.000000000000000000, 1.000000000000000000, 1.000000000000000000, 1.000000000000000000, 1.000000000000000000, 1.000000000000000000, 1.000000000000000000, 1.000000000000000000, 1.000000000000000000, 1.000000000000000000, 1.000000000000000000, 1.000000000000000000, 1.000000000000000000) ) ) 
 REPRESENTATION_ITEM ( '' )  SURFACE ( )  );
#39721=CARTESIAN_POINT ( 'NONE',  ( -3.531379752551939699, 15.51966450444894008, -11.47742190998778788 ) ) ;
#39736=CARTESIAN_POINT ( 'NONE',  ( 11.86145016429272836, 12.69999999999999929, -1.100000000000000311 ) ) ;
#39746=ORIENTED_EDGE ( 'NONE', *, *, #157187, .T. ) ;
#39766=SURFACE_STYLE_USAGE ( .BOTH. , #190264 ) ;
#39772=CARTESIAN_POINT ( 'NONE',  ( -10.10707714348148301, 4.359868340440408829, -5.857196085253971063 ) ) ;
#39824=DIRECTION ( 'NONE',  ( -0.8003905296791066215, 0.000000000000000000, -0.5994789404140892231 ) ) ;
#39828=ORIENTED_EDGE ( 'NONE', *, *, #19530, .T. ) ;
#39841=CARTESIAN_POINT ( 'NONE',  ( 11.81905481421901705, 13.75735655617266495, -1.592167362352180149 ) ) ;
#39843=AXIS2_PLACEMENT_3D ( 'NONE', #191579, #40026, #72501 ) ;
#39869=FACE_OUTER_BOUND ( 'NONE', #6126, .T. ) ;
#39876=CARTESIAN_POINT ( 'NONE',  ( 11.84668730067608600, 19.00000000000000000, -1.320000000000001616 ) ) ;
#39884=AXIS2_PLACEMENT_3D ( 'NONE', #81254, #148399, #193931 ) ;
#39893=CARTESIAN_POINT ( 'NONE',  ( 11.33772463945036790, 19.00000000000000000, -3.680000000000002824 ) ) ;
#39899=DIRECTION ( 'NONE',  ( 0.9885327375000381167, 0.000000000000000000, 0.1510067114093955609 ) ) ;
#39908=CIRCLE ( 'NONE', #160964, 0.08000000000000040412 ) ;
#39977=CARTESIAN_POINT ( 'NONE',  ( -11.76695491367977198, 4.673720869072629291, 4.995412848167409159 ) ) ;
#39989=( GEOMETRIC_REPRESENTATION_CONTEXT ( 3 ) GLOBAL_UNCERTAINTY_ASSIGNED_CONTEXT ( ( #191927 ) ) GLOBAL_UNIT_ASSIGNED_CONTEXT ( ( #38477, #118715, #101332 ) ) REPRESENTATION_CONTEXT ( 'NONE', 'WORKASPACE' ) );
#39993=AXIS2_PLACEMENT_3D ( 'NONE', #7468, #139650, #91965 ) ;
#40012=CARTESIAN_POINT ( 'NONE',  ( 10.51595811585101004, 9.986596539918549453, -3.553980774159643197 ) ) ;
#40026=DIRECTION ( 'NONE',  ( -1.000000000000000000, 0.000000000000000000, 0.000000000000000000 ) ) ;
#40039=DIRECTION ( 'NONE',  ( 0.000000000000000000, 0.000000000000000000, -1.000000000000000000 ) ) ;
#40071=CARTESIAN_POINT ( 'NONE',  ( -4.353456923439328108, 15.51896013954493192, 11.19146259264864085 ) ) ;
#40080=EDGE_LOOP ( 'NONE', ( #156000, #30119, #34739, #10982, #146094, #81451, #38759, #5324 ) ) ;
#40084=CARTESIAN_POINT ( 'NONE',  ( 11.88168329227126563, 11.38000000000000078, -1.685799833707129380 ) ) ;
#40085=CARTESIAN_POINT ( 'NONE',  ( 10.35108092051076412, 10.47472330378973204, 5.983479465268499276 ) ) ;
#40106=B_SPLINE_CURVE_WITH_KNOTS ( 'NONE', 3,
 ( #75248, #204133, #170598, #138124, #205217, #108883 ),
 .UNSPECIFIED., .F., .F.,
 ( 4, 2, 4 ),
 ( 0.000000000000000000, 0.0003779448103413553901, 0.0007558896206827107802 ),
 .UNSPECIFIED. ) ;
#40117=CARTESIAN_POINT ( 'NONE',  ( -10.82858503610327894, 5.585649091226504659, 6.509997993261127824 ) ) ;
#40121=UNCERTAINTY_MEASURE_WITH_UNIT (LENGTH_MEASURE( 1.000000000000000082E-05 ), #16299, 'distance_accuracy_value', 'NONE');
#40135=EDGE_LOOP ( 'NONE', ( #58314, #177613, #89278, #200665 ) ) ;
#40146=CIRCLE ( 'NONE', #136936, 0.08000000000000020983 ) ;
#40158=CARTESIAN_POINT ( 'NONE',  ( 11.89197816957260478, 13.79999999999999893, 0.8055420615339539125 ) ) ;
#40167=CARTESIAN_POINT ( 'NONE',  ( -8.795359111960578957, 14.48154074047005757, 8.214599990152152031 ) ) ;
#40174=CARTESIAN_POINT ( 'NONE',  ( 11.89942855770814312, 11.37999999999999901, -0.7000000000000009548 ) ) ;
#40193=ORIENTED_EDGE ( 'NONE', *, *, #29138, .T. ) ;
#40196=MECHANICAL_DESIGN_GEOMETRIC_PRESENTATION_REPRESENTATION('',(#19443),#140576);
#40213=VECTOR ( 'NONE', #48091, 1000.000000000000000 ) ;
#40255=CARTESIAN_POINT ( 'NONE',  ( -11.13243988973272636, 5.430794512910079419, -4.010128837087161280 ) ) ;
#40257=CARTESIAN_POINT ( 'NONE',  ( 9.165183341830644537, 14.44137815449902895, 8.758053443030863860 ) ) ;
#40272=AXIS2_PLACEMENT_3D ( 'NONE', #12485, #69749, #151045 ) ;
#40313=DIRECTION ( 'NONE',  ( 1.000000000000000000, -0.000000000000000000, -0.000000000000000000 ) ) ;
#40327=SURFACE_STYLE_USAGE ( .BOTH. , #87997 ) ;
#40358=FILL_AREA_STYLE ('',( #26212 ) ) ;
#40385=CYLINDRICAL_SURFACE ( 'NONE', #8902, 12.00000000000000178 ) ;
#40395=ORIENTED_EDGE ( 'NONE', *, *, #151879, .T. ) ;
#40424=PRESENTATION_STYLE_ASSIGNMENT (( #188789 ) ) ;
#40433=CARTESIAN_POINT ( 'NONE',  ( -11.69243366784185945, 8.407932920124673970, 1.097391832464843286 ) ) ;
#40439=CARTESIAN_POINT ( 'NONE',  ( -3.530628709500676976, 14.55202870934159520, -11.43095269779774448 ) ) ;
#40461=AXIS2_PLACEMENT_3D ( 'NONE', #76577, #109161, #39824 ) ;
#40483=FACE_OUTER_BOUND ( 'NONE', #189299, .T. ) ;
#40498=VERTEX_POINT ( 'NONE', #176843 ) ;
#40510=CARTESIAN_POINT ( 'NONE',  ( -15.75000000000000000, 12.69999999999998153, 1.799999999999999600 ) ) ;
#40516=( GEOMETRIC_REPRESENTATION_CONTEXT ( 3 ) GLOBAL_UNCERTAINTY_ASSIGNED_CONTEXT ( ( #40121 ) ) GLOBAL_UNIT_ASSIGNED_CONTEXT ( ( #16299, #34697, #108313 ) ) REPRESENTATION_CONTEXT ( 'NONE', 'WORKASPACE' ) );
#40524=ORIENTED_EDGE ( 'NONE', *, *, #157408, .T. ) ;
#40537=CARTESIAN_POINT ( 'NONE',  ( 9.453622214572620308, 4.518459228531092720, -7.392429638475873865 ) ) ;
#40547=CARTESIAN_POINT ( 'NONE',  ( -10.65047922011206261, 5.918049078515057460, 5.531760622192766874 ) ) ;
#40550=CARTESIAN_POINT ( 'NONE',  ( 11.84668730067608244, 12.69999999999998153, 1.319999999999998286 ) ) ;
#40567=ADVANCED_FACE ( 'NONE', ( #180046 ), #24430, .F. ) ;
#40577=DIRECTION ( 'NONE',  ( -0.000000000000000000, -1.000000000000000000, -0.000000000000000000 ) ) ;
#40584=ADVANCED_FACE ( 'NONE', ( #144390 ), #146504, .F. ) ;
#40588=DIRECTION ( 'NONE',  ( -0.9632918427306580433, 0.000000000000000000, 0.2684563758389303945 ) ) ;
#40600=CARTESIAN_POINT ( 'NONE',  ( -11.55950211276791428, 9.719999999999998863, -3.221476510067114329 ) ) ;
#40608=CARTESIAN_POINT ( 'NONE',  ( -11.33772463945037146, 11.00911576511424528, 3.599999999999998757 ) ) ;
#40612=ADVANCED_FACE ( 'NONE', ( #35908 ), #184282, .T. ) ;
#40663=CARTESIAN_POINT ( 'NONE',  ( -11.91002632418505058, 5.203875245307159503, 4.700031268430899800 ) ) ;
#40671=COLOUR_RGB ( '', 0.09019608, 0.27058824, 0.51372549) ;
#40689=CARTESIAN_POINT ( 'NONE',  ( 9.604651411913359027, 12.70286830212710072, 7.196651313930959581 ) ) ;
#40723=( NAMED_UNIT ( * ) PLANE_ANGLE_UNIT ( ) SI_UNIT ( $, .RADIAN. ) );
#40779=CARTESIAN_POINT ( 'NONE',  ( -10.37105062950515943, 6.927298630606520291, 5.133691221222295376 ) ) ;
#40785=CARTESIAN_POINT ( 'NONE',  ( 0.000000000000000000, 9.799999999999998934, 0.000000000000000000 ) ) ;
#40798=CARTESIAN_POINT ( 'NONE',  ( -15.75000000000000000, 12.30000000000000071, -1.800000000000001155 ) ) ;
#40802=( GEOMETRIC_REPRESENTATION_CONTEXT ( 3 ) GLOBAL_UNCERTAINTY_ASSIGNED_CONTEXT ( ( #81398 ) ) GLOBAL_UNIT_ASSIGNED_CONTEXT ( ( #207681, #57177, #88623 ) ) REPRESENTATION_CONTEXT ( 'NONE', 'WORKASPACE' ) );
#40844=ORIENTED_EDGE ( 'NONE', *, *, #72931, .F. ) ;
#40849=DIRECTION ( 'NONE',  ( 1.000000000000000000, -0.000000000000000000, -0.000000000000000000 ) ) ;
#40855=CARTESIAN_POINT ( 'NONE',  ( -11.27976636440881641, 5.060096319113082330, -5.788224378391188196 ) ) ;
#40918=CARTESIAN_POINT ( 'NONE',  ( 11.75119899582183614, 6.933193708961042034, -2.442676079799758426 ) ) ;
#40924=CIRCLE ( 'NONE', #193034, 11.92000000000000171 ) ;
#40928=PLANE ( 'NONE',  #37362 ) ;
#40945=CARTESIAN_POINT ( 'NONE',  ( -11.01135777277262129, 12.69999999999999929, -1.400000000000001910 ) ) ;
#40947=ORIENTED_EDGE ( 'NONE', *, *, #22937, .F. ) ;
#40951=LINE ( 'NONE', #4132, #12778 ) ;
#40971=CARTESIAN_POINT ( 'NONE',  ( 1.734723475976807094E-15, 15.00041888085534758, 11.91973154060107376 ) ) ;
#40989=SURFACE_SIDE_STYLE ('',( #189349 ) ) ;
#41051=CARTESIAN_POINT ( 'NONE',  ( -11.94980361058169116, 13.39999999999999858, 1.099999999999994982 ) ) ;
#41052=CARTESIAN_POINT ( 'NONE',  ( -10.14895191633106819, 4.000000000000000888, 7.601392964450660372 ) ) ;
#41083=CARTESIAN_POINT ( 'NONE',  ( -1.796836089791512103, 14.48004991555888310, 11.89866442307391736 ) ) ;
#41094=CARTESIAN_POINT ( 'NONE',  ( 11.96217875511318063, 11.32854366578976446, -0.9561995067075083066 ) ) ;
#41119=DIRECTION ( 'NONE',  ( 0.000000000000000000, 0.000000000000000000, -1.000000000000000000 ) ) ;
#41122=CARTESIAN_POINT ( 'NONE',  ( -9.604686356149274573, 3.481540744127370690, 7.193747284969077782 ) ) ;
#41135=FILL_AREA_STYLE ('',( #75743 ) ) ;
#41152=CARTESIAN_POINT ( 'NONE',  ( -1.741635578173613697, 15.44819650159847235, 11.86206419467665185 ) ) ;
#41165=CARTESIAN_POINT ( 'NONE',  ( -11.01135777277262306, 10.09367418006288197, 1.399999999999998579 ) ) ;
#41166=AXIS2_PLACEMENT_3D ( 'NONE', #59649, #28221, #124743 ) ;
#41167=CARTESIAN_POINT ( 'NONE',  ( 11.09299181971603510, 9.057582982347017975, -4.454713115659062694 ) ) ;
#41168=CARTESIAN_POINT ( 'NONE',  ( -1.499999999999964029, 7.750000000000000000, 10.64483442802189117 ) ) ;
#41189=SURFACE_SIDE_STYLE ('',( #6507 ) ) ;
#41198=CARTESIAN_POINT ( 'NONE',  ( -0.02465203476893947088, 15.46327782766690007, 11.97749487451462613 ) ) ;
#41199=CARTESIAN_POINT ( 'NONE',  ( -10.81012925547440773, 5.523932969818027949, 6.547168141744070802 ) ) ;
#41214=DIRECTION ( 'NONE',  ( 1.000000000000000000, -0.000000000000000000, -0.000000000000000000 ) ) ;
#41249=CARTESIAN_POINT ( 'NONE',  ( -6.714560252712822752, 14.48050415317768724, 9.956001885444296207 ) ) ;
#41252=DIRECTION ( 'NONE',  ( -0.6249999999999992228, 1.210928637341016588E-14, -0.7806247497998003437 ) ) ;
#41260=FILL_AREA_STYLE_COLOUR ( '', #30656 ) ;
#41262=VECTOR ( 'NONE', #26290, 1000.000000000000000 ) ;
#41298=CARTESIAN_POINT ( 'NONE',  ( -11.41381675112453387, 10.90000000000000036, -3.704697986577184299 ) ) ;
#41332=ORIENTED_EDGE ( 'NONE', *, *, #204060, .T. ) ;
#41338=CARTESIAN_POINT ( 'NONE',  ( -10.78227258717170578, 6.269840026405313793, 4.500979083849748541 ) ) ;
#41353=CARTESIAN_POINT ( 'NONE',  ( 11.94980361058169116, 12.70000000000000107, 1.099999999999994982 ) ) ;
#41357=ORIENTED_EDGE ( 'NONE', *, *, #23547, .T. ) ;
#41368=DIRECTION ( 'NONE',  ( 1.000000000000000000, -0.000000000000000000, -0.000000000000000000 ) ) ;
#41384=CARTESIAN_POINT ( 'NONE',  ( 11.89829993707161471, 13.82919228251124721, 1.561606677374347329 ) ) ;
#41395=ORIENTED_EDGE ( 'NONE', *, *, #175333, .T. ) ;
#41397=EDGE_LOOP ( 'NONE', ( #174661, #107209, #39167, #102565 ) ) ;
#41408=SURFACE_STYLE_FILL_AREA ( #123797 ) ;
#41411=AXIS2_PLACEMENT_3D ( 'NONE', #180562, #197866, #210917 ) ;
#41425=ORIENTED_EDGE ( 'NONE', *, *, #130663, .F. ) ;
#41433=( GEOMETRIC_REPRESENTATION_CONTEXT ( 3 ) GLOBAL_UNCERTAINTY_ASSIGNED_CONTEXT ( ( #196722 ) ) GLOBAL_UNIT_ASSIGNED_CONTEXT ( ( #25166, #7839, #175704 ) ) REPRESENTATION_CONTEXT ( 'NONE', 'WORKASPACE' ) );
#41497=( LENGTH_UNIT ( ) NAMED_UNIT ( * ) SI_UNIT ( .MILLI., .METRE. ) );
#41504=CARTESIAN_POINT ( 'NONE',  ( -11.01135777277262129, 10.89999999999998259, 1.399999999999998579 ) ) ;
#41508=CARTESIAN_POINT ( 'NONE',  ( -9.367496997901326949, 14.48154074413197456, -7.499999999620649227 ) ) ;
#41548=EDGE_CURVE ( 'NONE', #136086, #103541, #151640, .T. ) ;
#41558=CARTESIAN_POINT ( 'NONE',  ( -11.94650005372637835, 12.44897299662361867, 1.135399707157293658 ) ) ;
#41567=CARTESIAN_POINT ( 'NONE',  ( -11.41381678389388377, 11.02879418241073139, -3.704697885617973530 ) ) ;
#41572=ORIENTED_EDGE ( 'NONE', *, *, #45759, .F. ) ;
#41598=CARTESIAN_POINT ( 'NONE',  ( 10.48252959204799772, 8.670818378862373166, 6.558037413528325033 ) ) ;
#41602=CARTESIAN_POINT ( 'NONE',  ( -3.543819121313565468, 14.48034520796839253, -11.47346693582755606 ) ) ;
#41614=CARTESIAN_POINT ( 'NONE',  ( 9.574107575049746188, 3.767509416808712430, -7.159700411437375678 ) ) ;
#41616=DIRECTION ( 'NONE',  ( 1.224646799147343346E-16, 0.000000000000000000, -1.000000000000000000 ) ) ;
#41624=( NAMED_UNIT ( * ) SI_UNIT ( $, .STERADIAN. ) SOLID_ANGLE_UNIT ( ) );
#41651=CARTESIAN_POINT ( 'NONE',  ( 11.33772463945037146, 19.00000000000000000, 3.679999999999999272 ) ) ;
#41697=CARTESIAN_POINT ( 'NONE',  ( 0.000000000000000000, 3.999999999999994671, 12.00000000000000355 ) ) ;
#41704=CARTESIAN_POINT ( 'NONE',  ( 8.985344024325859991, 14.65809313286843185, 7.243008760641457044 ) ) ;
#41724=CARTESIAN_POINT ( 'NONE',  ( 11.86687215968023601, 9.990577876942188240, 1.056395335932121871 ) ) ;
#41728=SURFACE_STYLE_FILL_AREA ( #192199 ) ;
#41737=CARTESIAN_POINT ( 'NONE',  ( -11.33520460194134394, 5.279085700950885141, -5.677819296561938955 ) ) ;
#41751=DIRECTION ( 'NONE',  ( -0.000000000000000000, -1.000000000000000000, -0.000000000000000000 ) ) ;
#41764=CARTESIAN_POINT ( 'NONE',  ( 10.19611990457454453, 10.80814481035635310, 6.242388940945101439 ) ) ;
#41771=AXIS2_PLACEMENT_3D ( 'NONE', #128003, #75952, #176656 ) ;
#41786=AXIS2_PLACEMENT_3D ( 'NONE', #33905, #182280, #131468 ) ;
#41831=ORIENTED_EDGE ( 'NONE', *, *, #56390, .F. ) ;
#41839=EDGE_LOOP ( 'NONE', ( #30531, #53319, #26065, #3703 ) ) ;
#41855=CARTESIAN_POINT ( 'NONE',  ( -10.16827420574893814, 6.288608293322982767, 5.589418380748610637 ) ) ;
#41888=AXIS2_PLACEMENT_3D ( 'NONE', #200400, #182023, #67194 ) ;
#41894=SURFACE_SIDE_STYLE ('',( #158823 ) ) ;
#41918=VERTEX_POINT ( 'NONE', #150958 ) ;
#41927=CARTESIAN_POINT ( 'NONE',  ( -11.76696981052429614, 4.673730779118267620, -4.995440715239801044 ) ) ;
#41943=ORIENTED_EDGE ( 'NONE', *, *, #37763, .F. ) ;
#41995=CARTESIAN_POINT ( 'NONE',  ( 11.84692183557065626, 6.792745295355079094, 1.971868844856123681 ) ) ;
#42029=LINE ( 'NONE', #108141, #159463 ) ;
#42056=EDGE_CURVE ( 'NONE', #13289, #37994, #140905, .T. ) ;
#42085=ORIENTED_EDGE ( 'NONE', *, *, #67181, .F. ) ;
#42090=ORIENTED_EDGE ( 'NONE', *, *, #68660, .T. ) ;
#42116=CARTESIAN_POINT ( 'NONE',  ( 0.000000000000000000, 9.719999999999998863, 0.000000000000000000 ) ) ;
#42118=ORIENTED_EDGE ( 'NONE', *, *, #206271, .T. ) ;
#42122=CARTESIAN_POINT ( 'NONE',  ( -10.80846816847880909, 4.295462489797631456, 4.678010962757586100 ) ) ;
#42128=CARTESIAN_POINT ( 'NONE',  ( -11.89317557362582534, 11.26275843837606061, -1.599935658896117774 ) ) ;
#42144=LINE ( 'NONE', #159070, #32879 ) ;
#42184=CARTESIAN_POINT ( 'NONE',  ( 9.348761378620915607, 13.52553930298125096, -7.449808453853658641 ) ) ;
#42186=( GEOMETRIC_REPRESENTATION_CONTEXT ( 3 ) GLOBAL_UNCERTAINTY_ASSIGNED_CONTEXT ( ( #120879 ) ) GLOBAL_UNIT_ASSIGNED_CONTEXT ( ( #10082, #148366, #173690 ) ) REPRESENTATION_CONTEXT ( 'NONE', 'WORKASPACE' ) );
#42189=CARTESIAN_POINT ( 'NONE',  ( -9.912081330994999107, 3.481540842592264706, 6.783330821352332229 ) ) ;
#42214=COLOUR_RGB ( '', 0.40784314, 0.44705882, 0.49803922) ;
#42217=CARTESIAN_POINT ( 'NONE',  ( -5.973546839618155246, 15.51882391377835368, 10.41731636723813814 ) ) ;
#42219=DIRECTION ( 'NONE',  ( 0.000000000000000000, -1.000000000000000000, 0.000000000000000000 ) ) ;
#42256=FACE_OUTER_BOUND ( 'NONE', #73332, .T. ) ;
#42279=( BOUNDED_CURVE ( )  B_SPLINE_CURVE ( 3, ( #113110, #193219, #176977, #31802 ),
 .UNSPECIFIED., .F., .T. ) 
 B_SPLINE_CURVE_WITH_KNOTS ( ( 4, 4 ),
 ( 1.683648326080136037, 1.706346174174820041 ),
 .UNSPECIFIED. ) 
 CURVE ( )  GEOMETRIC_REPRESENTATION_ITEM ( )  RATIONAL_B_SPLINE_CURVE ( ( 1.000000000000000000, 0.9999570677684579412, 0.9999570677684579412, 1.000000000000000000 ) ) 
 REPRESENTATION_ITEM ( '' )  );
#42355=ORIENTED_EDGE ( 'NONE', *, *, #4802, .T. ) ;
#42364=CARTESIAN_POINT ( 'NONE',  ( 1.448815997565456204, 7.903552007303736637, 10.65195286442483358 ) ) ;
#42376=( NAMED_UNIT ( * ) SI_UNIT ( $, .STERADIAN. ) SOLID_ANGLE_UNIT ( ) );
#42386=DIRECTION ( 'NONE',  ( -0.8164965809277262565, 8.702247276351162783E-15, 0.5773502691896256200 ) ) ;
#42387=CARTESIAN_POINT ( 'NONE',  ( 10.51596412982177853, 13.61340918268422939, -3.553961965504329523 ) ) ;
#42388=CARTESIAN_POINT ( 'NONE',  ( 11.49966000274960898, 9.857671544352703208, -3.429881629453144232 ) ) ;
#42406=CARTESIAN_POINT ( 'NONE',  ( -10.47022434975266592, 4.009060182194922994, -5.775464948712724755 ) ) ;
#42459=CARTESIAN_POINT ( 'NONE',  ( -11.55950211276791428, 13.87999999999998302, 3.221476510067114329 ) ) ;
#42464=ORIENTED_EDGE ( 'NONE', *, *, #5717, .F. ) ;
#42477=AXIS2_PLACEMENT_3D ( 'NONE', #63418, #159850, #164124 ) ;
#42502=CIRCLE ( 'NONE', #97844, 12.00000000000000178 ) ;
#42507=EDGE_LOOP ( 'NONE', ( #71226, #205815, #193872, #50731 ) ) ;
#42516=CARTESIAN_POINT ( 'NONE',  ( 9.289939459345561090, 13.86364823901540788, 7.523963912448549785 ) ) ;
#42529=ORIENTED_EDGE ( 'NONE', *, *, #208952, .F. ) ;
#42536=CARTESIAN_POINT ( 'NONE',  ( 11.88168329227127096, 9.719999999999982876, 1.685799833707125606 ) ) ;
#42541=CARTESIAN_POINT ( 'NONE',  ( 11.55950211276791251, 9.719999999999982876, 3.221476510067110777 ) ) ;
#42548=ORIENTED_EDGE ( 'NONE', *, *, #121060, .F. ) ;
#42560=ORIENTED_EDGE ( 'NONE', *, *, #13809, .T. ) ;
#42584=CARTESIAN_POINT ( 'NONE',  ( -1.797327170199077839, 14.52975892672686342, -11.89862072626474898 ) ) ;
#42591=EDGE_LOOP ( 'NONE', ( #100847, #12155, #44292, #140439 ) ) ;
#42628=CARTESIAN_POINT ( 'NONE',  ( -11.97297122925973767, 12.30125079326911042, 0.8121202983519304475 ) ) ;
#42648=CARTESIAN_POINT ( 'NONE',  ( 10.26863146610705613, 10.84983613121963941, 6.215114292131002749 ) ) ;
#42655=CARTESIAN_POINT ( 'NONE',  ( -11.41381675112459959, 13.39999999999999325, 3.704697986577257129 ) ) ;
#42656=DIRECTION ( 'NONE',  ( -0.000000000000000000, 1.000000000000000000, 0.000000000000000000 ) ) ;
#42667=CIRCLE ( 'NONE', #104967, 0.07999999999999998779 ) ;
#42668=CARTESIAN_POINT ( 'NONE',  ( 11.23288463952165550, 7.775932670961701376, -5.438141635970919374 ) ) ;
#42672=CARTESIAN_POINT ( 'NONE',  ( -9.367496997901325173, 14.48154074412966175, -7.499999999620646562 ) ) ;
#42685=CARTESIAN_POINT ( 'NONE',  ( -15.75000000000000000, 13.79999999999999893, 0.6999999999999992895 ) ) ;
#42686=CARTESIAN_POINT ( 'NONE',  ( 9.574755896318496440, 4.231292707087964011, -7.158835548396402793 ) ) ;
#42709=DIRECTION ( 'NONE',  ( 0.000000000000000000, 0.000000000000000000, -1.000000000000000000 ) ) ;
#42713=LINE ( 'NONE', #155362, #94453 ) ;
#42726=CARTESIAN_POINT ( 'NONE',  ( 0.6674790882334172837, 16.00000000000000711, 11.66566053519463786 ) ) ;
#42740=CARTESIAN_POINT ( 'NONE',  ( 11.07790593930098311, 9.799999999999998934, -0.7000000000000009548 ) ) ;
#42769=( NAMED_UNIT ( * ) SI_UNIT ( $, .STERADIAN. ) SOLID_ANGLE_UNIT ( ) );
#42774=CARTESIAN_POINT ( 'NONE',  ( -11.48806469435255373, 12.26910227127551245, -3.468902948106704631 ) ) ;
#42776=CARTESIAN_POINT ( 'NONE',  ( 9.798003133828602884, 14.76688263464874851, 7.816136467581006997 ) ) ;
#42793=CARTESIAN_POINT ( 'NONE',  ( 0.000000000000000000, 9.799999999999998934, 0.000000000000000000 ) ) ;
#42805=ADVANCED_FACE ( 'NONE', ( #97701 ), #114009, .T. ) ;
#42808=CARTESIAN_POINT ( 'NONE',  ( -11.24554337403377069, 7.016168494911984688, 5.610835997672845465 ) ) ;
#42811=CARTESIAN_POINT ( 'NONE',  ( -10.98535488200955079, 12.34177443252770168, -1.593017372382190766 ) ) ;
#42835=CARTESIAN_POINT ( 'NONE',  ( 9.576657467935302037, 12.68194475294117574, 7.234045051690152661 ) ) ;
#42844=SURFACE_SIDE_STYLE ('',( #103553 ) ) ;
#42846=CARTESIAN_POINT ( 'NONE',  ( -11.88237951145550575, 13.75680652621284317, 0.9087114598430686696 ) ) ;
#42887=CARTESIAN_POINT ( 'NONE',  ( 0.08053691275167890185, 14.48195938056239385, 11.99972973886013961 ) ) ;
#42911=SURFACE_SIDE_STYLE ('',( #191247 ) ) ;
#42912=DIRECTION ( 'NONE',  ( 0.000000000000000000, 0.000000000000000000, -1.000000000000000000 ) ) ;
#42920=CARTESIAN_POINT ( 'NONE',  ( -11.24554337403377069, 7.016168494911984688, 5.610835997672845465 ) ) ;
#42925=CARTESIAN_POINT ( 'NONE',  ( 8.628381312412237492, 13.71601666663510066, 8.341747646421527662 ) ) ;
#42928=ORIENTED_EDGE ( 'NONE', *, *, #202990, .T. ) ;
#42936=ORIENTED_EDGE ( 'NONE', *, *, #72745, .T. ) ;
#42963=( GEOMETRIC_REPRESENTATION_CONTEXT ( 3 ) GLOBAL_UNCERTAINTY_ASSIGNED_CONTEXT ( ( #165334 ) ) GLOBAL_UNIT_ASSIGNED_CONTEXT ( ( #158740, #142518, #192278 ) ) REPRESENTATION_CONTEXT ( 'NONE', 'WORKASPACE' ) );
#42964=CARTESIAN_POINT ( 'NONE',  ( -15.75000000000000000, 12.69999999999998153, 3.199999999999997957 ) ) ;
#42994=CARTESIAN_POINT ( 'NONE',  ( -10.81015953665327345, 5.524082113754967160, -6.547048903644186346 ) ) ;
#43000=ORIENTED_EDGE ( 'NONE', *, *, #37661, .T. ) ;
#43003=CARTESIAN_POINT ( 'NONE',  ( 11.35610322553117513, 11.11421628929173089, 3.553412924323500643 ) ) ;
#43007=EDGE_CURVE ( 'NONE', #72859, #180190, #125608, .T. ) ;
#43010=CARTESIAN_POINT ( 'NONE',  ( -11.04536101718726293, 10.19999999999999929, 1.099999999999996758 ) ) ;
#43070=SURFACE_STYLE_FILL_AREA ( #143789 ) ;
#43075=DIRECTION ( 'NONE',  ( 0.000000000000000000, 0.4225362441286110715, -0.9063460279593478219 ) ) ;
#43076=ORIENTED_EDGE ( 'NONE', *, *, #212743, .T. ) ;
#43095=CARTESIAN_POINT ( 'NONE',  ( 11.04536101718726293, 13.50590937888830823, -1.100000000000000311 ) ) ;
#43097=CARTESIAN_POINT ( 'NONE',  ( 8.916861300403269297, 12.70687961389403675, 7.961634759295345809 ) ) ;
#43121=AXIS2_PLACEMENT_3D ( 'NONE', #97750, #51108, #163809 ) ;
#43125=CARTESIAN_POINT ( 'NONE',  ( 0.000000000000000000, 0.000000000000000000, 0.000000000000000000 ) ) ;
#43138=CARTESIAN_POINT ( 'NONE',  ( 8.279117182235522066, 15.22768336333823314, -8.688194556162066817 ) ) ;
#43174=CARTESIAN_POINT ( 'NONE',  ( -11.41157692552970460, 9.840896629129986195, 3.404533818002359435 ) ) ;
#43184=CARTESIAN_POINT ( 'NONE',  ( 11.84668730067608600, 13.39999999999998259, 1.399999999999998357 ) ) ;
#43189=CARTESIAN_POINT ( 'NONE',  ( 10.17148340815012020, 11.75186938811109627, -7.510838954888964025 ) ) ;
#43190=CARTESIAN_POINT ( 'NONE',  ( -11.19490907666120272, 4.805655862119510680, 5.952061394947645745 ) ) ;
#43252=SURFACE_STYLE_FILL_AREA ( #59472 ) ;
#43255=CARTESIAN_POINT ( 'NONE',  ( -10.60962610691052710, 4.146691825315026669, 5.607770086979924962 ) ) ;
#43267=ADVANCED_FACE ( 'NONE', ( #83548 ), #182699, .T. ) ;
#43303=CARTESIAN_POINT ( 'NONE',  ( 11.92619526913699524, 12.57219975838508041, 1.328859060402684644 ) ) ;
#43323=PRESENTATION_STYLE_ASSIGNMENT (( #175448 ) ) ;
#43333=ORIENTED_EDGE ( 'NONE', *, *, #171810, .F. ) ;
#43357=ORIENTED_EDGE ( 'NONE', *, *, #41548, .T. ) ;
#43378=CARTESIAN_POINT ( 'NONE',  ( 11.86145016429273191, 10.19999999999999929, -1.180000000000000604 ) ) ;
#43383=CARTESIAN_POINT ( 'NONE',  ( -11.89321938400720491, 11.26255278360659595, 1.599605898944226334 ) ) ;
#43389=CARTESIAN_POINT ( 'NONE',  ( 11.41381675112453387, 10.90000000000000036, -3.704697986577182522 ) ) ;
#43410=MECHANICAL_DESIGN_GEOMETRIC_PRESENTATION_REPRESENTATION('',(#126503),#39989);
#43411=CARTESIAN_POINT ( 'NONE',  ( -9.604686356149278126, 4.518467169708413778, -7.193747284969076006 ) ) ;
#43412=CARTESIAN_POINT ( 'NONE',  ( 10.51568781791557328, 13.61256730203911758, 3.554797817682051164 ) ) ;
#43414=FACE_OUTER_BOUND ( 'NONE', #773, .T. ) ;
#43425=CARTESIAN_POINT ( 'NONE',  ( 1.423205080756922314, 7.980384757729337863, 10.65537363484301459 ) ) ;
#43429=DIRECTION ( 'NONE',  ( 0.000000000000000000, 0.000000000000000000, -1.000000000000000000 ) ) ;
#43431=CARTESIAN_POINT ( 'NONE',  ( 0.000000000000000000, 12.29999999999998295, 0.000000000000000000 ) ) ;
#43442=ORIENTED_EDGE ( 'NONE', *, *, #26426, .F. ) ;
#43445=EDGE_CURVE ( 'NONE', #118697, #61441, #171944, .T. ) ;
#43446=SURFACE_STYLE_USAGE ( .BOTH. , #95404 ) ;
#43448=CARTESIAN_POINT ( 'NONE',  ( -11.78331023100045627, 9.799999999999998934, -1.800000000000001155 ) ) ;
#43455=ORIENTED_EDGE ( 'NONE', *, *, #158613, .F. ) ;
#43472=CARTESIAN_POINT ( 'NONE',  ( 7.320800350271525758, 15.00158243878686726, 10.35317514277968343 ) ) ;
#43495=DIRECTION ( 'NONE',  ( 0.000000000000000000, 1.804652791718263484E-16, -1.000000000000000000 ) ) ;
#43501=CARTESIAN_POINT ( 'NONE',  ( -10.62873463776380056, 12.30000000000000071, -3.200000000000001510 ) ) ;
#43519=ORIENTED_EDGE ( 'NONE', *, *, #127165, .T. ) ;
#43524=CARTESIAN_POINT ( 'NONE',  ( -11.41381675112453387, 13.39999999999998259, 3.704697986577180746 ) ) ;
#43578=CARTESIAN_POINT ( 'NONE',  ( 8.266504136565099969, 15.18065358759336547, 8.700162761727884941 ) ) ;
#43590=VERTEX_POINT ( 'NONE', #114540 ) ;
#43601=ORIENTED_EDGE ( 'NONE', *, *, #72745, .F. ) ;
#43622=ORIENTED_EDGE ( 'NONE', *, *, #3938, .F. ) ;
#43644=CARTESIAN_POINT ( 'NONE',  ( -10.48266952940149466, 5.268049057482275366, -5.154014898524191146 ) ) ;
#43659=LINE ( 'NONE', #194143, #56174 ) ;
#43709=FILL_AREA_STYLE_COLOUR ( '', #129172 ) ;
#43712=CARTESIAN_POINT ( 'NONE',  ( 11.81254310278123754, 7.953092247000543402, -2.153480349962514140 ) ) ;
#43714=ADVANCED_FACE ( 'NONE', ( #95045 ), #161095, .F. ) ;
#43716=CIRCLE ( 'NONE', #164751, 0.5000000000000016653 ) ;
#43720=CARTESIAN_POINT ( 'NONE',  ( -11.49978884755372732, 13.74270821162817668, 3.429452816445256236 ) ) ;
#43732=CARTESIAN_POINT ( 'NONE',  ( 8.384452190322788212, 12.99440559435832476, -8.518166066213405330 ) ) ;
#43735=ORIENTED_EDGE ( 'NONE', *, *, #36106, .T. ) ;
#43749=CARTESIAN_POINT ( 'NONE',  ( 9.518502046417362195, 4.418053365869059057, -7.307953274077121364 ) ) ;
#43756=CIRCLE ( 'NONE', #78355, 11.95586206896534698 ) ;
#43791=DIRECTION ( 'NONE',  ( -0.000000000000000000, -1.000000000000000000, -0.000000000000000000 ) ) ;
#43830=SURFACE_STYLE_FILL_AREA ( #112084 ) ;
#43837=CARTESIAN_POINT ( 'NONE',  ( 7.320235437844907267, 14.95386332671184881, 9.102015036127445669 ) ) ;
#43871=CARTESIAN_POINT ( 'NONE',  ( -12.04274103669372309, 7.374159847806027734, 3.963224530603232765 ) ) ;
#43890=ORIENTED_EDGE ( 'NONE', *, *, #209881, .T. ) ;
#43895=ORIENTED_EDGE ( 'NONE', *, *, #98658, .F. ) ;
#43896=CARTESIAN_POINT ( 'NONE',  ( 11.75926639340631041, 7.883781762499332046, -2.170924231206847743 ) ) ;
#43914=AXIS2_PLACEMENT_3D ( 'NONE', #179708, #64871, #65909 ) ;
#43941=CARTESIAN_POINT ( 'NONE',  ( -11.84668730067608600, 13.39999999999998259, 1.399999999999998579 ) ) ;
#43954=FILL_AREA_STYLE_COLOUR ( '', #157784 ) ;
#43980=CARTESIAN_POINT ( 'NONE',  ( -10.12897898315521061, 6.154003805053667620, 5.673299828594959848 ) ) ;
#43984=AXIS2_PLACEMENT_3D ( 'NONE', #70950, #154371, #22194 ) ;
#43986=SURFACE_STYLE_FILL_AREA ( #192327 ) ;
#44007=ORIENTED_EDGE ( 'NONE', *, *, #156764, .F. ) ;
#44015=COLOUR_RGB ( '', 0.09019608, 0.27058824, 0.51372549) ;
#44020=FACE_OUTER_BOUND ( 'NONE', #7979, .T. ) ;
#44044=DIRECTION ( 'NONE',  ( 1.000000000000000000, -0.000000000000000000, -0.000000000000000000 ) ) ;
#44047=CARTESIAN_POINT ( 'NONE',  ( -11.48788097203293823, 13.83043054397690241, -3.469500700354831491 ) ) ;
#44069=ORIENTED_EDGE ( 'NONE', *, *, #135546, .T. ) ;
#44073=CARTESIAN_POINT ( 'NONE',  ( -11.81911962874431055, 13.75710573484113830, 1.591749704452489533 ) ) ;
#44116=CARTESIAN_POINT ( 'NONE',  ( 11.48788097203293823, 9.769569456023095455, -3.469500700354831491 ) ) ;
#44118=CARTESIAN_POINT ( 'NONE',  ( 9.278192185738603825, 11.44758586271118084, 7.613438169660605936 ) ) ;
#44168=CARTESIAN_POINT ( 'NONE',  ( 9.017865005868369366, 14.59732426908277070, -7.917871330580335432 ) ) ;
#44170=PLANE ( 'NONE',  #130096 ) ;
#44179=CARTESIAN_POINT ( 'NONE',  ( 11.41126283316774348, 9.841253930915392800, 3.405403429622879230 ) ) ;
#44190=CARTESIAN_POINT ( 'NONE',  ( 7.861308842906358230, 15.31505636599913878, -9.009337879868121846 ) ) ;
#44223=ADVANCED_FACE ( 'NONE', ( #67549 ), #204834, .T. ) ;
#44243=CARTESIAN_POINT ( 'NONE',  ( 11.15162045555251957, 9.712998552558403276, 5.837063001226317382 ) ) ;
#44249=CARTESIAN_POINT ( 'NONE',  ( -11.84668729410359411, 11.00620512324533529, -1.400000000000001688 ) ) ;
#44251=( NAMED_UNIT ( * ) PLANE_ANGLE_UNIT ( ) SI_UNIT ( $, .RADIAN. ) );
#44292=ORIENTED_EDGE ( 'NONE', *, *, #183608, .T. ) ;
#44298=CARTESIAN_POINT ( 'NONE',  ( -0.4480869943418438472, 14.55305228462710687, 11.95586206503659277 ) ) ;
#44313=CARTESIAN_POINT ( 'NONE',  ( -10.19206596916605001, 3.593463588655721797, 6.350353714858171017 ) ) ;
#44353=DIRECTION ( 'NONE',  ( -1.000000000000000000, 0.000000000000000000, 3.491481338843133355E-15 ) ) ;
#44356=UNCERTAINTY_MEASURE_WITH_UNIT (LENGTH_MEASURE( 1.000000000000000082E-05 ), #30136, 'distance_accuracy_value', 'NONE');
#44368=ORIENTED_EDGE ( 'NONE', *, *, #171086, .F. ) ;
#44378=DIRECTION ( 'NONE',  ( 0.000000000000000000, 0.000000000000000000, -1.000000000000000000 ) ) ;
#44391=CARTESIAN_POINT ( 'NONE',  ( -9.348561386651960348, 4.000000000000000888, 7.001914024036569373 ) ) ;
#44401=AXIS2_PLACEMENT_3D ( 'NONE', #210910, #46312, #128699 ) ;
#44419=STYLED_ITEM ( 'NONE', ( #175518 ), #34286 ) ;
#44443=CARTESIAN_POINT ( 'NONE',  ( -0.7589079839483203749, 14.55289787277384583, 11.96588861122574521 ) ) ;
#44449=DIRECTION ( 'NONE',  ( 8.881784197001252323E-15, 0.000000000000000000, -1.000000000000000000 ) ) ;
#44478=DIRECTION ( 'NONE',  ( 7.993605777301127091E-15, 0.000000000000000000, 1.000000000000000000 ) ) ;
#44496=SURFACE_SIDE_STYLE ('',( #59654 ) ) ;
#44520=ORIENTED_EDGE ( 'NONE', *, *, #110772, .F. ) ;
#44532=CARTESIAN_POINT ( 'NONE',  ( -11.52888687719600647, 9.805768748949601488, 3.331331986263579736 ) ) ;
#44536=ADVANCED_FACE ( 'NONE', ( #63071 ), #78948, .T. ) ;
#44555=CARTESIAN_POINT ( 'NONE',  ( 1.416786528094145625, 7.999640415717673037, -11.00953083556808210 ) ) ;
#44567=EDGE_CURVE ( 'NONE', #209056, #102449, #116968, .T. ) ;
#44585=VERTEX_POINT ( 'NONE', #118281 ) ;
#44588=CARTESIAN_POINT ( 'NONE',  ( -9.797178276310326339, 4.534233751442683591, -6.931118765264285386 ) ) ;
#44613=CIRCLE ( 'NONE', #165652, 0.08000000000000020983 ) ;
#44632=B_SPLINE_CURVE_WITH_KNOTS ( 'NONE', 3,
 ( #14588, #34049, #212791, #167265, #64429, #68661, #100122, #130573, #17773, #84934, #196563, #48205, #151023, #31935, #149952, #1521 ),
 .UNSPECIFIED., .F., .F.,
 ( 4, 2, 2, 2, 2, 2, 2, 4 ),
 ( -5.999999999939666895E-08, 0.002684213935019686640, 0.004026350902529528264, 0.005368487870039371189, 0.006710624837549212379, 0.008052761805059056172, 0.009394898772568899964, 0.01073703574007874202 ),
 .UNSPECIFIED. ) ;
#44643=DIRECTION ( 'NONE',  ( 0.000000000000000000, 0.000000000000000000, -1.000000000000000000 ) ) ;
#44644=SURFACE_STYLE_FILL_AREA ( #59805 ) ;
#44713=CARTESIAN_POINT ( 'NONE',  ( -9.796852598875474882, 4.534176102514267725, -6.931574287351667252 ) ) ;
#44739=( LENGTH_UNIT ( ) NAMED_UNIT ( * ) SI_UNIT ( .MILLI., .METRE. ) );
#44772=CARTESIAN_POINT ( 'NONE',  ( 11.94105721237523277, 10.19999999999999929, -1.187919463087249827 ) ) ;
#44779=PLANE ( 'NONE',  #97705 ) ;
#44782=CARTESIAN_POINT ( 'NONE',  ( 10.26921470707188178, 10.85134567802567673, -6.214135076749980335 ) ) ;
#44794=ADVANCED_FACE ( 'NONE', ( #85710 ), #19485, .T. ) ;
#44803=CARTESIAN_POINT ( 'NONE',  ( 10.91109197447695855, 8.117831379166393191, -4.410072780793198532 ) ) ;
#44809=ORIENTED_EDGE ( 'NONE', *, *, #52849, .F. ) ;
#44825=CARTESIAN_POINT ( 'NONE',  ( 11.01135777277262306, 12.69999999999998153, 1.399999999999998579 ) ) ;
#44855=B_SPLINE_CURVE_WITH_KNOTS ( 'NONE', 3,
 ( #87215, #106724, #104546, #170591, #74180, #137045 ),
 .UNSPECIFIED., .F., .F.,
 ( 4, 2, 4 ),
 ( 0.000000000000000000, 0.5000000000000000000, 1.000000000000000000 ),
 .UNSPECIFIED. ) ;
#44857=CARTESIAN_POINT ( 'NONE',  ( -11.48806469435255373, 9.769102271275510674, -3.468902948106704631 ) ) ;
#44860=CARTESIAN_POINT ( 'NONE',  ( 0.7124089920923117880, 14.00000000000000533, 12.66466791154580207 ) ) ;
#44891=DIRECTION ( 'NONE',  ( 0.000000000000000000, 0.000000000000000000, -1.000000000000000000 ) ) ;
#44903=CARTESIAN_POINT ( 'NONE',  ( 9.056676007273772200, 14.47807714179512573, -7.134106128614786435 ) ) ;
#44906=CARTESIAN_POINT ( 'NONE',  ( 8.655308441557755472, 13.90277502934238463, 7.849885418944005266 ) ) ;
#44927=CARTESIAN_POINT ( 'NONE',  ( -9.857181934075960328, 5.275265258315555705, 6.218892358987248237 ) ) ;
#44938=CARTESIAN_POINT ( 'NONE',  ( -10.92046113480654768, 4.688422163420479016, 4.459782501114215592 ) ) ;
#44950=LINE ( 'NONE', #112135, #125283 ) ;
#44963=CARTESIAN_POINT ( 'NONE',  ( 10.85711101555931180, 9.595049302670672020, -5.123733482772419023 ) ) ;
#45009=FACE_OUTER_BOUND ( 'NONE', #131287, .T. ) ;
#45012=CARTESIAN_POINT ( 'NONE',  ( -11.81905481421901705, 13.75735655617264896, 1.592167362352176818 ) ) ;
#45021=CARTESIAN_POINT ( 'NONE',  ( -11.90610347052960627, 8.844549510192225128, 1.527030362374957262 ) ) ;
#45043=CARTESIAN_POINT ( 'NONE',  ( 11.07790593930098311, 11.29999999999999893, 0.6999999999999992895 ) ) ;
#45053=CARTESIAN_POINT ( 'NONE',  ( -12.40260256363088942, 6.580881934270854217, 3.466095386915876819 ) ) ;
#45074=DIRECTION ( 'NONE',  ( 0.000000000000000000, 0.000000000000000000, -1.000000000000000000 ) ) ;
#45076=CIRCLE ( 'NONE', #128178, 12.00000000000000355 ) ;
#45082=ORIENTED_EDGE ( 'NONE', *, *, #188457, .F. ) ;
#45098=CARTESIAN_POINT ( 'NONE',  ( 9.681502974757703939, 4.134313097118708313, 7.090028219590145397 ) ) ;
#45122=CARTESIAN_POINT ( 'NONE',  ( 3.999999999995414152E-05, 14.55305236562591098, 11.95586206891494996 ) ) ;
#45135=SURFACE_STYLE_FILL_AREA ( #194550 ) ;
#45165=UNCERTAINTY_MEASURE_WITH_UNIT (LENGTH_MEASURE( 1.000000000000000082E-05 ), #210151, 'distance_accuracy_value', 'NONE');
#45204=CARTESIAN_POINT ( 'NONE',  ( 11.78331023100045272, 9.799999999999982947, 1.799999999999999600 ) ) ;
#45206=VERTEX_POINT ( 'NONE', #18704 ) ;
#45224=DIRECTION ( 'NONE',  ( -0.8164965809277378028, 2.168827410163043206E-15, -0.5773502691896092998 ) ) ;
#45231=ORIENTED_EDGE ( 'NONE', *, *, #39272, .T. ) ;
#45257=CARTESIAN_POINT ( 'NONE',  ( 8.908442372161164968, 14.67457862154163628, -8.041203192133428601 ) ) ;
#45297=CARTESIAN_POINT ( 'NONE',  ( 7.320715180198387628, 14.46587040911547639, -9.511302536372342686 ) ) ;
#45307=CARTESIAN_POINT ( 'NONE',  ( 11.10187507031741028, 9.547320325560693988, -4.066230808108215022 ) ) ;
#45308=( GEOMETRIC_REPRESENTATION_CONTEXT ( 3 ) GLOBAL_UNCERTAINTY_ASSIGNED_CONTEXT ( ( #65671 ) ) GLOBAL_UNIT_ASSIGNED_CONTEXT ( ( #151307, #17002, #106874 ) ) REPRESENTATION_CONTEXT ( 'NONE', 'WORKASPACE' ) );
#45318=VERTEX_POINT ( 'NONE', #182275 ) ;
#45358=ORIENTED_EDGE ( 'NONE', *, *, #29782, .T. ) ;
#45359=FACE_OUTER_BOUND ( 'NONE', #153428, .T. ) ;
#45360=DIRECTION ( 'NONE',  ( -0.000000000000000000, 1.000000000000000000, 9.023263958591317418E-17 ) ) ;
#45364=DIRECTION ( 'NONE',  ( -1.000000000000000000, 0.000000000000000000, 0.000000000000000000 ) ) ;
#45372=TOROIDAL_SURFACE ( 'NONE', #38395, 11.18000000000000149, 0.08000000000000000167 ) ;
#45373=CARTESIAN_POINT ( 'NONE',  ( 10.62873463776380056, 13.79999999999999893, -3.200000000000001510 ) ) ;
#45382=CARTESIAN_POINT ( 'NONE',  ( -10.89183506716020666, 4.909321371462001871, 5.036854565707462150 ) ) ;
#45426=CARTESIAN_POINT ( 'NONE',  ( 11.41381675112453387, 13.39999999999998259, 3.704697986577180746 ) ) ;
#45434=AXIS2_PLACEMENT_3D ( 'NONE', #43378, #72648, #8714 ) ;
#45474=VERTEX_POINT ( 'NONE', #150875 ) ;
#45489=CARTESIAN_POINT ( 'NONE',  ( -11.86145016429273014, 10.90000000000000036, -1.100000000000002087 ) ) ;
#45510=CARTESIAN_POINT ( 'NONE',  ( 0.1453861984699222620, 14.53092100591740810, 11.99911925323659290 ) ) ;
#45521=ORIENTED_EDGE ( 'NONE', *, *, #191199, .F. ) ;
#45544=CARTESIAN_POINT ( 'NONE',  ( 11.52888687719590344, 12.30576874894964057, -3.331331986263459388 ) ) ;
#45546=LINE ( 'NONE', #62832, #6598 ) ;
#45557=ORIENTED_EDGE ( 'NONE', *, *, #78727, .T. ) ;
#45580=ORIENTED_EDGE ( 'NONE', *, *, #131308, .F. ) ;
#45581=CARTESIAN_POINT ( 'NONE',  ( -11.92619526248524409, 13.52744613914173932, -1.328859120100604585 ) ) ;
#45604=CARTESIAN_POINT ( 'NONE',  ( -11.96212011828583677, 9.771875549500631308, -0.9569185076418453839 ) ) ;
#45606=( NAMED_UNIT ( * ) PLANE_ANGLE_UNIT ( ) SI_UNIT ( $, .RADIAN. ) );
#45616=VERTEX_POINT ( 'NONE', #98398 ) ;
#45621=CARTESIAN_POINT ( 'NONE',  ( -11.33772467203841394, 13.50732847981850426, -3.600000000000000977 ) ) ;
#45628=DIRECTION ( 'NONE',  ( -0.000000000000000000, -1.000000000000000000, -0.000000000000000000 ) ) ;
#45637=( GEOMETRIC_REPRESENTATION_CONTEXT ( 3 ) GLOBAL_UNCERTAINTY_ASSIGNED_CONTEXT ( ( #109206 ) ) GLOBAL_UNIT_ASSIGNED_CONTEXT ( ( #79686, #212872, #130649 ) ) REPRESENTATION_CONTEXT ( 'NONE', 'WORKASPACE' ) );
#45649=VERTEX_POINT ( 'NONE', #20329 ) ;
#45655=ORIENTED_EDGE ( 'NONE', *, *, #78683, .F. ) ;
#45659=FACE_OUTER_BOUND ( 'NONE', #30980, .T. ) ;
#45666=CARTESIAN_POINT ( 'NONE',  ( -11.96215121607992415, 12.27166446219175988, 0.9565349792967585696 ) ) ;
#45672=B_SPLINE_CURVE_WITH_KNOTS ( 'NONE', 3,
 ( #140320, #139228, #172800, #204174, #203123, #73126 ),
 .UNSPECIFIED., .F., .F.,
 ( 4, 2, 4 ),
 ( 0.000000000000000000, 0.0003144386176887254184, 0.0006288772353774508368 ),
 .UNSPECIFIED. ) ;
#45692=CYLINDRICAL_SURFACE ( 'NONE', #142485, 0.3999999999999997446 ) ;
#45714=CARTESIAN_POINT ( 'NONE',  ( 0.000000000000000000, 11.29999999999998117, 0.000000000000000000 ) ) ;
#45736=ORIENTED_EDGE ( 'NONE', *, *, #213110, .T. ) ;
#45759=EDGE_CURVE ( 'NONE', #97721, #208480, #209469, .T. ) ;
#45796=CARTESIAN_POINT ( 'NONE',  ( -15.75000000000000000, 10.90000000000000036, 1.099999999999996758 ) ) ;
#45847=CARTESIAN_POINT ( 'NONE',  ( 11.15780464429275121, 9.116777561061677915, -4.430755320266929864 ) ) ;
#45866=CARTESIAN_POINT ( 'NONE',  ( 9.314578176993711267, 12.86557944855549351, 8.945654112524721313 ) ) ;
#45867=ORIENTED_EDGE ( 'NONE', *, *, #72048, .T. ) ;
#45877=ORIENTED_EDGE ( 'NONE', *, *, #59437, .F. ) ;
#45879=CARTESIAN_POINT ( 'NONE',  ( -15.75000000000000000, 13.79999999999999893, -0.7000000000000009548 ) ) ;
#45880=DIRECTION ( 'NONE',  ( 1.000000000000000000, -0.000000000000000000, -0.000000000000000000 ) ) ;
#45900=CIRCLE ( 'NONE', #194614, 0.07999999999999961309 ) ;
#45921=CARTESIAN_POINT ( 'NONE',  ( -11.41381675112460847, 10.06983264508524201, -3.704697986577268232 ) ) ;
#45924=CARTESIAN_POINT ( 'NONE',  ( -8.752560967070127873, 15.99999998464634388, 9.356054886183752473 ) ) ;
#45931=B_SPLINE_CURVE_WITH_KNOTS ( 'NONE', 3,
 ( #162240, #30099, #45297, #79900, #78831, #32229, #212019, #97248, #61529, #131902, #196856, #147067 ),
 .UNSPECIFIED., .F., .F.,
 ( 4, 2, 2, 2, 2, 4 ),
 ( 0.000000000000000000, 0.0007281235154085147036, 0.001456247030817029407, 0.001820308788521285892, 0.002184370546225541942, 0.002912494061634051876 ),
 .UNSPECIFIED. ) ;
#45967=CARTESIAN_POINT ( 'NONE',  ( 9.223659970357786619, 13.86322243015305844, -6.886736302288140266 ) ) ;
#45970=CARTESIAN_POINT ( 'NONE',  ( 8.724987196144599721, 13.71643412956232311, 7.773938044818101467 ) ) ;
#45978=CARTESIAN_POINT ( 'NONE',  ( -11.48243876534946040, 11.29999999999999893, -3.200000000000001510 ) ) ;
#46003=CARTESIAN_POINT ( 'NONE',  ( -12.93621305287376089, 7.735084883283615653, -1.079074430401041118 ) ) ;
#46028=CARTESIAN_POINT ( 'NONE',  ( 11.63116522980375578, 8.263862536643911127, 2.980981896763163608 ) ) ;
#46054=VECTOR ( 'NONE', #169829, 1000.000000000000000 ) ;
#46076=CARTESIAN_POINT ( 'NONE',  ( -11.45643882766868593, 6.922515100558133128, 3.422322265972647326 ) ) ;
#46085=CARTESIAN_POINT ( 'NONE',  ( -11.99998434469187991, 9.022909391445272931, -0.6142738339537157088 ) ) ;
#46093=EDGE_LOOP ( 'NONE', ( #151490, #193020 ) ) ;
#46106=( NAMED_UNIT ( * ) PLANE_ANGLE_UNIT ( ) SI_UNIT ( $, .RADIAN. ) );
#46117=CARTESIAN_POINT ( 'NONE',  ( -11.83624332731381124, 4.942650230196960592, 4.855242260347336192 ) ) ;
#46138=AXIS2_PLACEMENT_3D ( 'NONE', #29682, #182301, #114197 ) ;
#46146=ADVANCED_FACE ( 'NONE', ( #210945 ), #55564, .T. ) ;
#46148=CARTESIAN_POINT ( 'NONE',  ( -1.797316061902485052, 15.44822828525704850, 11.85333567385661446 ) ) ;
#46159=CARTESIAN_POINT ( 'NONE',  ( 9.574755896318485782, 4.231292707087955129, 7.158835548396386805 ) ) ;
#46167=ORIENTED_EDGE ( 'NONE', *, *, #130801, .T. ) ;
#46187=CARTESIAN_POINT ( 'NONE',  ( -10.74038358936941506, 4.109630040845076770, -4.806702709432750353 ) ) ;
#46234=DIRECTION ( 'NONE',  ( 0.000000000000000000, 0.000000000000000000, 1.000000000000000000 ) ) ;
#46265=CARTESIAN_POINT ( 'NONE',  ( -11.88168509644349058, 12.21999999999998288, 1.685788023084328513 ) ) ;
#46283=CARTESIAN_POINT ( 'NONE',  ( 11.88234649872613602, 11.25660782916751579, 0.9090484974825158160 ) ) ;
#46284=CARTESIAN_POINT ( 'NONE',  ( 9.072916337883725646, 12.13354503355262004, -7.783615223256313165 ) ) ;
#46287=CARTESIAN_POINT ( 'NONE',  ( -9.804626464733818381, 4.469082038635498577, 6.926798510140733001 ) ) ;
#46312=DIRECTION ( 'NONE',  ( 0.000000000000000000, 1.000000000000000000, 0.000000000000000000 ) ) ;
#46347=CARTESIAN_POINT ( 'NONE',  ( -9.429315115559251836, 5.003428342543706719, -6.892195246777336415 ) ) ;
#46360=CARTESIAN_POINT ( 'NONE',  ( 9.973831171035394405, 9.867947520626652036, -6.611755878741440107 ) ) ;
#46369=CARTESIAN_POINT ( 'NONE',  ( 9.963343620504341303, 12.35838256557349979, -7.799456358664951239 ) ) ;
#46370=CARTESIAN_POINT ( 'NONE',  ( -10.10575425844435138, 4.358269247758318699, 5.859476710806498900 ) ) ;
#46399=CARTESIAN_POINT ( 'NONE',  ( 1.423205080756922314, 7.980384757729337863, 10.65537363484301459 ) ) ;
#46405=ORIENTED_EDGE ( 'NONE', *, *, #39139, .T. ) ;
#46507=B_SPLINE_CURVE_WITH_KNOTS ( 'NONE', 3,
 ( #60789, #112812, #75975, #25078, #160424, #43501 ),
 .UNSPECIFIED., .F., .F.,
 ( 4, 2, 4 ),
 ( 0.000000000000000000, 0.0003205138222656014457, 0.0006410276445312028913 ),
 .UNSPECIFIED. ) ;
#46510=DIRECTION ( 'NONE',  ( 0.000000000000000000, 0.000000000000000000, 1.000000000000000000 ) ) ;
#46512=( LENGTH_UNIT ( ) NAMED_UNIT ( * ) SI_UNIT ( .MILLI., .METRE. ) );
#46523=CARTESIAN_POINT ( 'NONE',  ( -9.470186914265017464, 4.005096909781187264, 6.837150237413082365 ) ) ;
#46540=CARTESIAN_POINT ( 'NONE',  ( -11.41381675112453564, 10.06994333910004613, 3.704697986577180302 ) ) ;
#46551=ADVANCED_FACE ( 'NONE', ( #141502 ), #207510, .F. ) ;
#46566=VECTOR ( 'NONE', #47181, 1000.000000000000000 ) ;
#46572=CARTESIAN_POINT ( 'NONE',  ( -3.007794483472536307, 14.52974340527628527, 11.62584731636876789 ) ) ;
#46581=CARTESIAN_POINT ( 'NONE',  ( -11.01135777277262129, 12.69999999999998153, 1.399999999999998579 ) ) ;
#46606=CARTESIAN_POINT ( 'NONE',  ( 0.000000000000000000, 11.29999999999998117, 0.000000000000000000 ) ) ;
#46646=ORIENTED_EDGE ( 'NONE', *, *, #104111, .T. ) ;
#46648=VERTEX_POINT ( 'NONE', #29846 ) ;
#46652=FACE_OUTER_BOUND ( 'NONE', #165548, .T. ) ;
#46667=FACE_OUTER_BOUND ( 'NONE', #201122, .T. ) ;
#46669=FACE_OUTER_BOUND ( 'NONE', #12489, .T. ) ;
#46676=ORIENTED_EDGE ( 'NONE', *, *, #76035, .F. ) ;
#46682=ORIENTED_EDGE ( 'NONE', *, *, #72282, .F. ) ;
#46722=CARTESIAN_POINT ( 'NONE',  ( -9.984480469316341811, 4.552642677847350328, -6.658573114549724892 ) ) ;
#46744=CARTESIAN_POINT ( 'NONE',  ( -11.89942855770813956, 13.79999999999999893, -0.7000000000000009548 ) ) ;
#46759=FILL_AREA_STYLE_COLOUR ( '', #66341 ) ;
#46764=DIRECTION ( 'NONE',  ( -7.993605777301127091E-15, 0.000000000000000000, -1.000000000000000000 ) ) ;
#46790=CARTESIAN_POINT ( 'NONE',  ( 11.92619526913699879, 10.07218333338756722, -1.328859060402686199 ) ) ;
#46798=ORIENTED_EDGE ( 'NONE', *, *, #168648, .T. ) ;
#46848=CARTESIAN_POINT ( 'NONE',  ( 11.44800751629994906, 11.29999999999999893, -3.302956944461097777 ) ) ;
#46852=CARTESIAN_POINT ( 'NONE',  ( 0.000000000000000000, 13.88000000000000078, 0.000000000000000000 ) ) ;
#46865=( LENGTH_UNIT ( ) NAMED_UNIT ( * ) SI_UNIT ( .MILLI., .METRE. ) );
#46875=FACE_OUTER_BOUND ( 'NONE', #88999, .T. ) ;
#46886=ORIENTED_EDGE ( 'NONE', *, *, #127184, .T. ) ;
#46887=AXIS2_PLACEMENT_3D ( 'NONE', #66365, #194525, #32837 ) ;
#46922=SURFACE_STYLE_FILL_AREA ( #210450 ) ;
#46932=CARTESIAN_POINT ( 'NONE',  ( 12.65758923026637817, 7.325950736540248087, -3.630282196008513651 ) ) ;
#46942=CARTESIAN_POINT ( 'NONE',  ( 10.98545788874447560, 9.842562204520739044, 1.592267205258850238 ) ) ;
#46944=ORIENTED_EDGE ( 'NONE', *, *, #154810, .T. ) ;
#46946=DIRECTION ( 'NONE',  ( 1.000000000000000000, -0.000000000000000000, -0.000000000000000000 ) ) ;
#46947=VERTEX_POINT ( 'NONE', #80722 ) ;
#46985=CARTESIAN_POINT ( 'NONE',  ( -11.88533610222442505, 7.946055938851326772, -1.309387650900987854 ) ) ;
#46988=CARTESIAN_POINT ( 'NONE',  ( -11.86239285000045918, 12.21999999999998288, 1.812080536912751061 ) ) ;
#46999=VECTOR ( 'NONE', #20993, 1000.000000000000000 ) ;
#47017=DIRECTION ( 'NONE',  ( -0.000000000000000000, -1.000000000000000000, -0.000000000000000000 ) ) ;
#47028=AXIS2_PLACEMENT_3D ( 'NONE', #50168, #64288, #184414 ) ;
#47030=CARTESIAN_POINT ( 'NONE',  ( -11.82542156384632293, 8.168199132635775683, -2.262599552454852336 ) ) ;
#47034=CARTESIAN_POINT ( 'NONE',  ( 8.745069225198347951, 13.65147899241842744, -7.752220443290712026 ) ) ;
#47037=CARTESIAN_POINT ( 'NONE',  ( 8.060410475752370019, 13.54723888396606135, 8.643090488201771393 ) ) ;
#47069=CARTESIAN_POINT ( 'NONE',  ( -11.82198925196379946, 4.889592154110854239, -4.884635108899213485 ) ) ;
#47086=CARTESIAN_POINT ( 'NONE',  ( -9.453683584308942400, 14.52894124707535717, 7.391106286152997917 ) ) ;
#47096=CARTESIAN_POINT ( 'NONE',  ( 11.88154125640529912, 7.838767436447524162, -1.736782259460240452 ) ) ;
#47101=ORIENTED_EDGE ( 'NONE', *, *, #176346, .T. ) ;
#47147=CARTESIAN_POINT ( 'NONE',  ( -11.78331023100045627, 13.79999999999998295, 1.799999999999999600 ) ) ;
#47148=CARTESIAN_POINT ( 'NONE',  ( -11.81677561662610110, 7.791008328563874485, 1.827277289630534929 ) ) ;
#47157=CARTESIAN_POINT ( 'NONE',  ( -11.13073163568576263, 7.259140372625044080, -4.368349261952645612 ) ) ;
#47160=DIRECTION ( 'NONE',  ( 0.000000000000000000, -1.000000000000000000, 0.000000000000000000 ) ) ;
#47165=B_SPLINE_CURVE_WITH_KNOTS ( 'NONE', 3,
 ( #202647, #75871, #124710, #190669, #5500, #122588 ),
 .UNSPECIFIED., .F., .F.,
 ( 4, 2, 4 ),
 ( 0.000000000000000000, 0.0003155923098472861849, 0.0006311846196945723698 ),
 .UNSPECIFIED. ) ;
#47181=DIRECTION ( 'NONE',  ( 0.000000000000000000, -1.000000000000000000, 0.000000000000000000 ) ) ;
#47183=MECHANICAL_DESIGN_GEOMETRIC_PRESENTATION_REPRESENTATION('',(#50555),#92188);
#47190=CARTESIAN_POINT ( 'NONE',  ( -11.38502332509229831, 5.468749262791421373, -5.576278951475440948 ) ) ;
#47204=ORIENTED_EDGE ( 'NONE', *, *, #94657, .T. ) ;
#47208=CARTESIAN_POINT ( 'NONE',  ( -11.89839339040395139, 12.27122531596087818, 1.560885614203548100 ) ) ;
#47209=EDGE_CURVE ( 'NONE', #66179, #75921, #69763, .T. ) ;
#47227=CARTESIAN_POINT ( 'NONE',  ( 9.367496997597644537, 4.518459255873317204, 7.499999999999945821 ) ) ;
#47233=EDGE_CURVE ( 'NONE', #193425, #135649, #118093, .T. ) ;
#47238=VERTEX_POINT ( 'NONE', #154250 ) ;
#47255=CARTESIAN_POINT ( 'NONE',  ( 5.999999999964367170E-05, 14.55305236562399607, 11.95586206881391433 ) ) ;
#47260=CARTESIAN_POINT ( 'NONE',  ( -10.10707714348148301, 4.359868340440408829, -5.857196085253971063 ) ) ;
#47275=COLOUR_RGB ( '', 0.31764706, 0.68627451, 0.89019608) ;
#47282=VERTEX_POINT ( 'NONE', #200824 ) ;
#47337=STYLED_ITEM ( 'NONE', ( #173823 ), #143583 ) ;
#47351=EDGE_LOOP ( 'NONE', ( #144330, #36799, #78048, #192926 ) ) ;
#47356=CARTESIAN_POINT ( 'NONE',  ( 11.49097317489974834, 7.329182238404295724, -3.312691226010819889 ) ) ;
#47376=EDGE_CURVE ( 'NONE', #104947, #158693, #184563, .T. ) ;
#47396=DIRECTION ( 'NONE',  ( 1.000000000000000000, -0.000000000000000000, -0.000000000000000000 ) ) ;
#47415=ORIENTED_EDGE ( 'NONE', *, *, #93584, .F. ) ;
#47420=AXIS2_PLACEMENT_3D ( 'NONE', #214002, #96057, #46234 ) ;
#47427=ADVANCED_FACE ( 'NONE', ( #51418 ), #50346, .F. ) ;
#47444=CARTESIAN_POINT ( 'NONE',  ( 10.48924606301532592, 11.88481095883722283, -6.433727461572112283 ) ) ;
#47449=MECHANICAL_DESIGN_GEOMETRIC_PRESENTATION_REPRESENTATION('',(#71682),#89047);
#47454=CYLINDRICAL_SURFACE ( 'NONE', #117065, 0.3999999999999997446 ) ;
#47473=VECTOR ( 'NONE', #179905, 1000.000000000000000 ) ;
#47480=CARTESIAN_POINT ( 'NONE',  ( -10.37923916842784422, 4.890109552615133026, -5.358306740738790097 ) ) ;
#47594=ADVANCED_FACE ( 'NONE', ( #107698 ), #77701, .T. ) ;
#47603=EDGE_LOOP ( 'NONE', ( #201635, #170356, #8161, #79922 ) ) ;
#47606=CARTESIAN_POINT ( 'NONE',  ( 11.33772463945036790, 13.40000000000000036, -3.600000000000002309 ) ) ;
#47616=COLOUR_RGB ( '', 0.09019608, 0.27058824, 0.51372549) ;
#47625=( GEOMETRIC_REPRESENTATION_CONTEXT ( 3 ) GLOBAL_UNCERTAINTY_ASSIGNED_CONTEXT ( ( #174404 ) ) GLOBAL_UNIT_ASSIGNED_CONTEXT ( ( #188796, #206102, #56671 ) ) REPRESENTATION_CONTEXT ( 'NONE', 'WORKASPACE' ) );
#47628=CARTESIAN_POINT ( 'NONE',  ( -11.86686399458719343, 11.10928729775337054, -1.056461745586973811 ) ) ;
#47659=CARTESIAN_POINT ( 'NONE',  ( 8.210118869120222485, 14.14525406291519261, 8.752433360441910892 ) ) ;
#47699=( NAMED_UNIT ( * ) PLANE_ANGLE_UNIT ( ) SI_UNIT ( $, .RADIAN. ) );
#47701=DIRECTION ( 'NONE',  ( -0.9982742078614211811, 0.000000000000000000, 0.05872483221476467591 ) ) ;
#47737=AXIS2_PLACEMENT_3D ( 'NONE', #174060, #175117, #112297 ) ;
#47755=EDGE_CURVE ( 'NONE', #199511, #152913, #55867, .T. ) ;
#47796=CARTESIAN_POINT ( 'NONE',  ( -10.28236465222290441, 4.804674082874877072, -6.107148855343119465 ) ) ;
#47797=B_SPLINE_CURVE_WITH_KNOTS ( 'NONE', 3,
 ( #202783, #36029, #52295, #203849, #5634, #154069 ),
 .UNSPECIFIED., .F., .F.,
 ( 4, 2, 4 ),
 ( 0.001251957608719239451, 0.001565178843344208238, 0.001878400077969176810 ),
 .UNSPECIFIED. ) ;
#47806=CARTESIAN_POINT ( 'NONE',  ( 11.55950211276791251, 12.21999999999998288, 3.221476510067110777 ) ) ;
#47818=MECHANICAL_DESIGN_GEOMETRIC_PRESENTATION_REPRESENTATION('',(#213810),#41433);
#47819=CARTESIAN_POINT ( 'NONE',  ( -11.55950211276791251, 12.29999999999998472, 3.221476510067111665 ) ) ;
#47830=( NAMED_UNIT ( * ) SI_UNIT ( $, .STERADIAN. ) SOLID_ANGLE_UNIT ( ) );
#47831=CARTESIAN_POINT ( 'NONE',  ( -15.75000000000000000, 10.19999999999999929, -1.800000000000001155 ) ) ;
#47861=CARTESIAN_POINT ( 'NONE',  ( 11.94105721237523277, 12.69999999999999929, 1.187919463087244720 ) ) ;
#47863=FILL_AREA_STYLE ('',( #133378 ) ) ;
#47865=ORIENTED_EDGE ( 'NONE', *, *, #2982, .F. ) ;
#47875=CARTESIAN_POINT ( 'NONE',  ( -11.33772463945037146, 13.39999999999998259, 3.679999999999999272 ) ) ;
#47876=ORIENTED_EDGE ( 'NONE', *, *, #156690, .T. ) ;
#47878=CARTESIAN_POINT ( 'NONE',  ( -11.41381675112453387, 12.69999999999998153, 3.704697986577180746 ) ) ;
#47894=ORIENTED_EDGE ( 'NONE', *, *, #87324, .F. ) ;
#47963=CARTESIAN_POINT ( 'NONE',  ( 0.06005734137062448269, 14.50235776792163023, 11.99783618803943064 ) ) ;
#47971=CARTESIAN_POINT ( 'NONE',  ( -11.89942855770813956, 9.719999999999998863, -0.7000000000000009548 ) ) ;
#47987=FACE_OUTER_BOUND ( 'NONE', #203360, .T. ) ;
#47996=PLANE ( 'NONE',  #8444 ) ;
#48006=CARTESIAN_POINT ( 'NONE',  ( 9.936380849164404339, 11.28055779531969272, 8.367445120465268005 ) ) ;
#48008=VERTEX_POINT ( 'NONE', #96747 ) ;
#48010=ORIENTED_EDGE ( 'NONE', *, *, #203843, .F. ) ;
#48012=ORIENTED_EDGE ( 'NONE', *, *, #76439, .F. ) ;
#48021=VERTEX_POINT ( 'NONE', #61012 ) ;
#48024=CARTESIAN_POINT ( 'NONE',  ( -11.89835103415199313, 11.32893085832464308, 1.561208891256346876 ) ) ;
#48055=ORIENTED_EDGE ( 'NONE', *, *, #83136, .F. ) ;
#48061=CARTESIAN_POINT ( 'NONE',  ( -10.94892327452127034, 5.391491584528539605, 4.806427459653232148 ) ) ;
#48066=CARTESIAN_POINT ( 'NONE',  ( -11.01500063815905328, 5.353715452092881577, 4.767907905931622281 ) ) ;
#48091=DIRECTION ( 'NONE',  ( 1.000000000000000000, -0.000000000000000000, -0.000000000000000000 ) ) ;
#48107=CARTESIAN_POINT ( 'NONE',  ( 9.243053468019274632, 13.75123835987339760, -6.856199898420598515 ) ) ;
#48110=CARTESIAN_POINT ( 'NONE',  ( 8.651451850166534285, 13.72329050238413117, 9.384217411227872674 ) ) ;
#48141=CARTESIAN_POINT ( 'NONE',  ( -12.40260256363088942, 6.580881934270854217, 3.466095386915876819 ) ) ;
#48162=ORIENTED_EDGE ( 'NONE', *, *, #179732, .T. ) ;
#48169=CARTESIAN_POINT ( 'NONE',  ( 11.99956672297294880, 7.640688894226271621, 0.4526725690500942312 ) ) ;
#48202=DIRECTION ( 'NONE',  ( 0.000000000000000000, 0.000000000000000000, -1.000000000000000000 ) ) ;
#48205=CARTESIAN_POINT ( 'NONE',  ( -7.788274451701516554, 14.55185945186256724, -9.081450335369259719 ) ) ;
#48217=CARTESIAN_POINT ( 'NONE',  ( -11.95736795583652778, 7.932031143568775811, -1.043616941178784785 ) ) ;
#48226=CARTESIAN_POINT ( 'NONE',  ( -11.32370062957175172, 7.703969811881795415, -3.978908248158274930 ) ) ;
#48238=VECTOR ( 'NONE', #94832, 1000.000000000000000 ) ;
#48255=ORIENTED_EDGE ( 'NONE', *, *, #66268, .T. ) ;
#48272=CARTESIAN_POINT ( 'NONE',  ( -11.88156762547254175, 12.22000008454030073, 1.686557021358693342 ) ) ;
#48274=CARTESIAN_POINT ( 'NONE',  ( -10.50000000000000000, 13.40000000000000036, -3.600000000000002309 ) ) ;
#48275=CARTESIAN_POINT ( 'NONE',  ( 0.000000000000000000, 12.29999999999998295, 0.000000000000000000 ) ) ;
#48307=CARTESIAN_POINT ( 'NONE',  ( -1.499999999999930278, -6.071532165918824830E-15, -10.99818166789402518 ) ) ;
#48329=CARTESIAN_POINT ( 'NONE',  ( -11.84668730067608600, 12.69999999999999929, -1.400000000000001910 ) ) ;
#48333=EDGE_CURVE ( 'NONE', #159860, #123335, #93941, .T. ) ;
#48362=B_SPLINE_CURVE_WITH_KNOTS ( 'NONE', 3,
 ( #39102, #190658, #22818, #26030, #6571, #90000 ),
 .UNSPECIFIED., .F., .F.,
 ( 4, 2, 4 ),
 ( 0.000000000000000000, 0.0003258677429877276867, 0.0006517354859754553734 ),
 .UNSPECIFIED. ) ;
#48371=CIRCLE ( 'NONE', #127924, 11.95586200173889146 ) ;
#48444=EDGE_CURVE ( 'NONE', #123444, #162756, #111300, .T. ) ;
#48473=VERTEX_POINT ( 'NONE', #137763 ) ;
#48476=EDGE_LOOP ( 'NONE', ( #95415, #122101, #169640, #2791 ) ) ;
#48502=CARTESIAN_POINT ( 'NONE',  ( -1.249999999999964695, 8.500000000000000000, -10.97907099895069294 ) ) ;
#48503=CARTESIAN_POINT ( 'NONE',  ( 10.78205070141670774, 8.191904004416022289, 2.765601532466400947 ) ) ;
#48504=CARTESIAN_POINT ( 'NONE',  ( -10.44369227015510404, 5.112964020592959180, 5.232143560358712087 ) ) ;
#48513=CARTESIAN_POINT ( 'NONE',  ( 0.000000000000000000, 13.79999999999999893, 0.000000000000000000 ) ) ;
#48559=FILL_AREA_STYLE_COLOUR ( '', #44015 ) ;
#48566=ADVANCED_FACE ( 'NONE', ( #73808 ), #87929, .F. ) ;
#48651=CARTESIAN_POINT ( 'NONE',  ( -11.80248046418316044, 12.29999999999998295, 1.695421849633139466 ) ) ;
#48708=CARTESIAN_POINT ( 'NONE',  ( 8.776224899084642317, 13.27471476138782691, 8.184001253707560153 ) ) ;
#48758=B_SPLINE_CURVE_WITH_KNOTS ( 'NONE', 3,
 ( #173917, #96669, #65177, #64143, #212502, #208492 ),
 .UNSPECIFIED., .F., .F.,
 ( 4, 2, 4 ),
 ( 0.000000000000000000, 0.0003767643964918267023, 0.0007535287929836531878 ),
 .UNSPECIFIED. ) ;
#48768=CARTESIAN_POINT ( 'NONE',  ( -1.500000000000039524, 7.000000000000000000, -10.89724735885167739 ) ) ;
#48786=CARTESIAN_POINT ( 'NONE',  ( 11.48243876534946217, 9.719999999999998863, -3.200000000000001510 ) ) ;
#48791=CARTESIAN_POINT ( 'NONE',  ( -10.79708633470181134, 6.390220175058726859, -5.149361723773914434 ) ) ;
#48809=SURFACE_STYLE_USAGE ( .BOTH. , #114926 ) ;
#48841=CARTESIAN_POINT ( 'NONE',  ( -10.41369770442025633, 5.038847794253626944, -5.873885783557990514 ) ) ;
#48843=VERTEX_POINT ( 'NONE', #13056 ) ;
#48845=EDGE_CURVE ( 'NONE', #197321, #118044, #160773, .T. ) ;
#48859=STYLED_ITEM ( 'NONE', ( #18886 ), #171225 ) ;
#48872=SURFACE_SIDE_STYLE ('',( #164743 ) ) ;
#48884=ORIENTED_EDGE ( 'NONE', *, *, #213665, .T. ) ;
#48907=CARTESIAN_POINT ( 'NONE',  ( -9.645001968711920171, 4.042125922905831281, 6.587946042608958663 ) ) ;
#48908=VERTEX_POINT ( 'NONE', #212317 ) ;
#48941=CARTESIAN_POINT ( 'NONE',  ( -9.351007409486083333, 15.43944876071892125, -7.441777623099242511 ) ) ;
#48969=CARTESIAN_POINT ( 'NONE',  ( 11.35569630219380777, 11.11268439291370314, -3.554478010595023107 ) ) ;
#48988=EDGE_LOOP ( 'NONE', ( #38058, #170107, #159666, #66722, #70005, #21953 ) ) ;
#48996=VECTOR ( 'NONE', #4914, 1000.000000000000000 ) ;
#48999=ORIENTED_EDGE ( 'NONE', *, *, #98822, .F. ) ;
#49022=CARTESIAN_POINT ( 'NONE',  ( 1.250000000000037526, 8.500000000000000000, 10.97907099895068583 ) ) ;
#49028=VERTEX_POINT ( 'NONE', #88480 ) ;
#49044=PRESENTATION_STYLE_ASSIGNMENT (( #115164 ) ) ;
#49055=CARTESIAN_POINT ( 'NONE',  ( 8.484127223451739752, 12.60054268945961198, 8.443863754375202646 ) ) ;
#49068=ORIENTED_EDGE ( 'NONE', *, *, #76833, .F. ) ;
#49072=CARTESIAN_POINT ( 'NONE',  ( 11.07790593930098311, 12.30000000000000071, -0.7000000000000009548 ) ) ;
#49101=ORIENTED_EDGE ( 'NONE', *, *, #79457, .T. ) ;
#49107=APPLICATION_CONTEXT ( 'automotive_design' ) ;
#49109=CARTESIAN_POINT ( 'NONE',  ( -11.95500822865703761, 8.101291463845146978, -0.2602123231208265941 ) ) ;
#49112=CARTESIAN_POINT ( 'NONE',  ( 0.000000000000000000, 18.91999999999999815, 11.18000000000000149 ) ) ;
#49113=CARTESIAN_POINT ( 'NONE',  ( -11.57271903506312150, 7.021589676523640300, -3.181598541533452895 ) ) ;
#49137=MECHANICAL_DESIGN_GEOMETRIC_PRESENTATION_REPRESENTATION('',(#24999),#63045);
#49140=LINE ( 'NONE', #196448, #40213 ) ;
#49157=CARTESIAN_POINT ( 'NONE',  ( 9.254012853841652841, 13.68113304516277573, -6.839690896908458662 ) ) ;
#49178=CARTESIAN_POINT ( 'NONE',  ( 11.80251051724185807, 13.79999999999999893, -1.695257889419042874 ) ) ;
#49189=CARTESIAN_POINT ( 'NONE',  ( -10.71026998871754721, 6.055660674263378951, 4.667787751035539223 ) ) ;
#49203=VERTEX_POINT ( 'NONE', #116254 ) ;
#49217=CARTESIAN_POINT ( 'NONE',  ( 9.428250952287726250, 13.54490846161957052, -7.423481931054031868 ) ) ;
#49252=CARTESIAN_POINT ( 'NONE',  ( 0.000000000000000000, 13.88000000000000078, 0.000000000000000000 ) ) ;
#49266=CARTESIAN_POINT ( 'NONE',  ( -11.63072395171695028, 7.359443703391274738, -2.774425872105819035 ) ) ;
#49275=CARTESIAN_POINT ( 'NONE',  ( -11.75631475800592973, 8.608613766629060748, -2.422433509477694535 ) ) ;
#49278=DIRECTION ( 'NONE',  ( 0.000000000000000000, 1.000000000000000000, 0.000000000000000000 ) ) ;
#49283=ORIENTED_EDGE ( 'NONE', *, *, #93834, .F. ) ;
#49298=( LENGTH_UNIT ( ) NAMED_UNIT ( * ) SI_UNIT ( .MILLI., .METRE. ) );
#49322=AXIS2_PLACEMENT_3D ( 'NONE', #111540, #145081, #141883 ) ;
#49324=CARTESIAN_POINT ( 'NONE',  ( -11.81907076198591966, 12.34268775403524643, 1.592066415281218505 ) ) ;
#49332=LINE ( 'NONE', #102325, #107389 ) ;
#49363=DIRECTION ( 'NONE',  ( -1.000000000000000000, 0.000000000000000000, 0.000000000000000000 ) ) ;
#49373=ORIENTED_EDGE ( 'NONE', *, *, #831, .F. ) ;
#49383=ORIENTED_EDGE ( 'NONE', *, *, #57719, .F. ) ;
#49387=DIRECTION ( 'NONE',  ( 0.9982742078614211811, 0.000000000000000000, 0.05872483221476467591 ) ) ;
#49435=AXIS2_PLACEMENT_3D ( 'NONE', #151041, #11964, #47701 ) ;
#49445=ORIENTED_EDGE ( 'NONE', *, *, #58073, .T. ) ;
#49452=AXIS2_PLACEMENT_3D ( 'NONE', #50972, #119228, #86663 ) ;
#49466=VECTOR ( 'NONE', #9403, 1000.000000000000000 ) ;
#49497=DIRECTION ( 'NONE',  ( 1.000000000000000000, -0.000000000000000000, -0.000000000000000000 ) ) ;
#49500=DIRECTION ( 'NONE',  ( -0.9885327375000381167, 0.000000000000000000, 0.1510067114093955609 ) ) ;
#49514=( GEOMETRIC_REPRESENTATION_CONTEXT ( 3 ) GLOBAL_UNCERTAINTY_ASSIGNED_CONTEXT ( ( #23272 ) ) GLOBAL_UNIT_ASSIGNED_CONTEXT ( ( #80900, #164281, #99290 ) ) REPRESENTATION_CONTEXT ( 'NONE', 'WORKASPACE' ) );
#49524=CARTESIAN_POINT ( 'NONE',  ( -10.83922355283164407, 5.627439893072524235, -6.488667358217312220 ) ) ;
#49538=CARTESIAN_POINT ( 'NONE',  ( 9.000805734720596973, 12.35661786295821329, -7.869413734470969146 ) ) ;
#49546=CARTESIAN_POINT ( 'NONE',  ( 10.14144399767215532, 13.65493833298847548, 7.304070082181278956 ) ) ;
#49557=CARTESIAN_POINT ( 'NONE',  ( 7.104014429467876646, 14.55305237038501076, -9.619583963686880068 ) ) ;
#49560=ORIENTED_EDGE ( 'NONE', *, *, #173138, .F. ) ;
#49576=FILL_AREA_STYLE ('',( #148161 ) ) ;
#49594=FACE_OUTER_BOUND ( 'NONE', #58050, .T. ) ;
#49652=UNCERTAINTY_MEASURE_WITH_UNIT (LENGTH_MEASURE( 1.000000000000000082E-05 ), #51684, 'distance_accuracy_value', 'NONE');
#49706=PLANE ( 'NONE',  #113232 ) ;
#49728=CARTESIAN_POINT ( 'NONE',  ( 11.45846087878786612, 11.09311600781393814, 3.566076377698156996 ) ) ;
#49729=( GEOMETRIC_REPRESENTATION_CONTEXT ( 3 ) GLOBAL_UNCERTAINTY_ASSIGNED_CONTEXT ( ( #107569 ) ) GLOBAL_UNIT_ASSIGNED_CONTEXT ( ( #50152, #167110, #57621 ) ) REPRESENTATION_CONTEXT ( 'NONE', 'WORKASPACE' ) );
#49753=CARTESIAN_POINT ( 'NONE',  ( 11.41176686791169281, 12.34049196513144153, 3.404018756831826309 ) ) ;
#49760=CARTESIAN_POINT ( 'NONE',  ( 8.456790047136887978, 13.99512100581969065, 8.514254332811203696 ) ) ;
#49779=ADVANCED_FACE ( 'NONE', ( #203813 ), #145899, .T. ) ;
#49799=CARTESIAN_POINT ( 'NONE',  ( 11.89839339040395316, 9.771225315960784030, -1.560885614203536997 ) ) ;
#49816=CARTESIAN_POINT ( 'NONE',  ( -10.97030176249251276, 13.79999999999998295, 1.695215491223428739 ) ) ;
#49817=CARTESIAN_POINT ( 'NONE',  ( -10.10575425844435138, 4.358269247758318699, 5.859476710806498900 ) ) ;
#49827=CARTESIAN_POINT ( 'NONE',  ( 11.86145016429272836, 13.40000000000000036, -1.100000000000002087 ) ) ;
#49843=CARTESIAN_POINT ( 'NONE',  ( -11.94980361058168938, 10.19999999999999929, -1.100000000000000311 ) ) ;
#49891=VERTEX_POINT ( 'NONE', #209153 ) ;
#49899=EDGE_LOOP ( 'NONE', ( #102910, #49283, #129722, #161676, #106785, #127007 ) ) ;
#49907=CARTESIAN_POINT ( 'NONE',  ( -11.41126283316785361, 12.34125393091541056, -3.405403429622882783 ) ) ;
#49918=CARTESIAN_POINT ( 'NONE',  ( -8.128493925383358132, 15.44816835653746345, 8.812316018300776932 ) ) ;
#49925=ORIENTED_EDGE ( 'NONE', *, *, #79325, .T. ) ;
#49934=( LENGTH_UNIT ( ) NAMED_UNIT ( * ) SI_UNIT ( .MILLI., .METRE. ) );
#49979=EDGE_CURVE ( 'NONE', #37534, #14390, #64197, .T. ) ;
#49993=ORIENTED_EDGE ( 'NONE', *, *, #6048, .T. ) ;
#50015=CARTESIAN_POINT ( 'NONE',  ( 11.81900460097218186, 12.34242865125861854, -1.592493057836596337 ) ) ;
#50020=CARTESIAN_POINT ( 'NONE',  ( 11.92051736251533534, 12.44819756207319728, 1.381800029228856808 ) ) ;
#50025=EDGE_CURVE ( 'NONE', #104947, #144257, #201175, .T. ) ;
#50042=ORIENTED_EDGE ( 'NONE', *, *, #111757, .F. ) ;
#50048=EDGE_CURVE ( 'NONE', #59479, #130487, #208150, .T. ) ;
#50052=CARTESIAN_POINT ( 'NONE',  ( 11.86145017031113902, 11.00581953513848354, -1.100000000000000533 ) ) ;
#50054=VERTEX_POINT ( 'NONE', #180078 ) ;
#50056=( GEOMETRIC_REPRESENTATION_CONTEXT ( 3 ) GLOBAL_UNCERTAINTY_ASSIGNED_CONTEXT ( ( #662 ) ) GLOBAL_UNIT_ASSIGNED_CONTEXT ( ( #182215, #181158, #154005 ) ) REPRESENTATION_CONTEXT ( 'NONE', 'WORKASPACE' ) );
#50103=MECHANICAL_DESIGN_GEOMETRIC_PRESENTATION_REPRESENTATION('',(#133150),#15442);
#50104=CARTESIAN_POINT ( 'NONE',  ( 11.48243876534946217, 13.79999999999998295, 3.199999999999997957 ) ) ;
#50116=CARTESIAN_POINT ( 'NONE',  ( 9.295773149506796784, 12.92845620919447036, 8.961466013164043787 ) ) ;
#50126=CARTESIAN_POINT ( 'NONE',  ( 0.000000000000000000, 4.518467169708412889, 0.000000000000000000 ) ) ;
#50151=CARTESIAN_POINT ( 'NONE',  ( 11.33772463945036790, 10.19999999999999929, -3.600000000000000977 ) ) ;
#50152=( LENGTH_UNIT ( ) NAMED_UNIT ( * ) SI_UNIT ( .MILLI., .METRE. ) );
#50168=CARTESIAN_POINT ( 'NONE',  ( 0.000000000000000000, 15.44736672593543148, 0.000000000000000000 ) ) ;
#50169=B_SPLINE_CURVE_WITH_KNOTS ( 'NONE', 3,
 ( #66970, #166642, #133109, #84317, #50751, #153168 ),
 .UNSPECIFIED., .F., .F.,
 ( 4, 2, 4 ),
 ( 0.000000000000000000, 0.0003202493251089926678, 0.0006404986502179853356 ),
 .UNSPECIFIED. ) ;
#50192=SURFACE_STYLE_FILL_AREA ( #68543 ) ;
#50194=EDGE_CURVE ( 'NONE', #186645, #127188, #151091, .T. ) ;
#50257=COLOUR_RGB ( '', 0.72549020, 0.75294118, 0.79215686) ;
#50281=CARTESIAN_POINT ( 'NONE',  ( 8.444108128620271714, 14.00294857740392551, -8.463389435957207496 ) ) ;
#50320=CARTESIAN_POINT ( 'NONE',  ( -11.97302537858683991, 12.30124010191950035, -0.8111997896468238212 ) ) ;
#50333=( NAMED_UNIT ( * ) SI_UNIT ( $, .STERADIAN. ) SOLID_ANGLE_UNIT ( ) );
#50346=CYLINDRICAL_SURFACE ( 'NONE', #149251, 0.3999999999999997446 ) ;
#50372=ORIENTED_EDGE ( 'NONE', *, *, #129583, .F. ) ;
#50377=CARTESIAN_POINT ( 'NONE',  ( 11.48243876534946217, 11.29999999999998117, 3.199999999999997957 ) ) ;
#50378=DIRECTION ( 'NONE',  ( 0.8752544141058831162, 0.05606191405903982600, -0.4804027189558818245 ) ) ;
#50386=CARTESIAN_POINT ( 'NONE',  ( -1.499999999999946709, 7.750000000000000000, 15.75000000000000711 ) ) ;
#50446=SURFACE_STYLE_USAGE ( .BOTH. , #169520 ) ;
#50465=PLANE ( 'NONE',  #276 ) ;
#50494=CARTESIAN_POINT ( 'NONE',  ( -9.117697077652850979, 16.00000000001154987, -7.299999999985687715 ) ) ;
#50496=CARTESIAN_POINT ( 'NONE',  ( -10.87640920097716091, 5.776148811624420176, 6.414305308649663750 ) ) ;
#50525=FACE_OUTER_BOUND ( 'NONE', #25903, .T. ) ;
#50532=CARTESIAN_POINT ( 'NONE',  ( 11.92619526913699879, 19.00000000000000000, -1.328859060402686199 ) ) ;
#50552=FILL_AREA_STYLE ('',( #63610 ) ) ;
#50555=STYLED_ITEM ( 'NONE', ( #57321 ), #141351 ) ;
#50589=CARTESIAN_POINT ( 'NONE',  ( -9.928285507789787800, 5.423409019249701757, -6.081825614513333811 ) ) ;
#50604=CARTESIAN_POINT ( 'NONE',  ( 11.71300746584224228, 6.994125539613667897, 2.416616313326010346 ) ) ;
#50617=CARTESIAN_POINT ( 'NONE',  ( 9.476162529375914190, 12.06195001017501411, -6.315961596902559982 ) ) ;
#50632=CARTESIAN_POINT ( 'NONE',  ( 11.84668730067608600, 10.90000000000000036, -1.400000000000001910 ) ) ;
#50633=STYLED_ITEM ( 'NONE', ( #64172 ), #125288 ) ;
#50634=CARTESIAN_POINT ( 'NONE',  ( 0.008622056077349157799, 14.55305231409391808, 11.95585894185517084 ) ) ;
#50649=( BOUNDED_SURFACE ( )  B_SPLINE_SURFACE ( 3, 2, ( 
 ( #183826, #70052, #201121 ),
 ( #72192, #10140, #86334 ),
 ( #174817, #20249, #119972 ),
 ( #154543, #185949, #71123 ),
 ( #136166, #104736, #39721 ),
 ( #202184, #102587, #108791 ),
 ( #153474, #37581, #184882 ),
 ( #170782, #103665, #36507 ),
 ( #152405, #52762, #53841 ),
 ( #169713, #117835, #92506 ),
 ( #118897, #35438, #22372 ),
 ( #2916, #21303, #87410 ),
 ( #5048, #167585, #137239 ),
 ( #203261, #55973, #54904 ) ),
 .UNSPECIFIED., .F., .F., .T. ) 
 B_SPLINE_SURFACE_WITH_KNOTS ( ( 4, 2, 2, 2, 2, 2, 4 ),
 ( 3, 3 ),
 ( 0.000000000000000000, 0.002683261324918884486, 0.004024891987378326728, 0.005366522649837768971, 0.006708153312297211214, 0.008049783974756653457, 0.01073304529967553794 ),
 ( 0.000000000000000000, 1.000000000000000000 ),
 .UNSPECIFIED. ) 
 GEOMETRIC_REPRESENTATION_ITEM ( )  RATIONAL_B_SPLINE_SURFACE ( (
 ( 1.000000000000000000, 0.8509629433967599299, 1.000000000000000000),
 ( 1.000000000000000000, 0.8507446670468529204, 1.000000000000000000),
 ( 1.000000000000000000, 0.8493858944964507440, 1.000000000000000000),
 ( 1.000000000000000000, 0.8493961065500198471, 1.000000000000000000),
 ( 1.000000000000000000, 0.8496860651742271786, 1.000000000000000000),
 ( 1.000000000000000000, 0.8504612216956620729, 1.000000000000000000),
 ( 1.000000000000000000, 0.8509399017528684883, 1.000000000000000000),
 ( 1.000000000000000000, 0.8509844523289342710, 1.000000000000000000),
 ( 1.000000000000000000, 0.8505593500240633542, 1.000000000000000000),
 ( 1.000000000000000000, 0.8498310943761082648, 1.000000000000000000),
 ( 1.000000000000000000, 0.8495301021900780736, 1.000000000000000000),
 ( 1.000000000000000000, 0.8494575155450423409, 1.000000000000000000),
 ( 1.000000000000000000, 0.8507364992962466177, 1.000000000000000000),
 ( 1.000000000000000000, 0.8509629433892478279, 1.000000000000000000) ) ) 
 REPRESENTATION_ITEM ( '' )  SURFACE ( )  );
#50725=CARTESIAN_POINT ( 'NONE',  ( -11.97929049433705373, 9.719999999999998863, 0.7046979865771804130 ) ) ;
#50731=ORIENTED_EDGE ( 'NONE', *, *, #78129, .F. ) ;
#50736=SURFACE_STYLE_FILL_AREA ( #36612 ) ;
#50751=CARTESIAN_POINT ( 'NONE',  ( -10.50000000000003730, 11.00843159320399955, -3.600000000000042277 ) ) ;
#50792=ADVANCED_FACE ( 'NONE', ( #139872 ), #153973, .F. ) ;
#50819=CARTESIAN_POINT ( 'NONE',  ( 11.35605497252127449, 12.48581854048353001, 3.553547709190206572 ) ) ;
#50847=STYLED_ITEM ( 'NONE', ( #213253 ), #150547 ) ;
#50868=FACE_OUTER_BOUND ( 'NONE', #162815, .T. ) ;
#50896=( NAMED_UNIT ( * ) SI_UNIT ( $, .STERADIAN. ) SOLID_ANGLE_UNIT ( ) );
#50911=CARTESIAN_POINT ( 'NONE',  ( -11.37655908458146037, 7.827155916726787233, -3.682564549178993119 ) ) ;
#50922=ORIENTED_EDGE ( 'NONE', *, *, #80683, .F. ) ;
#50930=CARTESIAN_POINT ( 'NONE',  ( 0.000000000000000000, 19.00000000000000000, 0.000000000000000000 ) ) ;
#50933=ADVANCED_FACE ( 'NONE', ( #44020 ), #8291, .F. ) ;
#50942=( NAMED_UNIT ( * ) SI_UNIT ( $, .STERADIAN. ) SOLID_ANGLE_UNIT ( ) );
#50944=CARTESIAN_POINT ( 'NONE',  ( 1.349890321011204986, 8.200329036966268248, -10.79298809153610961 ) ) ;
#50962=PRESENTATION_STYLE_ASSIGNMENT (( #202512 ) ) ;
#50972=CARTESIAN_POINT ( 'NONE',  ( 0.000000000000000000, 7.980384757729337863, 0.000000000000000000 ) ) ;
#50984=DIRECTION ( 'NONE',  ( 0.000000000000000000, 0.000000000000000000, -1.000000000000000000 ) ) ;
#50992=ORIENTED_EDGE ( 'NONE', *, *, #93121, .T. ) ;
#51044=ORIENTED_EDGE ( 'NONE', *, *, #25664, .T. ) ;
#51108=DIRECTION ( 'NONE',  ( -0.8164965809277274778, -1.312140583148642173E-14, -0.5773502691896237327 ) ) ;
#51113=CARTESIAN_POINT ( 'NONE',  ( 0.000000000000000000, 15.44694763437329676, -11.95586206896577153 ) ) ;
#51117=AXIS2_PLACEMENT_3D ( 'NONE', #143713, #177236, #28849 ) ;
#51126=ORIENTED_EDGE ( 'NONE', *, *, #202990, .F. ) ;
#51147=CARTESIAN_POINT ( 'NONE',  ( 11.44779963594988637, 10.19999999999999929, -3.600000000000000977 ) ) ;
#51163=ORIENTED_EDGE ( 'NONE', *, *, #101713, .T. ) ;
#51168=CARTESIAN_POINT ( 'NONE',  ( -11.43645483535884999, 5.654992568747732484, -5.469194708833876817 ) ) ;
#51179=CARTESIAN_POINT ( 'NONE',  ( 9.808998241650231265, 12.88675894182173387, 8.003755498086194464 ) ) ;
#51181=VERTEX_POINT ( 'NONE', #202907 ) ;
#51192=CARTESIAN_POINT ( 'NONE',  ( -3.542975373178607779, 14.48034456167257744, 11.47372972533055524 ) ) ;
#51197=CARTESIAN_POINT ( 'NONE',  ( 11.95359438121989726, 12.49578100291300053, -1.059536798430469107 ) ) ;
#51206=VECTOR ( 'NONE', #21381, 1000.000000000000000 ) ;
#51225=ORIENTED_EDGE ( 'NONE', *, *, #75347, .F. ) ;
#51231=DIRECTION ( 'NONE',  ( -1.000000000000000000, -2.210062264950106756E-32, 1.224646799147353207E-16 ) ) ;
#51236=CARTESIAN_POINT ( 'NONE',  ( -11.32735429993228138, 6.355809303862883120, 3.965345152087539127 ) ) ;
#51251=ORIENTED_EDGE ( 'NONE', *, *, #21974, .F. ) ;
#51264=CIRCLE ( 'NONE', #78911, 0.08000000000000014044 ) ;
#51282=CARTESIAN_POINT ( 'NONE',  ( 8.253351008435402036, 13.32471229395089907, -8.566933989776503111 ) ) ;
#51288=ORIENTED_EDGE ( 'NONE', *, *, #186883, .T. ) ;
#51299=FACE_OUTER_BOUND ( 'NONE', #169695, .T. ) ;
#51339=CARTESIAN_POINT ( 'NONE',  ( 9.769029508667873785, 11.88457606340896255, -6.891197000744894829 ) ) ;
#51343=CARTESIAN_POINT ( 'NONE',  ( 11.94980361490495469, 13.50332124735856709, -1.099999952232860290 ) ) ;
#51345=( GEOMETRIC_REPRESENTATION_CONTEXT ( 3 ) GLOBAL_UNCERTAINTY_ASSIGNED_CONTEXT ( ( #62453 ) ) GLOBAL_UNIT_ASSIGNED_CONTEXT ( ( #7370, #141709, #10579 ) ) REPRESENTATION_CONTEXT ( 'NONE', 'WORKASPACE' ) );
#51352=EDGE_CURVE ( 'NONE', #131565, #36225, #124971, .T. ) ;
#51356=CARTESIAN_POINT ( 'NONE',  ( -11.91826849282518452, 10.89999999999997904, 1.399999999999998579 ) ) ;
#51382=EDGE_CURVE ( 'NONE', #187611, #177822, #43659, .T. ) ;
#51392=CARTESIAN_POINT ( 'NONE',  ( -11.97929049433705551, 12.30000000000000071, -0.7046979865771820783 ) ) ;
#51408=ORIENTED_EDGE ( 'NONE', *, *, #60871, .F. ) ;
#51418=FACE_OUTER_BOUND ( 'NONE', #149181, .T. ) ;
#51436=EDGE_LOOP ( 'NONE', ( #209795, #114593, #13668, #172813 ) ) ;
#51447=LINE ( 'NONE', #101245, #58267 ) ;
#51477=VERTEX_POINT ( 'NONE', #177912 ) ;
#51505=EDGE_CURVE ( 'NONE', #170318, #105457, #59882, .T. ) ;
#51516=CARTESIAN_POINT ( 'NONE',  ( -11.87828357749937780, 13.80310252740409283, 1.708055325888793163 ) ) ;
#51518=( NAMED_UNIT ( * ) SI_UNIT ( $, .STERADIAN. ) SOLID_ANGLE_UNIT ( ) );
#51541=UNCERTAINTY_MEASURE_WITH_UNIT (LENGTH_MEASURE( 1.000000000000000082E-05 ), #144711, 'distance_accuracy_value', 'NONE');
#51568=CARTESIAN_POINT ( 'NONE',  ( -1.724555757182347993, 14.99999999999692157, -11.68000002332616205 ) ) ;
#51570=CARTESIAN_POINT ( 'NONE',  ( -10.52284959769361805, 5.420271152154175986, 5.071911021504272199 ) ) ;
#51599=ORIENTED_EDGE ( 'NONE', *, *, #76523, .F. ) ;
#51601=FILL_AREA_STYLE ('',( #169604 ) ) ;
#51611=( NAMED_UNIT ( * ) SI_UNIT ( $, .STERADIAN. ) SOLID_ANGLE_UNIT ( ) );
#51612=FACE_OUTER_BOUND ( 'NONE', #56267, .T. ) ;
#51619=DIRECTION ( 'NONE',  ( -0.000000000000000000, -1.000000000000000000, -0.000000000000000000 ) ) ;
#51622=AXIS2_PLACEMENT_3D ( 'NONE', #168315, #53492, #164065 ) ;
#51638=ORIENTED_EDGE ( 'NONE', *, *, #72896, .T. ) ;
#51642=CARTESIAN_POINT ( 'NONE',  ( 11.97297122925985313, 9.801250793269113970, -0.8121202983519358876 ) ) ;
#51674=CARTESIAN_POINT ( 'NONE',  ( -11.25372107582773396, 4.972923339538419363, -5.839092030517418763 ) ) ;
#51684=( LENGTH_UNIT ( ) NAMED_UNIT ( * ) SI_UNIT ( .MILLI., .METRE. ) );
#51688=ORIENTED_EDGE ( 'NONE', *, *, #161732, .F. ) ;
#51691=CARTESIAN_POINT ( 'NONE',  ( 11.53430674162873260, 7.314159620192208777, 3.343773152020875106 ) ) ;
#51695=ORIENTED_EDGE ( 'NONE', *, *, #210252, .F. ) ;
#51702=CARTESIAN_POINT ( 'NONE',  ( 10.40314139648789471, 12.22719254644319697, 6.661332869700506976 ) ) ;
#51707=B_SPLINE_CURVE_WITH_KNOTS ( 'NONE', 3,
 ( #127772, #177496, #95192, #105097, #88845, #188453, #73641, #189520, #155969, #41167, #174368, #206829, #25947, #9700, #123557, #141885, #139739, #159157, #75778, #154902, #157044, #187383, #57392, #56332, #122491, #39015, #10756, #205763, #6486, #8632, #204681, #40085, #207894, #72562, #140816, #76830, #58463, #107276 ),
 .UNSPECIFIED., .F., .F.,
 ( 4, 2, 2, 2, 2, 2, 2, 2, 2, 2, 2, 2, 2, 2, 2, 2, 2, 2, 4 ),
 ( -5.999999999960951245E-08, 0.001341446902958200009, 0.002682953805916399662, 0.004024460708874599314, 0.005365967611832798967, 0.006707474514790999487, 0.008048981417749198272, 0.009390488320707397057, 0.01006124177218649905, 0.01073199522366559758, 0.01207350212662379636, 0.01341500902958199862, 0.01475651593254019914, 0.01542726938401930113, 0.01609802283549840313, 0.01743952973845660712, 0.01878103664141481111, 0.02012254354437301856, 0.02146405044733121908 ),
 .UNSPECIFIED. ) ;
#51714=CARTESIAN_POINT ( 'NONE',  ( -11.89942855770814134, 12.30000000000000071, 0.6999999999999992895 ) ) ;
#51757=( BOUNDED_SURFACE ( )  B_SPLINE_SURFACE ( 3, 2, ( 
 ( #117943, #66957, #133096 ),
 ( #53949, #120088, #199094 ),
 ( #116866, #85376, #183936 ),
 ( #186063, #35548, #169827 ),
 ( #19294, #119011, #21413 ),
 ( #124373, #157868, #73381 ) ),
 .UNSPECIFIED., .F., .F., .T. ) 
 B_SPLINE_SURFACE_WITH_KNOTS ( ( 4, 2, 4 ),
 ( 3, 3 ),
 ( -4.336808689942017736E-19, 0.0003831416164015013842, 0.0007662832328030032020 ),
 ( 0.000000000000000000, 1.000000000000000000 ),
 .UNSPECIFIED. ) 
 GEOMETRIC_REPRESENTATION_ITEM ( )  RATIONAL_B_SPLINE_SURFACE ( (
 ( 1.000000000000000000, 0.7071067811865475727, 1.000000000000000000),
 ( 1.000000000000000000, 0.6829713513653472567, 1.000000000000000000),
 ( 1.000000000000000000, 0.6534833722372194176, 1.000000000000000000),
 ( 1.000000000000000000, 0.6054027484662655167, 1.000000000000000000),
 ( 1.000000000000000000, 0.5875453974414952540, 1.000000000000000000),
 ( 1.000000000000000000, 0.5879095031487528988, 1.000000000000000000) ) ) 
 REPRESENTATION_ITEM ( '' )  SURFACE ( )  );
#51810=CARTESIAN_POINT ( 'NONE',  ( -11.89197816957260478, 9.799999999999998934, 0.8055420615339484725 ) ) ;
#51822=( NAMED_UNIT ( * ) PLANE_ANGLE_UNIT ( ) SI_UNIT ( $, .RADIAN. ) );
#51826=CARTESIAN_POINT ( 'NONE',  ( 10.56458543818803975, 8.812335408702820061, -5.705356791435097996 ) ) ;
#51841=FACE_OUTER_BOUND ( 'NONE', #202767, .T. ) ;
#51853=CARTESIAN_POINT ( 'NONE',  ( 10.97031310326519282, 12.30000000000000071, -1.695146482106562269 ) ) ;
#51879=CARTESIAN_POINT ( 'NONE',  ( 11.44779965693276402, 13.49686076798686862, 3.599999932275866676 ) ) ;
#51902=CARTESIAN_POINT ( 'NONE',  ( 8.434540686698982270, 14.01269480687351177, 8.472994457261282975 ) ) ;
#51958=DIRECTION ( 'NONE',  ( 0.5773487058764860125, 0.002327115863041261980, 0.8164943700690817652 ) ) ;
#51983=CARTESIAN_POINT ( 'NONE',  ( -10.49167311136684511, 5.343773310534622567, 5.730690286876297002 ) ) ;
#51999=DIRECTION ( 'NONE',  ( -0.000000000000000000, -1.000000000000000000, -0.000000000000000000 ) ) ;
#52000=PLANE ( 'NONE',  #143976 ) ;
#52011=PRESENTATION_STYLE_ASSIGNMENT (( #68227 ) ) ;
#52043=ORIENTED_EDGE ( 'NONE', *, *, #43445, .T. ) ;
#52051=DIRECTION ( 'NONE',  ( 0.000000000000000000, 0.000000000000000000, 1.000000000000000000 ) ) ;
#52061=DIRECTION ( 'NONE',  ( 0.000000000000000000, 0.000000000000000000, 1.000000000000000000 ) ) ;
#52064=FACE_OUTER_BOUND ( 'NONE', #51436, .T. ) ;
#52101=CARTESIAN_POINT ( 'NONE',  ( -1.423205080756851260, 7.980384757729337863, 10.65537363484302524 ) ) ;
#52108=STYLED_ITEM ( 'NONE', ( #179339 ), #169204 ) ;
#52151=CARTESIAN_POINT ( 'NONE',  ( 0.000000000000000000, 9.719999999999998863, 0.000000000000000000 ) ) ;
#52166=( GEOMETRIC_REPRESENTATION_CONTEXT ( 3 ) GLOBAL_UNCERTAINTY_ASSIGNED_CONTEXT ( ( #90449 ) ) GLOBAL_UNIT_ASSIGNED_CONTEXT ( ( #102775, #52946, #214333 ) ) REPRESENTATION_CONTEXT ( 'NONE', 'WORKASPACE' ) );
#52203=CARTESIAN_POINT ( 'NONE',  ( -15.75000000000000000, 11.29999999999999893, -1.800000000000001155 ) ) ;
#52222=EDGE_CURVE ( 'NONE', #124966, #168364, #73637, .T. ) ;
#52225=CARTESIAN_POINT ( 'NONE',  ( -11.92619525870750508, 10.07377703206319808, -1.328859154004902621 ) ) ;
#52231=CARTESIAN_POINT ( 'NONE',  ( 0.000000000000000000, 15.00041888085534758, 0.000000000000000000 ) ) ;
#52232=CARTESIAN_POINT ( 'NONE',  ( -12.26626736352559455, 6.252815285820443769, 3.851661612215340647 ) ) ;
#52243=CARTESIAN_POINT ( 'NONE',  ( 9.680359324772695118, 13.43752487939448947, 8.167046318416051776 ) ) ;
#52295=CARTESIAN_POINT ( 'NONE',  ( 11.04984958223792368, 12.49082486231873546, 1.056557932048283188 ) ) ;
#52296=DIRECTION ( 'NONE',  ( 0.000000000000000000, 0.000000000000000000, -1.000000000000000000 ) ) ;
#52300=CARTESIAN_POINT ( 'NONE',  ( -11.51269375458374000, 6.866968676300322372, -3.391140620325245880 ) ) ;
#52346=CARTESIAN_POINT ( 'NONE',  ( 7.925031528659947533, 13.65663895357722701, -8.702496307462409320 ) ) ;
#52353=ORIENTED_EDGE ( 'NONE', *, *, #57473, .T. ) ;
#52394=DIRECTION ( 'NONE',  ( 0.000000000000000000, 0.000000000000000000, 1.000000000000000000 ) ) ;
#52406=CARTESIAN_POINT ( 'NONE',  ( 11.89942855770814312, 13.79999999999999893, -0.7000000000000009548 ) ) ;
#52409=MECHANICAL_DESIGN_GEOMETRIC_PRESENTATION_REPRESENTATION('',(#197721),#73256);
#52414=CARTESIAN_POINT ( 'NONE',  ( 10.50000000000000355, 11.00718427492793161, 3.599999999999998312 ) ) ;
#52460=CARTESIAN_POINT ( 'NONE',  ( -11.37585333846683255, 7.825601127584223882, 3.684762987566864378 ) ) ;
#52465=VERTEX_POINT ( 'NONE', #100121 ) ;
#52466=AXIS2_PLACEMENT_3D ( 'NONE', #122694, #207032, #173507 ) ;
#52471=EDGE_CURVE ( 'NONE', #122534, #104947, #11323, .T. ) ;
#52475=DIRECTION ( 'NONE',  ( 1.000000000000000000, -0.000000000000000000, -0.000000000000000000 ) ) ;
#52487=ORIENTED_EDGE ( 'NONE', *, *, #103791, .F. ) ;
#52517=AXIS2_PLACEMENT_3D ( 'NONE', #8150, #41751, #91572 ) ;
#52543=SURFACE_SIDE_STYLE ('',( #126429 ) ) ;
#52547=EDGE_CURVE ( 'NONE', #201145, #181120, #183494, .T. ) ;
#52551=DIRECTION ( 'NONE',  ( 0.000000000000000000, 0.000000000000000000, 1.000000000000000000 ) ) ;
#52570=FACE_OUTER_BOUND ( 'NONE', #103666, .T. ) ;
#52587=PRESENTATION_STYLE_ASSIGNMENT (( #135982 ) ) ;
#52620=CARTESIAN_POINT ( 'NONE',  ( -7.247736482492767252, 15.00000000000521538, -10.57961706324489626 ) ) ;
#52622=CARTESIAN_POINT ( 'NONE',  ( -10.47476534206535170, 5.237283261923990629, -5.169982392003922733 ) ) ;
#52691=CARTESIAN_POINT ( 'NONE',  ( 11.86145017354043674, 10.09514365543876124, -1.100000000000000533 ) ) ;
#52721=CARTESIAN_POINT ( 'NONE',  ( -11.76696981052429614, 4.673730779118267620, -4.995440715239801044 ) ) ;
#52722=FILL_AREA_STYLE ('',( #136127 ) ) ;
#52731=CARTESIAN_POINT ( 'NONE',  ( -10.48267169704037727, 5.268073273308885973, 5.153989745587932880 ) ) ;
#52737=CARTESIAN_POINT ( 'NONE',  ( 11.49074101613450338, 7.329535750694848417, -3.313523036300598967 ) ) ;
#52749=CARTESIAN_POINT ( 'NONE',  ( 8.810850279130727714, 13.35345686061384640, -7.679452701197651443 ) ) ;
#52762=CARTESIAN_POINT ( 'NONE',  ( -5.991398640336265125, 15.46937860491462757, -10.40685062603460587 ) ) ;
#52765=CARTESIAN_POINT ( 'NONE',  ( 11.84101807917483740, 11.11021500260877382, -1.444039656437080543 ) ) ;
#52780=EDGE_CURVE ( 'NONE', #79300, #92493, #115152, .T. ) ;
#52783=ORIENTED_EDGE ( 'NONE', *, *, #44567, .F. ) ;
#52791=CARTESIAN_POINT ( 'NONE',  ( -9.497657701571187161, 14.57981886740818922, -7.334628297552537646 ) ) ;
#52801=( GEOMETRIC_REPRESENTATION_CONTEXT ( 3 ) GLOBAL_UNCERTAINTY_ASSIGNED_CONTEXT ( ( #51541 ) ) GLOBAL_UNIT_ASSIGNED_CONTEXT ( ( #144711, #177171, #210723 ) ) REPRESENTATION_CONTEXT ( 'NONE', 'WORKASPACE' ) );
#52804=CARTESIAN_POINT ( 'NONE',  ( 11.89197369110779512, 13.80000000000000249, -0.8056055387119873679 ) ) ;
#52822=VECTOR ( 'NONE', #161306, 1000.000000000000000 ) ;
#52826=ORIENTED_EDGE ( 'NONE', *, *, #184968, .T. ) ;
#52849=EDGE_CURVE ( 'NONE', #70402, #2318, #118684, .T. ) ;
#52877=CARTESIAN_POINT ( 'NONE',  ( 11.09110889797585919, 7.944360173633553401, -4.602131112445142058 ) ) ;
#52924=PRESENTATION_STYLE_ASSIGNMENT (( #3078 ) ) ;
#52946=( NAMED_UNIT ( * ) PLANE_ANGLE_UNIT ( ) SI_UNIT ( $, .RADIAN. ) );
#52968=ORIENTED_EDGE ( 'NONE', *, *, #13749, .T. ) ;
#52973=PLANE ( 'NONE',  #74745 ) ;
#52991=AXIS2_PLACEMENT_3D ( 'NONE', #193766, #212134, #31288 ) ;
#53005=ORIENTED_EDGE ( 'NONE', *, *, #96921, .F. ) ;
#53007=DIRECTION ( 'NONE',  ( 0.000000000000000000, 0.000000000000000000, -1.000000000000000000 ) ) ;
#53018=CARTESIAN_POINT ( 'NONE',  ( -11.49978884755372732, 11.24270821162817668, 3.429452816445257124 ) ) ;
#53047=CARTESIAN_POINT ( 'NONE',  ( 10.59763834280244232, 9.799999999999998934, -3.303285708550596222 ) ) ;
#53062=CARTESIAN_POINT ( 'NONE',  ( 1.499999999999959588, 8.500000000000000000, -10.89724735885168805 ) ) ;
#53063=CARTESIAN_POINT ( 'NONE',  ( -11.04536101718726293, 10.09409062111168964, -1.100000000000000311 ) ) ;
#53106=DIRECTION ( 'NONE',  ( -0.000000000000000000, 1.000000000000000000, -0.000000000000000000 ) ) ;
#53115=VERTEX_POINT ( 'NONE', #75094 ) ;
#53121=LINE ( 'NONE', #3278, #177088 ) ;
#53129=VECTOR ( 'NONE', #203836, 1000.000000000000000 ) ;
#53160=CARTESIAN_POINT ( 'NONE',  ( -10.12531724201500616, 3.239403609407997653, 5.873437370650227862 ) ) ;
#53163=UNCERTAINTY_MEASURE_WITH_UNIT (LENGTH_MEASURE( 1.000000000000000082E-05 ), #207917, 'distance_accuracy_value', 'NONE');
#53198=CARTESIAN_POINT ( 'NONE',  ( 11.78331023100045627, 13.79999999999998295, 1.799999999999999600 ) ) ;
#53212=CARTESIAN_POINT ( 'NONE',  ( -10.30773516381138855, 3.837475087047823141, -6.058016394929252257 ) ) ;
#53244=CARTESIAN_POINT ( 'NONE',  ( -9.333041836226904309, 15.44694763438996077, -7.472413793095822321 ) ) ;
#53283=EDGE_LOOP ( 'NONE', ( #167868, #163308, #30424, #119957 ) ) ;
#53293=MECHANICAL_DESIGN_GEOMETRIC_PRESENTATION_REPRESENTATION('',(#105266),#11829);
#53295=CARTESIAN_POINT ( 'NONE',  ( -10.47476631618627252, 5.237304525980054137, 5.169966676860812349 ) ) ;
#53297=CARTESIAN_POINT ( 'NONE',  ( 11.44791656467458552, 13.79999999999997939, 3.303228920649576406 ) ) ;
#53298=VECTOR ( 'NONE', #154735, 1000.000000000000000 ) ;
#53319=ORIENTED_EDGE ( 'NONE', *, *, #37763, .T. ) ;
#53321=CARTESIAN_POINT ( 'NONE',  ( 11.94105721237523277, 12.69999999999999929, -1.187919463087248939 ) ) ;
#53337=CIRCLE ( 'NONE', #143371, 11.92000000000000171 ) ;
#53346=FILL_AREA_STYLE_COLOUR ( '', #77413 ) ;
#53355=FACE_OUTER_BOUND ( 'NONE', #143186, .T. ) ;
#53356=CARTESIAN_POINT ( 'NONE',  ( -9.470186914265017464, 4.005096909781187264, 6.837150237413082365 ) ) ;
#53360=ADVANCED_FACE ( 'NONE', ( #179010 ), #201475, .T. ) ;
#53402=CARTESIAN_POINT ( 'NONE',  ( 8.111888149748871513, 13.89538954745913912, -9.737069523379568992 ) ) ;
#53410=CIRCLE ( 'NONE', #105394, 0.08000000000000040412 ) ;
#53419=CARTESIAN_POINT ( 'NONE',  ( 11.84104725192624130, 13.60983537451419778, -1.443823348526961814 ) ) ;
#53420=ORIENTED_EDGE ( 'NONE', *, *, #39019, .T. ) ;
#53431=CARTESIAN_POINT ( 'NONE',  ( -10.52284260640670688, 5.420240069097000735, -5.071998063130033430 ) ) ;
#53435=CARTESIAN_POINT ( 'NONE',  ( 7.978204059565677575, 15.27351506021529381, -8.905885731102706870 ) ) ;
#53439=COLOUR_RGB ( '', 0.66274510, 0.83137255, 0.94901961) ;
#53460=CARTESIAN_POINT ( 'NONE',  ( -15.75000000000000000, 9.799999999999982947, 3.199999999999997957 ) ) ;
#53466=CARTESIAN_POINT ( 'NONE',  ( 11.94651559118242901, 13.65130655878981791, -1.135242698369562042 ) ) ;
#53472=CARTESIAN_POINT ( 'NONE',  ( 0.000000000000000000, 13.88000000000000078, 0.000000000000000000 ) ) ;
#53475=CARTESIAN_POINT ( 'NONE',  ( 11.81907076198602802, 12.34268775403521623, -1.592066415281268243 ) ) ;
#53492=DIRECTION ( 'NONE',  ( -1.000000000000000000, 0.000000000000000000, 0.000000000000000000 ) ) ;
#53514=CARTESIAN_POINT ( 'NONE',  ( -10.99768633959234521, 5.378919375605944353, -4.807944750716973026 ) ) ;
#53525=DIRECTION ( 'NONE',  ( 0.000000000000000000, 1.000000000000000000, 0.000000000000000000 ) ) ;
#53558=ORIENTED_EDGE ( 'NONE', *, *, #68305, .T. ) ;
#53578=CARTESIAN_POINT ( 'NONE',  ( -11.40791084141324951, 7.888933430996066143, -3.732120612452610953 ) ) ;
#53579=( NAMED_UNIT ( * ) SI_UNIT ( $, .STERADIAN. ) SOLID_ANGLE_UNIT ( ) );
#53618=LINE ( 'NONE', #103438, #110380 ) ;
#53637=( LENGTH_UNIT ( ) NAMED_UNIT ( * ) SI_UNIT ( .MILLI., .METRE. ) );
#53655=DIRECTION ( 'NONE',  ( 1.000000000000000000, -0.000000000000000000, -0.000000000000000000 ) ) ;
#53689=CARTESIAN_POINT ( 'NONE',  ( -9.117697077654417726, 14.00000000001154987, -7.299999999986900079 ) ) ;
#53691=CARTESIAN_POINT ( 'NONE',  ( -11.14501278000869355, 7.223412960316487386, -3.546411330735405265 ) ) ;
#53701=( LENGTH_UNIT ( ) NAMED_UNIT ( * ) SI_UNIT ( .MILLI., .METRE. ) );
#53723=CYLINDRICAL_SURFACE ( 'NONE', #179613, 0.3999999999999997446 ) ;
#53733=CYLINDRICAL_SURFACE ( 'NONE', #125837, 11.09999999999999964 ) ;
#53747=AXIS2_PLACEMENT_3D ( 'NONE', #69873, #53655, #36324 ) ;
#53756=B_SPLINE_CURVE_WITH_KNOTS ( 'NONE', 3,
 ( #5496, #171228, #185337, #173388, #71577, #88937 ),
 .UNSPECIFIED., .F., .F.,
 ( 4, 2, 4 ),
 ( 0.000000000000000000, 0.0003779448103413554985, 0.0007558896206827109970 ),
 .UNSPECIFIED. ) ;
#53799=VECTOR ( 'NONE', #148417, 1000.000000000000000 ) ;
#53800=CARTESIAN_POINT ( 'NONE',  ( -9.748930057865852206, 3.057420161666833280, -6.444087955423147385 ) ) ;
#53801=PRESENTATION_STYLE_ASSIGNMENT (( #103622 ) ) ;
#53818=CARTESIAN_POINT ( 'NONE',  ( 11.39494474744699737, 7.467063048907871092, -3.787837880199416585 ) ) ;
#53830=CARTESIAN_POINT ( 'NONE',  ( 11.83562794788958072, 6.758279503156755297, 3.688202522935868810 ) ) ;
#53841=CARTESIAN_POINT ( 'NONE',  ( -5.991201129311522600, 15.51884043574794880, -10.40697265741862054 ) ) ;
#53843=CARTESIAN_POINT ( 'NONE',  ( -11.92046840572485777, 12.44747875205729670, -1.382231356234943309 ) ) ;
#53890=VERTEX_POINT ( 'NONE', #88970 ) ;
#53900=DIRECTION ( 'NONE',  ( -0.6249999999683966134, 6.689064965917005136E-09, 0.7806247498251027706 ) ) ;
#53949=CARTESIAN_POINT ( 'NONE',  ( 11.44800751629993130, 12.29999999999998295, 3.302956944461088451 ) ) ;
#53950=EDGE_CURVE ( 'NONE', #201145, #37826, #129092, .T. ) ;
#53952=CARTESIAN_POINT ( 'NONE',  ( 8.992125047306153363, 12.32489318961469316, -7.949360258372097476 ) ) ;
#53975=( NAMED_UNIT ( * ) PLANE_ANGLE_UNIT ( ) SI_UNIT ( $, .RADIAN. ) );
#53984=DIRECTION ( 'NONE',  ( 1.000000000000000000, -0.000000000000000000, -0.000000000000000000 ) ) ;
#53997=DIRECTION ( 'NONE',  ( 0.000000000000000000, 0.000000000000000000, 1.000000000000000000 ) ) ;
#53999=DIRECTION ( 'NONE',  ( 1.000000000000000000, -0.000000000000000000, -0.000000000000000000 ) ) ;
#54000=ORIENTED_EDGE ( 'NONE', *, *, #89762, .T. ) ;
#54023=FILL_AREA_STYLE ('',( #16157 ) ) ;
#54045=CARTESIAN_POINT ( 'NONE',  ( 9.508009452561562824, 4.000000000000000888, 7.612500000000001599 ) ) ;
#54048=ORIENTED_EDGE ( 'NONE', *, *, #109604, .F. ) ;
#54084=ORIENTED_EDGE ( 'NONE', *, *, #37600, .T. ) ;
#54110=LINE ( 'NONE', #60232, #31394 ) ;
#54119=EDGE_LOOP ( 'NONE', ( #41943, #204692, #175033, #37200 ) ) ;
#54129=CYLINDRICAL_SURFACE ( 'NONE', #8654, 12.00000000000000178 ) ;
#54154=CARTESIAN_POINT ( 'NONE',  ( -11.97185388258315086, 11.37999990720392418, 0.8311143155443556640 ) ) ;
#54188=VERTEX_POINT ( 'NONE', #76954 ) ;
#54193=CARTESIAN_POINT ( 'NONE',  ( -10.50000000000000000, 10.90000000000000036, -3.600000000000002309 ) ) ;
#54229=DIRECTION ( 'NONE',  ( 0.2275916378995520295, -0.8825604872558504566, -0.4114474847327602713 ) ) ;
#54232=CARTESIAN_POINT ( 'NONE',  ( -10.52476609942256758, 3.676887381874808902, 5.198941853688804571 ) ) ;
#54263=CARTESIAN_POINT ( 'NONE',  ( -4.836645478815604804, 15.51845284201978004, 10.99103774147543255 ) ) ;
#54274=CARTESIAN_POINT ( 'NONE',  ( 11.86685672517501899, 13.60918917859810584, 1.056525322636017172 ) ) ;
#54282=ORIENTED_EDGE ( 'NONE', *, *, #72514, .T. ) ;
#54291=DIRECTION ( 'NONE',  ( -0.000000000000000000, -1.000000000000000000, -0.000000000000000000 ) ) ;
#54315=CARTESIAN_POINT ( 'NONE',  ( -8.123305787156343882, 15.44793803671086252, -8.783211840604518983 ) ) ;
#54318=VERTEX_POINT ( 'NONE', #28219 ) ;
#54333=FACE_OUTER_BOUND ( 'NONE', #117274, .T. ) ;
#54350=( LENGTH_UNIT ( ) NAMED_UNIT ( * ) SI_UNIT ( .MILLI., .METRE. ) );
#54355=ORIENTED_EDGE ( 'NONE', *, *, #74843, .T. ) ;
#54371=ADVANCED_FACE ( 'NONE', ( #58586 ), #175551, .T. ) ;
#54382=CARTESIAN_POINT ( 'NONE',  ( 10.16976112282614508, 11.75387517088144484, 7.514388995082887490 ) ) ;
#54394=CARTESIAN_POINT ( 'NONE',  ( -11.01135777277262484, 10.09501355085105878, -1.400000000000001021 ) ) ;
#54478=CARTESIAN_POINT ( 'NONE',  ( 8.335182146949760451, 13.17516691652663319, -8.541839703048623278 ) ) ;
#54485=ORIENTED_EDGE ( 'NONE', *, *, #180841, .T. ) ;
#54506=CARTESIAN_POINT ( 'NONE',  ( -10.45142907045522129, 5.144535043903895932, -5.216774619840575333 ) ) ;
#54529=EDGE_LOOP ( 'NONE', ( #178808, #207018, #113995, #38932 ) ) ;
#54537=CARTESIAN_POINT ( 'NONE',  ( 11.86687215968023601, 13.60942212305790022, -1.056395335932036383 ) ) ;
#54544=ORIENTED_EDGE ( 'NONE', *, *, #74564, .F. ) ;
#54546=CIRCLE ( 'NONE', #19895, 0.08000000000000014044 ) ;
#54580=DIRECTION ( 'NONE',  ( -0.000000000000000000, 1.000000000000000000, -0.000000000000000000 ) ) ;
#54581=CARTESIAN_POINT ( 'NONE',  ( -11.94105721237523099, 12.69999999999999929, -1.187919463087248939 ) ) ;
#54609=EDGE_CURVE ( 'NONE', #34845, #20233, #14860, .T. ) ;
#54644=DIRECTION ( 'NONE',  ( 0.000000000000000000, 0.000000000000000000, 1.000000000000000000 ) ) ;
#54645=SURFACE_STYLE_FILL_AREA ( #34127 ) ;
#54676=DIRECTION ( 'NONE',  ( 0.000000000000000000, 0.000000000000000000, -1.000000000000000000 ) ) ;
#54682=DIRECTION ( 'NONE',  ( 0.000000000000000000, 1.000000000000000000, 0.000000000000000000 ) ) ;
#54715=DIRECTION ( 'NONE',  ( 0.000000000000000000, 0.000000000000000000, -1.000000000000000000 ) ) ;
#54729=CARTESIAN_POINT ( 'NONE',  ( -10.51582573219070227, 11.11290858478269783, 3.554376768052134317 ) ) ;
#54734=VECTOR ( 'NONE', #208773, 1000.000000000000000 ) ;
#54757=CARTESIAN_POINT ( 'NONE',  ( -10.02504487015220569, 5.769816241140256707, -5.888073156868665059 ) ) ;
#54777=CARTESIAN_POINT ( 'NONE',  ( -10.40218499402273800, 5.060399005975109610, 5.893486624065884527 ) ) ;
#54803=CIRCLE ( 'NONE', #186204, 0.08000000000000040412 ) ;
#54861=VERTEX_POINT ( 'NONE', #110640 ) ;
#54866=CARTESIAN_POINT ( 'NONE',  ( -10.81809272050965376, 3.158133435639066899, -6.646723133134004868 ) ) ;
#54880=ORIENTED_EDGE ( 'NONE', *, *, #134668, .T. ) ;
#54882=CARTESIAN_POINT ( 'NONE',  ( 11.99989233169111991, 6.624601663682995856, 0.5005250340842011259 ) ) ;
#54896=( BOUNDED_SURFACE ( )  B_SPLINE_SURFACE ( 3, 2, ( 
 ( #60927, #83279, #58791 ),
 ( #17204, #126008, #29504 ),
 ( #145429, #49728, #115857 ),
 ( #33478, #99551, #165615 ),
 ( #144362, #93455, #194120 ),
 ( #207167, #193047, #143289 ) ),
 .UNSPECIFIED., .F., .F., .F. ) 
 B_SPLINE_SURFACE_WITH_KNOTS ( ( 4, 2, 4 ),
 ( 3, 3 ),
 ( 0.000000000000000000, 0.0003831327362561329415, 0.0007662654725122658829 ),
 ( 0.000000000000000000, 1.000000000000000000 ),
 .UNSPECIFIED. ) 
 GEOMETRIC_REPRESENTATION_ITEM ( )  RATIONAL_B_SPLINE_SURFACE ( (
 ( 1.000000000000000000, 0.5879095031487664436, 1.000000000000000000),
 ( 1.000000000000000000, 0.5873691247590056008, 1.000000000000000000),
 ( 1.000000000000000000, 0.6054349545482283768, 1.000000000000000000),
 ( 1.000000000000000000, 0.6533334602781794009, 1.000000000000000000),
 ( 1.000000000000000000, 0.6828746263139577888, 1.000000000000000000),
 ( 1.000000000000000000, 0.7071067811865475727, 1.000000000000000000) ) ) 
 REPRESENTATION_ITEM ( '' )  SURFACE ( )  );
#54904=CARTESIAN_POINT ( 'NONE',  ( -9.367496996292747014, 15.51845925589211106, -7.500000001629759439 ) ) ;
#54909=EDGE_CURVE ( 'NONE', #30835, #156842, #63945, .T. ) ;
#54947=DIRECTION ( 'NONE',  ( 1.000000000000000000, -0.000000000000000000, -0.000000000000000000 ) ) ;
#54951=CARTESIAN_POINT ( 'NONE',  ( -10.39336823037077195, 4.932734307774878424, -5.330979603150785451 ) ) ;
#54979=DIRECTION ( 'NONE',  ( 1.000000000000000000, -0.000000000000000000, -0.000000000000000000 ) ) ;
#55009=ORIENTED_EDGE ( 'NONE', *, *, #75599, .T. ) ;
#55036=EDGE_CURVE ( 'NONE', #200044, #61984, #152932, .T. ) ;
#55069=( NAMED_UNIT ( * ) PLANE_ANGLE_UNIT ( ) SI_UNIT ( $, .RADIAN. ) );
#55101=CARTESIAN_POINT ( 'NONE',  ( -11.84668730067608244, 10.09363775091779125, 1.399999999999998357 ) ) ;
#55114=CARTESIAN_POINT ( 'NONE',  ( -9.340702556249549815, 15.44694763438218033, -7.462845556860568941 ) ) ;
#55136=CARTESIAN_POINT ( 'NONE',  ( -11.91292854676714974, 9.985184703269748496, 1.446370920797324100 ) ) ;
#55143=LINE ( 'NONE', #103900, #35328 ) ;
#55152=CARTESIAN_POINT ( 'NONE',  ( -11.16150260363039060, 4.727604019697102977, 6.014961758122009172 ) ) ;
#55168=DIRECTION ( 'NONE',  ( 0.6250000000674432732, -1.452638498762078799E-08, 0.7806247497458018714 ) ) ;
#55182=CARTESIAN_POINT ( 'NONE',  ( -0.9015567080380649800, 15.51893790258581518, -11.97447543335910503 ) ) ;
#55183=CARTESIAN_POINT ( 'NONE',  ( -8.784717086998243829, 14.48107293590954825, 8.187136581970905880 ) ) ;
#55190=( LENGTH_UNIT ( ) NAMED_UNIT ( * ) SI_UNIT ( .MILLI., .METRE. ) );
#55200=ADVANCED_FACE ( 'NONE', ( #176279 ), #77693, .F. ) ;
#55202=CARTESIAN_POINT ( 'NONE',  ( -1.500000000000038636, 7.750000000000000000, -10.64483442802187341 ) ) ;
#55223=ORIENTED_EDGE ( 'NONE', *, *, #123377, .T. ) ;
#55250=CARTESIAN_POINT ( 'NONE',  ( -3.505115903893319729, 15.47003409145715480, 11.48545873523604044 ) ) ;
#55296=DIRECTION ( 'NONE',  ( -0.000000000000000000, -1.000000000000000000, -0.000000000000000000 ) ) ;
#55297=CARTESIAN_POINT ( 'NONE',  ( -10.73969341588288628, 4.108126672274917013, 4.807887712954548753 ) ) ;
#55301=UNCERTAINTY_MEASURE_WITH_UNIT (LENGTH_MEASURE( 1.000000000000000082E-05 ), #165748, 'distance_accuracy_value', 'NONE');
#55312=EDGE_LOOP ( 'NONE', ( #19136, #133945, #154951, #81296, #20354, #25235, #31625, #75932 ) ) ;
#55313=SURFACE_STYLE_USAGE ( .BOTH. , #190621 ) ;
#55345=CARTESIAN_POINT ( 'NONE',  ( -9.756440972247897747, 3.530925782592636342, -6.991133065687681558 ) ) ;
#55369=ORIENTED_EDGE ( 'NONE', *, *, #93908, .F. ) ;
#55376=CARTESIAN_POINT ( 'NONE',  ( -1.734723475976807094E-15, 4.000007913748543587, -12.17999999982603399 ) ) ;
#55386=VERTEX_POINT ( 'NONE', #17997 ) ;
#55391=FACE_BOUND ( 'NONE', #179032, .T. ) ;
#55397=CARTESIAN_POINT ( 'NONE',  ( 1.727399429735891272E-15, 14.67582449756711149, 11.75119994318007421 ) ) ;
#55407=ADVANCED_FACE ( 'NONE', ( #50525 ), #122286, .T. ) ;
#55429=CARTESIAN_POINT ( 'NONE',  ( -10.45911050446410506, 5.175404930453152197, 5.201426885097844455 ) ) ;
#55470=( BOUNDED_SURFACE ( )  B_SPLINE_SURFACE ( 3, 2, ( 
 ( #121609, #187579, #53321 ),
 ( #167084, #102074, #133545 ),
 ( #169202, #51197, #34921 ),
 ( #202745, #18675, #151900 ),
 ( #184373, #118385, #168140 ),
 ( #19741, #85821, #119454 ) ),
 .UNSPECIFIED., .F., .F., .T. ) 
 B_SPLINE_SURFACE_WITH_KNOTS ( ( 4, 2, 4 ),
 ( 3, 3 ),
 ( 0.000000000000000000, 0.0003754691837024766985, 0.0007509383674049533971 ),
 ( 0.000000000000000000, 1.000000000000000000 ),
 .UNSPECIFIED. ) 
 GEOMETRIC_REPRESENTATION_ITEM ( )  RATIONAL_B_SPLINE_SURFACE ( (
 ( 1.000000000000000000, 0.6711954675835395401, 1.000000000000000000),
 ( 1.000000000000000000, 0.6709646295267174265, 1.000000000000000000),
 ( 1.000000000000000000, 0.6771840716659688342, 1.000000000000000000),
 ( 1.000000000000000000, 0.6927481755866825575, 1.000000000000000000),
 ( 1.000000000000000000, 0.7017972101310403499, 1.000000000000000000),
 ( 1.000000000000000000, 0.7071067811865475727, 1.000000000000000000) ) ) 
 REPRESENTATION_ITEM ( '' )  SURFACE ( )  );
#55484=CARTESIAN_POINT ( 'NONE',  ( 0.000000000000000000, 11.37999999999999901, 0.000000000000000000 ) ) ;
#55487=ORIENTED_EDGE ( 'NONE', *, *, #648, .F. ) ;
#55489=EDGE_CURVE ( 'NONE', #195372, #24390, #73798, .T. ) ;
#55490=ORIENTED_EDGE ( 'NONE', *, *, #122495, .T. ) ;
#55494=CARTESIAN_POINT ( 'NONE',  ( -1.423205080756925867, 7.980384757729337863, -10.65537363484301636 ) ) ;
#55514=ORIENTED_EDGE ( 'NONE', *, *, #71209, .F. ) ;
#55539=CARTESIAN_POINT ( 'NONE',  ( -11.33772463945037146, 13.39999999999998259, 3.599999999999999201 ) ) ;
#55552=VERTEX_POINT ( 'NONE', #57996 ) ;
#55554=CARTESIAN_POINT ( 'NONE',  ( 0.000000000000000000, 19.00000000000000000, 0.000000000000000000 ) ) ;
#55564=( BOUNDED_SURFACE ( )  B_SPLINE_SURFACE ( 3, 3, ( 
 ( #13814, #114599, #179541, #62570, #31161, #82019, #79886, #131887, #63648, #198945, #83076, #181642, #178474, #32213, #116713, #97234 ),
 ( #162227, #80959, #180590, #98287, #128733, #50589, #164348, #182713, #148109, #161155, #214112, #194707, #197895, #46347, #733, #65739 ),
 ( #49524, #115646, #30085, #33269, #99354, #17001, #149154, #6084, #85219, #200022, #117795, #151306, #104694, #136126, #86294, #102542 ),
 ( #204277, #2875, #5007, #51674, #137198, #38617, #35395, #68945, #101472, #36468, #118854, #183787, #185907, #21261, #168606, #100406 ),
 ( #52721, #1810, #72155, #122088, #55933, #34331, #167543, #88445, #203222, #20207, #54866, #184837, #154506, #71081, #18066, #166474 ),
 ( #201080, #152364, #67868, #3942, #70010, #202140, #121019, #19143, #135067, #37542, #103621, #53800, #138264, #119931, #84154, #169674 ),
 ( #87367, #153436, #186985, #150241, #170745, #134015, #22330, #155573, #27699, #173983, #140422, #25555, #158773, #142553, #143631, #77511 ) ),
 .UNSPECIFIED., .T., .F., .T. ) 
 B_SPLINE_SURFACE_WITH_KNOTS ( ( 4, 3, 4 ),
 ( 4, 2, 2, 2, 2, 2, 2, 4 ),
 ( 0.000000000000000000, 0.5000000000000000000, 1.000000000000000000 ),
 ( 0.6095821870314059865, 0.6120980958896804491, 0.6146140047479549118, 0.6196458224645037260, 0.6297094578976014656, 0.6397880689092279027, 0.6448273744150412323, 0.6498666799208544509 ),
 .UNSPECIFIED. ) 
 GEOMETRIC_REPRESENTATION_ITEM ( )  RATIONAL_B_SPLINE_SURFACE ( (
 ( 1.000000000000000000, 1.000000000000000000, 1.000000000000000000, 1.000000000000000000, 1.000000000000000000, 1.000000000000000000, 1.000000000000000000, 1.000000000000000000, 1.000000000000000000, 1.000000000000000000, 1.000000000000000000, 1.000000000000000000, 1.000000000000000000, 1.000000000000000000, 1.000000000000000000, 1.000000000000000000),
 ( 0.3333333333333333703, 0.3333333333333333703, 0.3333333333333333703, 0.3333333333333333703, 0.3333333333333333703, 0.3333333333333333703, 0.3333333333333333703, 0.3333333333333333703, 0.3333333333333333703, 0.3333333333333333703, 0.3333333333333333703, 0.3333333333333333703, 0.3333333333333333703, 0.3333333333333333703, 0.3333333333333333703, 0.3333333333333333703),
 ( 0.3333333333333333703, 0.3333333333333333703, 0.3333333333333333703, 0.3333333333333333703, 0.3333333333333333703, 0.3333333333333333703, 0.3333333333333333703, 0.3333333333333333703, 0.3333333333333333703, 0.3333333333333333703, 0.3333333333333333703, 0.3333333333333333703, 0.3333333333333333703, 0.3333333333333333703, 0.3333333333333333703, 0.3333333333333333703),
 ( 1.000000000000000000, 1.000000000000000000, 1.000000000000000000, 1.000000000000000000, 1.000000000000000000, 1.000000000000000000, 1.000000000000000000, 1.000000000000000000, 1.000000000000000000, 1.000000000000000000, 1.000000000000000000, 1.000000000000000000, 1.000000000000000000, 1.000000000000000000, 1.000000000000000000, 1.000000000000000000),
 ( 0.3333333333333333703, 0.3333333333333333703, 0.3333333333333333703, 0.3333333333333333703, 0.3333333333333333703, 0.3333333333333333703, 0.3333333333333333703, 0.3333333333333333703, 0.3333333333333333703, 0.3333333333333333703, 0.3333333333333333703, 0.3333333333333333703, 0.3333333333333333703, 0.3333333333333333703, 0.3333333333333333703, 0.3333333333333333703),
 ( 0.3333333333333333703, 0.3333333333333333703, 0.3333333333333333703, 0.3333333333333333703, 0.3333333333333333703, 0.3333333333333333703, 0.3333333333333333703, 0.3333333333333333703, 0.3333333333333333703, 0.3333333333333333703, 0.3333333333333333703, 0.3333333333333333703, 0.3333333333333333703, 0.3333333333333333703, 0.3333333333333333703, 0.3333333333333333703),
 ( 1.000000000000000000, 1.000000000000000000, 1.000000000000000000, 1.000000000000000000, 1.000000000000000000, 1.000000000000000000, 1.000000000000000000, 1.000000000000000000, 1.000000000000000000, 1.000000000000000000, 1.000000000000000000, 1.000000000000000000, 1.000000000000000000, 1.000000000000000000, 1.000000000000000000, 1.000000000000000000) ) ) 
 REPRESENTATION_ITEM ( '' )  SURFACE ( )  );
#55593=ORIENTED_EDGE ( 'NONE', *, *, #208559, .T. ) ;
#55607=DIRECTION ( 'NONE',  ( -0.6249999999996199707, 4.211139888037421403E-14, -0.7806247498001041007 ) ) ;
#55636=CARTESIAN_POINT ( 'NONE',  ( -15.75000000000000000, 12.69999999999999929, -3.600000000000000977 ) ) ;
#55681=EDGE_CURVE ( 'NONE', #211051, #127758, #1097, .T. ) ;
#55685=CARTESIAN_POINT ( 'NONE',  ( -9.086263084862915562, 14.48154074114212797, -7.851261044451125493 ) ) ;
#55697=CARTESIAN_POINT ( 'NONE',  ( 9.601861708076905089, 3.883749503203147047, -7.121442012218629714 ) ) ;
#55709=COLOUR_RGB ( '', 0.72549020, 0.75294118, 0.79215686) ;
#55710=CARTESIAN_POINT ( 'NONE',  ( -11.75936552431323179, 8.614003048789559358, 2.408008290394755058 ) ) ;
#55761=( NAMED_UNIT ( * ) PLANE_ANGLE_UNIT ( ) SI_UNIT ( $, .RADIAN. ) );
#55768=CARTESIAN_POINT ( 'NONE',  ( 11.94105721237523277, 10.19999999999999929, -1.187919463087249827 ) ) ;
#55779=CARTESIAN_POINT ( 'NONE',  ( 1.469576158976823947E-15, 15.00000000000000000, 12.00000000000000178 ) ) ;
#55786=CARTESIAN_POINT ( 'NONE',  ( 10.12955225396220271, 13.73833855058678743, 7.326689838346525541 ) ) ;
#55803=AXIS2_PLACEMENT_3D ( 'NONE', #167300, #2626, #103362 ) ;
#55808=CARTESIAN_POINT ( 'NONE',  ( 11.97929049433705551, 9.799999999999997158, 0.7046979865771803020 ) ) ;
#55821=CARTESIAN_POINT ( 'NONE',  ( -11.36817070414822695, 5.406007704794011381, -5.610921796774237968 ) ) ;
#55822=COLOUR_RGB ( '', 0.31764706, 0.68627451, 0.89019608) ;
#55827=ADVANCED_FACE ( 'NONE', ( #72087 ), #202073, .T. ) ;
#55831=SURFACE_STYLE_USAGE ( .BOTH. , #22228 ) ;
#55841=LINE ( 'NONE', #172809, #136039 ) ;
#55845=EDGE_LOOP ( 'NONE', ( #33638, #199869, #73402, #157347, #185354, #80881, #21665, #101202 ) ) ;
#55852=DIRECTION ( 'NONE',  ( 0.000000000000000000, 1.000000000000000000, 0.000000000000000000 ) ) ;
#55867=CIRCLE ( 'NONE', #176938, 0.08000000000000040412 ) ;
#55924=B_SPLINE_CURVE_WITH_KNOTS ( 'NONE', 3,
 ( #27509, #195356, #113104, #14443, #11251, #77329 ),
 .UNSPECIFIED., .F., .F.,
 ( 4, 2, 4 ),
 ( 0.000000000000000000, 0.0003258677429877275783, 0.0006517354859754551566 ),
 .UNSPECIFIED. ) ;
#55927=ADVANCED_FACE ( 'NONE', ( #156580, #90515, #171743, #86230, #23340, #8173, #155502, #74257 ), #53733, .F. ) ;
#55929=AXIS2_PLACEMENT_3D ( 'NONE', #25266, #175810, #131106 ) ;
#55933=CARTESIAN_POINT ( 'NONE',  ( -11.66942904513850543, 4.336835040752899495, -5.185078083676367910 ) ) ;
#55944=CARTESIAN_POINT ( 'NONE',  ( -10.45911201557330195, 5.175391108250987138, -5.201428006079835242 ) ) ;
#55950=CARTESIAN_POINT ( 'NONE',  ( 8.989385892795640487, 12.33334389077627335, 7.952349317847390076 ) ) ;
#55973=CARTESIAN_POINT ( 'NONE',  ( -9.367496997192910513, 15.46908218390266043, -7.500000000505454345 ) ) ;
#56020=CARTESIAN_POINT ( 'NONE',  ( -9.912197829101469182, 5.385002637010017246, -6.113573717307969169 ) ) ;
#56021=VECTOR ( 'NONE', #124616, 1000.000000000000000 ) ;
#56024=LINE ( 'NONE', #185998, #176593 ) ;
#56028=ORIENTED_EDGE ( 'NONE', *, *, #167754, .F. ) ;
#56031=CARTESIAN_POINT ( 'NONE',  ( 11.89942855770814312, 13.88000000000000078, -0.7000000000000009548 ) ) ;
#56046=PRESENTATION_STYLE_ASSIGNMENT (( #205478 ) ) ;
#56136=SURFACE_SIDE_STYLE ('',( #142760 ) ) ;
#56140=CARTESIAN_POINT ( 'NONE',  ( 11.78331023100045627, 12.21999999999998288, 1.799999999999999600 ) ) ;
#56174=VECTOR ( 'NONE', #144385, 1000.000000000000000 ) ;
#56195=EDGE_CURVE ( 'NONE', #95365, #210028, #28965, .T. ) ;
#56218=CARTESIAN_POINT ( 'NONE',  ( -10.83925572545687999, 5.627432043407305962, 6.488667418600654102 ) ) ;
#56233=VECTOR ( 'NONE', #64652, 1000.000000000000000 ) ;
#56249=CARTESIAN_POINT ( 'NONE',  ( -6.748402495618347707, 15.51952511201470841, -9.932705302265116387 ) ) ;
#56250=CARTESIAN_POINT ( 'NONE',  ( -4.796985430826090635, 14.48151950780699693, 11.00853662041797598 ) ) ;
#56258=DIRECTION ( 'NONE',  ( 0.3162277660168373861, -0.9486832980505139901, 0.000000000000000000 ) ) ;
#56262=CYLINDRICAL_SURFACE ( 'NONE', #33226, 0.3999999999999996336 ) ;
#56267=EDGE_LOOP ( 'NONE', ( #91338, #203666, #21572, #80382 ) ) ;
#56268=AXIS2_PLACEMENT_3D ( 'NONE', #50126, #116247, #117313 ) ;
#56269=FILL_AREA_STYLE_COLOUR ( '', #81137 ) ;
#56287=DIRECTION ( 'NONE',  ( 0.2684563758389304500, -5.821219718043054220E-15, -0.9632918427306581544 ) ) ;
#56296=CARTESIAN_POINT ( 'NONE',  ( 1.474311205794113012E-15, 15.00000000000000355, 11.68000000000000504 ) ) ;
#56315=CARTESIAN_POINT ( 'NONE',  ( -11.84668730067608600, 19.00000000000000000, 1.319999999999998286 ) ) ;
#56317=CARTESIAN_POINT ( 'NONE',  ( -11.33772463945036968, 13.40000000000000036, -3.600000000000002309 ) ) ;
#56325=ORIENTED_EDGE ( 'NONE', *, *, #183211, .F. ) ;
#56332=CARTESIAN_POINT ( 'NONE',  ( 11.57674487772738914, 8.193752454921764183, 2.992692998337922461 ) ) ;
#56361=CARTESIAN_POINT ( 'NONE',  ( -11.27970626620888517, 5.059847508428347851, 5.788342990380983544 ) ) ;
#56390=EDGE_CURVE ( 'NONE', #53890, #197321, #21958, .T. ) ;
#56404=CARTESIAN_POINT ( 'NONE',  ( 11.86145017354087372, 13.50485634456124551, 1.099999999999996980 ) ) ;
#56414=CARTESIAN_POINT ( 'NONE',  ( -9.333041836230018262, 14.55305236562984383, 7.472413793098201751 ) ) ;
#56450=ORIENTED_EDGE ( 'NONE', *, *, #2314, .T. ) ;
#56481=DIRECTION ( 'NONE',  ( -0.000000000000000000, 1.000000000000000000, 9.023263958591317418E-17 ) ) ;
#56484=ORIENTED_EDGE ( 'NONE', *, *, #160843, .F. ) ;
#56491=AXIS2_PLACEMENT_3D ( 'NONE', #36403, #169613, #187986 ) ;
#56500=CARTESIAN_POINT ( 'NONE',  ( -10.96033999287893224, 4.843182460328104177, 4.379153535238802242 ) ) ;
#56502=CARTESIAN_POINT ( 'NONE',  ( 7.825489347732291989, 14.97139610117899444, 9.977962224420885207 ) ) ;
#56508=DIRECTION ( 'NONE',  ( 0.5773502691896272854, 0.000000000000000000, -0.8164965809277250353 ) ) ;
#56544=AXIS2_PLACEMENT_3D ( 'NONE', #39496, #138078, #172714 ) ;
#56545=TOROIDAL_SURFACE ( 'NONE', #194914, 11.92000000000000171, 0.08000000000000000167 ) ;
#56574=( NAMED_UNIT ( * ) PLANE_ANGLE_UNIT ( ) SI_UNIT ( $, .RADIAN. ) );
#56620=VERTEX_POINT ( 'NONE', #56683 ) ;
#56633=AXIS2_PLACEMENT_3D ( 'NONE', #68457, #35972, #165981 ) ;
#56636=CIRCLE ( 'NONE', #8227, 12.00000000000000178 ) ;
#56671=( NAMED_UNIT ( * ) SI_UNIT ( $, .STERADIAN. ) SOLID_ANGLE_UNIT ( ) );
#56672=CARTESIAN_POINT ( 'NONE',  ( -10.99878419127389684, 6.872217442641685103, 3.961452310287494338 ) ) ;
#56677=CARTESIAN_POINT ( 'NONE',  ( -8.803107927929307408, 14.53091780748839490, -8.204921721742058693 ) ) ;
#56683=CARTESIAN_POINT ( 'NONE',  ( 11.84668730067608600, 12.69999999999998153, 1.399999999999998579 ) ) ;
#56684=EDGE_LOOP ( 'NONE', ( #61919, #40395, #81230, #38076 ) ) ;
#56711=DIRECTION ( 'NONE',  ( 0.000000000000000000, 0.000000000000000000, -1.000000000000000000 ) ) ;
#56729=CARTESIAN_POINT ( 'NONE',  ( -11.55950211276791251, 11.37999999999999901, -3.221476510067115662 ) ) ;
#56745=CARTESIAN_POINT ( 'NONE',  ( 11.84668730067608600, 10.19999999999999929, -1.400000000000001910 ) ) ;
#56757=EDGE_CURVE ( 'NONE', #198330, #151228, #56636, .T. ) ;
#56770=ORIENTED_EDGE ( 'NONE', *, *, #182687, .F. ) ;
#56781=CARTESIAN_POINT ( 'NONE',  ( -11.07041934583884313, 7.106884258450539171, -4.635831715794138219 ) ) ;
#56806=DIRECTION ( 'NONE',  ( -0.000000000000000000, -1.000000000000000000, 0.000000000000000000 ) ) ;
#56811=EDGE_CURVE ( 'NONE', #204988, #195372, #108696, .T. ) ;
#56819=( BOUNDED_SURFACE ( )  B_SPLINE_SURFACE ( 3, 2, ( 
 ( #180561, #98259, #65710 ),
 ( #52691, #84125, #150211 ),
 ( #164316, #1783, #67840 ),
 ( #133986, #81989, #148077 ),
 ( #199993, #51642, #117766 ),
 ( #118820, #131858, #197865 ) ),
 .UNSPECIFIED., .F., .F., .T. ) 
 B_SPLINE_SURFACE_WITH_KNOTS ( ( 4, 2, 4 ),
 ( 3, 3 ),
 ( 0.000000000000000000, 0.0003754691837024766985, 0.0007509383674049533971 ),
 ( 0.000000000000000000, 1.000000000000000000 ),
 .UNSPECIFIED. ) 
 GEOMETRIC_REPRESENTATION_ITEM ( )  RATIONAL_B_SPLINE_SURFACE ( (
 ( 1.000000000000000000, 0.6711954675835395401, 1.000000000000000000),
 ( 1.000000000000000000, 0.6709646295267174265, 1.000000000000000000),
 ( 1.000000000000000000, 0.6771840716659688342, 1.000000000000000000),
 ( 1.000000000000000000, 0.6927481755866825575, 1.000000000000000000),
 ( 1.000000000000000000, 0.7017972101310361310, 1.000000000000000000),
 ( 1.000000000000000000, 0.7071067811865475727, 1.000000000000000000) ) ) 
 REPRESENTATION_ITEM ( '' )  SURFACE ( )  );
#56857=FACE_OUTER_BOUND ( 'NONE', #15459, .T. ) ;
#56859=CARTESIAN_POINT ( 'NONE',  ( 7.292702578216013976, 15.96614424547465205, 9.125377228003427987 ) ) ;
#56878=CARTESIAN_POINT ( 'NONE',  ( 11.88237264505823987, 9.843229615316822390, 0.9087825512662162097 ) ) ;
#56892=CARTESIAN_POINT ( 'NONE',  ( -12.46228870304231329, 8.331136472732479703, -2.451782011337487965 ) ) ;
#56902=ORIENTED_EDGE ( 'NONE', *, *, #120283, .F. ) ;
#56932=CARTESIAN_POINT ( 'NONE',  ( 0.000000000000000000, 12.29999999999998295, 0.000000000000000000 ) ) ;
#56937=B_SPLINE_CURVE_WITH_KNOTS ( 'NONE', 3,
 ( #95020, #46265, #175204, #59291, #60354, #161070 ),
 .UNSPECIFIED., .F., .F.,
 ( 4, 2, 4 ),
 ( 0.000000000000000000, 0.0003779448103413555527, 0.0007558896206827111055 ),
 .UNSPECIFIED. ) ;
#56995=VECTOR ( 'NONE', #201680, 1000.000000000000000 ) ;
#57002=DIRECTION ( 'NONE',  ( -0.000000000000000000, 1.000000000000000000, -0.000000000000000000 ) ) ;
#57003=EDGE_CURVE ( 'NONE', #19657, #97605, #10706, .T. ) ;
#57009=CARTESIAN_POINT ( 'NONE',  ( -10.01587959479698320, 5.734125918284786572, -5.906598880481439551 ) ) ;
#57012=EDGE_CURVE ( 'NONE', #75921, #58680, #77718, .T. ) ;
#57014=AXIS2_PLACEMENT_3D ( 'NONE', #4278, #70348, #136465 ) ;
#57034=CARTESIAN_POINT ( 'NONE',  ( 11.92619526913699879, 12.69999999999998153, 1.328859060402684644 ) ) ;
#57047=ADVANCED_FACE ( 'NONE', ( #116945 ), #45372, .T. ) ;
#57086=CARTESIAN_POINT ( 'NONE',  ( -9.429315115559251836, 5.003428342543706719, -6.892195246777336415 ) ) ;
#57110=FILL_AREA_STYLE ('',( #153548 ) ) ;
#57116=EDGE_CURVE ( 'NONE', #123335, #186645, #211251, .T. ) ;
#57149=CARTESIAN_POINT ( 'NONE',  ( 8.868539443929959631, 12.79154120890452440, 8.085006497731432873 ) ) ;
#57167=SURFACE_SIDE_STYLE ('',( #21429 ) ) ;
#57169=ORIENTED_EDGE ( 'NONE', *, *, #75599, .F. ) ;
#57177=( NAMED_UNIT ( * ) PLANE_ANGLE_UNIT ( ) SI_UNIT ( $, .RADIAN. ) );
#57205=SURFACE_STYLE_USAGE ( .BOTH. , #56136 ) ;
#57215=PLANE ( 'NONE',  #44401 ) ;
#57218=VECTOR ( 'NONE', #160975, 1000.000000000000000 ) ;
#57224=FILL_AREA_STYLE ('',( #8456 ) ) ;
#57227=DIRECTION ( 'NONE',  ( 1.000000000000000000, -0.000000000000000000, -0.000000000000000000 ) ) ;
#57232=CARTESIAN_POINT ( 'NONE',  ( -11.33772463945037146, 12.69999999999998153, 3.599999999999999201 ) ) ;
#57235=B_SPLINE_CURVE_WITH_KNOTS ( 'NONE', 3,
 ( #57284, #204568, #107159, #88730, #172106, #74600, #23699 ),
 .UNSPECIFIED., .F., .F.,
 ( 4, 3, 4 ),
 ( 0.000000000000000000, 3.303441823992926441E-05, 4.225144977697881029E-05 ),
 .UNSPECIFIED. ) ;
#57258=FILL_AREA_STYLE ('',( #24739 ) ) ;
#57269=CARTESIAN_POINT ( 'NONE',  ( 11.84668730067608244, 10.19999999999999929, -1.320000000000001616 ) ) ;
#57284=CARTESIAN_POINT ( 'NONE',  ( 1.734723475976807094E-15, 14.57349900225068495, 11.91973154060107376 ) ) ;
#57285=CARTESIAN_POINT ( 'NONE',  ( -10.82994025801865590, 5.589394046361075397, 6.507174183487985708 ) ) ;
#57321=PRESENTATION_STYLE_ASSIGNMENT (( #120263 ) ) ;
#57324=CARTESIAN_POINT ( 'NONE',  ( 11.97929049433705373, 11.37999999999999901, -0.7046979865771834106 ) ) ;
#57331=CARTESIAN_POINT ( 'NONE',  ( 9.367496997597598352, 3.481540744127370690, 7.500000000000000000 ) ) ;
#57337=CARTESIAN_POINT ( 'NONE',  ( -7.788094311009213122, 14.55185938206740026, 9.081607124763383609 ) ) ;
#57344=FACE_OUTER_BOUND ( 'NONE', #39448, .T. ) ;
#57364=PLANE ( 'NONE',  #18266 ) ;
#57392=CARTESIAN_POINT ( 'NONE',  ( 11.75674451658838393, 7.888068978623318017, 2.183490823870577024 ) ) ;
#57416=( LENGTH_UNIT ( ) NAMED_UNIT ( * ) SI_UNIT ( .MILLI., .METRE. ) );
#57425=CARTESIAN_POINT ( 'NONE',  ( -0.05083690440159556456, 15.48930801145573533, 11.99422659986762163 ) ) ;
#57426=CARTESIAN_POINT ( 'NONE',  ( -10.81685113641997020, 3.157239479008171035, 6.648618798508739935 ) ) ;
#57427=ORIENTED_EDGE ( 'NONE', *, *, #172633, .F. ) ;
#57444=FACE_OUTER_BOUND ( 'NONE', #120630, .T. ) ;
#57459=CARTESIAN_POINT ( 'NONE',  ( 0.000000000000000000, 18.91999999999999815, -12.00000000000000178 ) ) ;
#57473=EDGE_CURVE ( 'NONE', #51181, #197365, #117940, .T. ) ;
#57481=CARTESIAN_POINT ( 'NONE',  ( -7.058728332971268671, 14.55191201140709012, 9.659722983215184300 ) ) ;
#57485=DIRECTION ( 'NONE',  ( 0.000000000000000000, 1.000000000000000000, 0.000000000000000000 ) ) ;
#57497=AXIS2_PLACEMENT_3D ( 'NONE', #7704, #42386, #23957 ) ;
#57518=ORIENTED_EDGE ( 'NONE', *, *, #158806, .F. ) ;
#57540=EDGE_CURVE ( 'NONE', #106229, #169055, #155798, .T. ) ;
#57567=CARTESIAN_POINT ( 'NONE',  ( -11.50450067106337571, 6.429220943216678030, -3.050492100467481205 ) ) ;
#57569=CARTESIAN_POINT ( 'NONE',  ( 9.598595877357185557, 13.73909624707286703, 8.266025096903813818 ) ) ;
#57578=EDGE_CURVE ( 'NONE', #157346, #37534, #93783, .T. ) ;
#57581=CARTESIAN_POINT ( 'NONE',  ( 11.86145017031048177, 12.59418046486144327, 1.099999999999996980 ) ) ;
#57585=MECHANICAL_DESIGN_GEOMETRIC_PRESENTATION_REPRESENTATION('',(#71310),#85233);
#57591=CARTESIAN_POINT ( 'NONE',  ( 1.250000000000037526, 8.500000000000000000, -11.02939254900286592 ) ) ;
#57596=LINE ( 'NONE', #172418, #68384 ) ;
#57608=ADVANCED_FACE ( 'NONE', ( #28994 ), #202284, .T. ) ;
#57621=( NAMED_UNIT ( * ) SI_UNIT ( $, .STERADIAN. ) SOLID_ANGLE_UNIT ( ) );
#57633=CARTESIAN_POINT ( 'NONE',  ( -11.86145016429273014, 10.90000000000000036, -1.100000000000002087 ) ) ;
#57655=PLANE ( 'NONE',  #29019 ) ;
#57679=EDGE_CURVE ( 'NONE', #93554, #103541, #109252, .T. ) ;
#57680=FACE_OUTER_BOUND ( 'NONE', #190607, .T. ) ;
#57689=VERTEX_POINT ( 'NONE', #178451 ) ;
#57719=EDGE_CURVE ( 'NONE', #58569, #30509, #88084, .T. ) ;
#57723=CARTESIAN_POINT ( 'NONE',  ( -10.12738493804958750, 3.691521601903835936, 6.358798186737252500 ) ) ;
#57729=DIRECTION ( 'NONE',  ( 0.000000000000000000, 0.000000000000000000, 1.000000000000000000 ) ) ;
#57736=CARTESIAN_POINT ( 'NONE',  ( -10.50660484223216606, 5.359830900411396648, 5.105327592218940502 ) ) ;
#57741=CARTESIAN_POINT ( 'NONE',  ( -11.86145016429273014, 10.19999999999999929, -1.100000000000000311 ) ) ;
#57744=DIRECTION ( 'NONE',  ( 0.000000000000000000, 0.000000000000000000, -1.000000000000000000 ) ) ;
#57784=CARTESIAN_POINT ( 'NONE',  ( -11.94980361058168938, 12.70000000000000107, 1.099999999999996980 ) ) ;
#57799=ORIENTED_EDGE ( 'NONE', *, *, #212293, .F. ) ;
#57801=SURFACE_SIDE_STYLE ('',( #24208 ) ) ;
#57809=CARTESIAN_POINT ( 'NONE',  ( -11.52483635780546578, 13.87999991357544438, 3.345866325258015639 ) ) ;
#57819=CARTESIAN_POINT ( 'NONE',  ( 9.243398672612485711, 11.59071330704323799, 7.171203578799023148 ) ) ;
#57822=ORIENTED_EDGE ( 'NONE', *, *, #81935, .T. ) ;
#57823=CARTESIAN_POINT ( 'NONE',  ( -4.797639995575725180, 14.48151998940196883, -11.00824919010792158 ) ) ;
#57827=ORIENTED_EDGE ( 'NONE', *, *, #179751, .F. ) ;
#57830=B_SPLINE_CURVE_WITH_KNOTS ( 'NONE', 3,
 ( #19710, #6649, #186477, #168111, #90073, #187546 ),
 .UNSPECIFIED., .F., .F.,
 ( 4, 2, 4 ),
 ( 0.0006305064395556248327, 0.0009448735008584364763, 0.001259240562161248120 ),
 .UNSPECIFIED. ) ;
#57844=SURFACE_STYLE_FILL_AREA ( #206218 ) ;
#57852=EDGE_CURVE ( 'NONE', #84082, #14287, #59116, .T. ) ;
#57871=TRIMMED_CURVE ( 'NONE', #135053, ( PARAMETER_VALUE ( 2.526112944919405301 ), #24326 ), ( PARAMETER_VALUE ( 3.141592653589793116 ), #55779 ), .T., .PARAMETER. ) ;
#57892=ORIENTED_EDGE ( 'NONE', *, *, #181856, .F. ) ;
#57907=B_SPLINE_CURVE_WITH_KNOTS ( 'NONE', 3,
 ( #42459, #95485, #94410, #109646, #210247, #43524 ),
 .UNSPECIFIED., .F., .F.,
 ( 4, 2, 4 ),
 ( 0.000000000000000000, 0.0003845013059668464604, 0.0007690026119336929207 ),
 .UNSPECIFIED. ) ;
#57917=CARTESIAN_POINT ( 'NONE',  ( 11.88221712267702834, 7.173824839832926514, 1.903813004346444515 ) ) ;
#57924=CARTESIAN_POINT ( 'NONE',  ( 9.887462820343554171, 14.58581677083729566, 7.687850877847926867 ) ) ;
#57957=CARTESIAN_POINT ( 'NONE',  ( -11.82196040793749425, 4.889518425415825931, 4.884593937341564107 ) ) ;
#57966=ORIENTED_EDGE ( 'NONE', *, *, #103791, .T. ) ;
#57967=STYLED_ITEM ( 'NONE', ( #176501 ), #146923 ) ;
#57986=CARTESIAN_POINT ( 'NONE',  ( 9.904948225507595794, 11.51217390914785099, 6.696207100445890070 ) ) ;
#57996=CARTESIAN_POINT ( 'NONE',  ( 9.428250952287722697, 13.54490846161957585, -7.423481931054030092 ) ) ;
#57997=DIRECTION ( 'NONE',  ( 1.000000000000000000, -0.000000000000000000, 1.224646799147353207E-16 ) ) ;
#58013=CARTESIAN_POINT ( 'NONE',  ( 11.04984958223792368, 9.990824862318733679, 1.056557932048283188 ) ) ;
#58033=DIRECTION ( 'NONE',  ( 1.224646799147343346E-16, 0.000000000000000000, 1.000000000000000000 ) ) ;
#58036=CARTESIAN_POINT ( 'NONE',  ( -10.89183506715999883, 4.909321371462038286, 5.036854565707436393 ) ) ;
#58050=EDGE_LOOP ( 'NONE', ( #77209, #145686, #206456, #3934 ) ) ;
#58057=ORIENTED_EDGE ( 'NONE', *, *, #100659, .F. ) ;
#58073=EDGE_CURVE ( 'NONE', #174805, #85120, #109407, .T. ) ;
#58075=CARTESIAN_POINT ( 'NONE',  ( -10.78552488895401318, 8.017604977416297629, -4.042330561003328881 ) ) ;
#58080=SURFACE_SIDE_STYLE ('',( #43986 ) ) ;
#58112=EDGE_CURVE ( 'NONE', #49891, #143955, #25910, .T. ) ;
#58118=FILL_AREA_STYLE ('',( #74374 ) ) ;
#58128=ORIENTED_EDGE ( 'NONE', *, *, #89674, .T. ) ;
#58145=AXIS2_PLACEMENT_3D ( 'NONE', #136340, #168820, #185052 ) ;
#58152=CARTESIAN_POINT ( 'NONE',  ( -10.40894566972866286, 4.029202461753065734, -7.241727701387177696 ) ) ;
#58205=ORIENTED_EDGE ( 'NONE', *, *, #64968, .F. ) ;
#58206=CIRCLE ( 'NONE', #99797, 0.08000000000000027922 ) ;
#58213=B_SPLINE_CURVE_WITH_KNOTS ( 'NONE', 3,
 ( #194715, #78825, #128741, #743, #96183, #114607 ),
 .UNSPECIFIED., .F., .F.,
 ( 4, 2, 4 ),
 ( 0.000000000000000000, 0.0003767011250903910184, 0.0007534022501807818200 ),
 .UNSPECIFIED. ) ;
#58224=DIRECTION ( 'NONE',  ( 0.000000000000000000, -1.000000000000000000, -9.023263958591317418E-17 ) ) ;
#58229=EDGE_CURVE ( 'NONE', #90728, #140333, #197488, .T. ) ;
#58230=ORIENTED_EDGE ( 'NONE', *, *, #9224, .T. ) ;
#58232=CARTESIAN_POINT ( 'NONE',  ( 11.88172094500853859, 9.720000056015921430, 1.685553348215818925 ) ) ;
#58258=CARTESIAN_POINT ( 'NONE',  ( -9.434499674138207226, 14.57978396016029699, -7.415633383874704165 ) ) ;
#58267=VECTOR ( 'NONE', #22094, 1000.000000000000000 ) ;
#58268=CARTESIAN_POINT ( 'NONE',  ( -10.50000000000000000, 13.39999999999998259, 3.599999999999999201 ) ) ;
#58270=CARTESIAN_POINT ( 'NONE',  ( 8.276983181174589532, 15.22877027432517494, -8.690223756940865130 ) ) ;
#58273=EDGE_CURVE ( 'NONE', #7968, #117790, #34980, .T. ) ;
#58314=ORIENTED_EDGE ( 'NONE', *, *, #140577, .F. ) ;
#58317=ORIENTED_EDGE ( 'NONE', *, *, #128138, .F. ) ;
#58332=DIRECTION ( 'NONE',  ( 0.000000000000000000, 0.000000000000000000, -1.000000000000000000 ) ) ;
#58344=ORIENTED_EDGE ( 'NONE', *, *, #10029, .F. ) ;
#58346=CARTESIAN_POINT ( 'NONE',  ( 10.95308175811721085, 9.799999999999998934, -1.800000000000001155 ) ) ;
#58347=CARTESIAN_POINT ( 'NONE',  ( -11.96212011828584210, 13.82812445049947669, 0.9569185076417884295 ) ) ;
#58348=CARTESIAN_POINT ( 'NONE',  ( -11.75337143377970328, 4.618255228540592228, 5.022398747751031678 ) ) ;
#58359=EDGE_CURVE ( 'NONE', #201490, #108500, #114547, .T. ) ;
#58377=CARTESIAN_POINT ( 'NONE',  ( -9.367496996292747014, 15.51845925588232333, -7.500000001629758550 ) ) ;
#58390=DIRECTION ( 'NONE',  ( 0.000000000000000000, 7.254698431490414842E-17, -1.000000000000000000 ) ) ;
#58391=SURFACE_STYLE_USAGE ( .BOTH. , #155897 ) ;
#58410=CARTESIAN_POINT ( 'NONE',  ( 9.574107565776355244, 3.767509419443892504, 7.159700408882949674 ) ) ;
#58411=CARTESIAN_POINT ( 'NONE',  ( -9.748756651491515157, 4.000000000000000888, 7.301653494243616649 ) ) ;
#58416=FILL_AREA_STYLE_COLOUR ( '', #156596 ) ;
#58428=CARTESIAN_POINT ( 'NONE',  ( 11.86145016429273191, 10.90000000000000036, 1.099999999999996758 ) ) ;
#58430=PRESENTATION_STYLE_ASSIGNMENT (( #140783 ) ) ;
#58447=CARTESIAN_POINT ( 'NONE',  ( -3.069676183974461292, 15.51994954726069409, 11.60951955297166016 ) ) ;
#58449=CARTESIAN_POINT ( 'NONE',  ( -11.88168329227126563, 9.720000000000000639, -1.685799833707129380 ) ) ;
#58457=ORIENTED_EDGE ( 'NONE', *, *, #97488, .T. ) ;
#58462=AXIS2_PLACEMENT_3D ( 'NONE', #156931, #205647, #204569 ) ;
#58463=CARTESIAN_POINT ( 'NONE',  ( 9.422972378981830488, 13.09454993570456161, 7.356553532920802496 ) ) ;
#58492=CARTESIAN_POINT ( 'NONE',  ( -0.08053691275167716712, 15.51887838114830132, 11.99972973886013961 ) ) ;
#58502=ORIENTED_EDGE ( 'NONE', *, *, #183135, .T. ) ;
#58529=LINE ( 'NONE', #27083, #81575 ) ;
#58541=FACE_OUTER_BOUND ( 'NONE', #135395, .T. ) ;
#58550=CARTESIAN_POINT ( 'NONE',  ( 0.000000000000000000, 0.000000000000000000, 0.000000000000000000 ) ) ;
#58555=AXIS2_PLACEMENT_3D ( 'NONE', #93464, #180029, #18569 ) ;
#58569=VERTEX_POINT ( 'NONE', #30217 ) ;
#58586=FACE_OUTER_BOUND ( 'NONE', #172887, .T. ) ;
#58609=( NAMED_UNIT ( * ) SI_UNIT ( $, .STERADIAN. ) SOLID_ANGLE_UNIT ( ) );
#58610=CARTESIAN_POINT ( 'NONE',  ( -11.80247861663003484, 9.799999999999998934, -1.695431928471868188 ) ) ;
#58612=CARTESIAN_POINT ( 'NONE',  ( -11.91826849282518452, 13.39999999999999858, -1.400000000000001465 ) ) ;
#58620=TOROIDAL_SURFACE ( 'NONE', #179681, 11.92000000000000171, 0.08000000000000000167 ) ;
#58638=CARTESIAN_POINT ( 'NONE',  ( -11.86687215968023601, 9.990577876942106528, -1.056395335932043045 ) ) ;
#58678=FACE_OUTER_BOUND ( 'NONE', #86612, .T. ) ;
#58680=VERTEX_POINT ( 'NONE', #118100 ) ;
#58725=( NAMED_UNIT ( * ) SI_UNIT ( $, .STERADIAN. ) SOLID_ANGLE_UNIT ( ) );
#58740=ORIENTED_EDGE ( 'NONE', *, *, #183211, .T. ) ;
#58756=CARTESIAN_POINT ( 'NONE',  ( 0.3554123170485448124, 15.00000000000058265, -12.67999999502907471 ) ) ;
#58791=CARTESIAN_POINT ( 'NONE',  ( 11.41381675112453387, 10.89999999999998259, 3.704697986577180302 ) ) ;
#58804=CARTESIAN_POINT ( 'NONE',  ( -1.538741480077424601E-10, 14.53091781611522748, -12.00000000000003375 ) ) ;
#58818=CARTESIAN_POINT ( 'NONE',  ( -11.41381675112453387, 19.00000000000000000, -3.704697986577182522 ) ) ;
#58864=ORIENTED_EDGE ( 'NONE', *, *, #118985, .T. ) ;
#58866=FILL_AREA_STYLE ('',( #43709 ) ) ;
#58870=CARTESIAN_POINT ( 'NONE',  ( 11.63272104808981666, 8.261185799347773084, 2.974823062023182363 ) ) ;
#58873=VECTOR ( 'NONE', #147470, 1000.000000000000000 ) ;
#58877=CARTESIAN_POINT ( 'NONE',  ( -11.48784849554592924, 13.83049527181932348, 3.469614872287846374 ) ) ;
#58880=B_SPLINE_CURVE_WITH_KNOTS ( 'NONE', 3,
 ( #169041, #17435, #151745, #70448, #120374, #83519, #52101 ),
 .UNSPECIFIED., .F., .F.,
 ( 4, 3, 4 ),
 ( -0.0002318125648490880985, 0.000000000000000000, 0.0004044109710639508877 ),
 .UNSPECIFIED. ) ;
#58892=CARTESIAN_POINT ( 'NONE',  ( 9.941052257571969974, 9.384232882455165736, -7.145601325162150630 ) ) ;
#58899=ORIENTED_EDGE ( 'NONE', *, *, #134279, .F. ) ;
#58908=CARTESIAN_POINT ( 'NONE',  ( 9.476364159883861049, 3.602179703620751905, -7.289721612074726131 ) ) ;
#58918=LINE ( 'NONE', #92520, #113492 ) ;
#58946=CARTESIAN_POINT ( 'NONE',  ( 0.3263184169964571946, 14.00000000000058265, 11.67999999558625213 ) ) ;
#58964=ORIENTED_EDGE ( 'NONE', *, *, #200653, .F. ) ;
#58987=CARTESIAN_POINT ( 'NONE',  ( 9.086253353280454803, 13.39999999999999680, -7.838367176906162470 ) ) ;
#58994=CARTESIAN_POINT ( 'NONE',  ( 8.518320732998095224, 14.76619040281040718, 9.398253358897362020 ) ) ;
#59024=CARTESIAN_POINT ( 'NONE',  ( -11.31901822352654641, 5.215070234333009758, -5.710337001866061968 ) ) ;
#59048=CARTESIAN_POINT ( 'NONE',  ( 10.80502615499130314, 9.582201645171684490, 5.117034356647724991 ) ) ;
#59096=PRESENTATION_STYLE_ASSIGNMENT (( #92694 ) ) ;
#59113=CIRCLE ( 'NONE', #207836, 11.09999999999999964 ) ;
#59116=CIRCLE ( 'NONE', #124924, 0.08000000000000040412 ) ;
#59129=FILL_AREA_STYLE_COLOUR ( '', #37434 ) ;
#59134=EDGE_CURVE ( 'NONE', #83956, #75921, #139638, .T. ) ;
#59138=CARTESIAN_POINT ( 'NONE',  ( -9.997759874121660673, 5.662387697485826266, 5.943071269081472430 ) ) ;
#59165=ORIENTED_EDGE ( 'NONE', *, *, #135967, .F. ) ;
#59182=PRODUCT ( 'chamber', 'chamber', '', ( #102406 ) ) ;
#59183=EDGE_CURVE ( 'NONE', #140668, #131565, #103413, .T. ) ;
#59203=FILL_AREA_STYLE ('',( #122169 ) ) ;
#59208=CARTESIAN_POINT ( 'NONE',  ( -10.20559888102932256, 5.000029895416906456, -7.525687786258633771 ) ) ;
#59241=B_SPLINE_CURVE_WITH_KNOTS ( 'NONE', 3,
 ( #30142, #64764, #147108, #113593, #144997, #179596, #31217, #114656, #130906, #196898 ),
 .UNSPECIFIED., .F., .F.,
 ( 4, 2, 2, 2, 4 ),
 ( 7.239403734744659911E-05, 0.0003307887970069321769, 0.0005891835566664177818, 0.0008475783163259033868, 0.001105973075985389100 ),
 .UNSPECIFIED. ) ;
#59260=EDGE_CURVE ( 'NONE', #86738, #159273, #114387, .T. ) ;
#59264=AXIS2_PLACEMENT_3D ( 'NONE', #145111, #128901, #194882 ) ;
#59270=MECHANICAL_DESIGN_GEOMETRIC_PRESENTATION_REPRESENTATION('',(#118249),#183877);
#59288=CARTESIAN_POINT ( 'NONE',  ( 11.41381675112453387, 12.69999999999999929, -3.704697986577184299 ) ) ;
#59291=CARTESIAN_POINT ( 'NONE',  ( -11.92045683181315674, 12.44724072120513547, 1.382340670101856350 ) ) ;
#59311=CARTESIAN_POINT ( 'NONE',  ( 11.71312635250765055, 6.993950423356553259, 2.415994165151631901 ) ) ;
#59320=CARTESIAN_POINT ( 'NONE',  ( -6.024157315724540496, 15.51887179519442306, 10.38786933647550192 ) ) ;
#59331=CARTESIAN_POINT ( 'NONE',  ( -11.86239285000045918, 11.37999999999999901, -1.812080536912752837 ) ) ;
#59343=CARTESIAN_POINT ( 'NONE',  ( 0.000000000000000000, 4.446955548196733332, 0.000000000000000000 ) ) ;
#59404=EDGE_LOOP ( 'NONE', ( #2649, #18087, #42529, #37923 ) ) ;
#59407=CARTESIAN_POINT ( 'NONE',  ( 9.692997807120237397, 13.38204337665774624, -8.150562841249751500 ) ) ;
#59408=CARTESIAN_POINT ( 'NONE',  ( -10.68898853036274055, 3.992937990999307907, 4.901699750972148273 ) ) ;
#59414=CARTESIAN_POINT ( 'NONE',  ( -11.88156762547253997, 11.37999991545968115, -1.686557021358706221 ) ) ;
#59437=EDGE_CURVE ( 'NONE', #24390, #70986, #206597, .T. ) ;
#59457=CARTESIAN_POINT ( 'NONE',  ( -11.86145016429273191, 13.40000000000000036, -1.180000000000002158 ) ) ;
#59467=CARTESIAN_POINT ( 'NONE',  ( 9.333041836227126353, 3.553052365627043407, 7.472413793103448221 ) ) ;
#59472=FILL_AREA_STYLE ('',( #58416 ) ) ;
#59476=CARTESIAN_POINT ( 'NONE',  ( -10.14265820453532818, 3.662953273883144512, 6.345113228764306612 ) ) ;
#59479=VERTEX_POINT ( 'NONE', #50377 ) ;
#59503=DIRECTION ( 'NONE',  ( -0.000000000000000000, -1.000000000000000000, -0.000000000000000000 ) ) ;
#59511=EDGE_LOOP ( 'NONE', ( #17340, #139094, #212369, #50372 ) ) ;
#59539=FILL_AREA_STYLE_COLOUR ( '', #143530 ) ;
#59542=EDGE_CURVE ( 'NONE', #61441, #30537, #113447, .T. ) ;
#59545=( BOUNDED_SURFACE ( )  B_SPLINE_SURFACE ( 3, 2, ( 
 ( #209538, #127340, #15605 ),
 ( #129475, #32948, #146730 ),
 ( #94772, #212748, #64382 ),
 ( #130527, #213792, #196518 ),
 ( #31894, #114273, #47086 ),
 ( #131564, #180270, #111064 ),
 ( #197565, #62250, #115329 ),
 ( #181320, #99022, #193310 ),
 ( #177070, #28686, #112140 ),
 ( #160820, #12412, #78492 ),
 ( #144609, #210624, #128411 ),
 ( #194378, #29758, #95843 ),
 ( #133682, #135787, #38277 ),
 ( #149906, #152035, #148827 ),
 ( #34002, #153095, #100076 ),
 ( #83813, #116384, #68614 ),
 ( #132612, #3606, #85960 ),
 ( #87023, #170399, #136856 ) ),
 .UNSPECIFIED., .F., .F., .F. ) 
 B_SPLINE_SURFACE_WITH_KNOTS ( ( 4, 2, 2, 2, 2, 2, 2, 2, 4 ),
 ( 3, 3 ),
 ( 0.000000000000000000, 8.835779872240032032E-05, 0.0001767155974448006406, 0.0003534311948896012813, 0.0007068623897792025625, 0.001060293584668803735, 0.001237009182113604430, 0.001325366980836004778, 0.001413724779558405125 ),
 ( 0.000000000000000000, 1.000000000000000000 ),
 .UNSPECIFIED. ) 
 GEOMETRIC_REPRESENTATION_ITEM ( )  RATIONAL_B_SPLINE_SURFACE ( (
 ( 1.000000000000000000, 0.8509629433930272491, 1.000000000000000000),
 ( 1.000000000000000000, 0.8498006689636994349, 1.000000000000000000),
 ( 1.000000000000000000, 0.8320552335758597540, 1.000000000000000000),
 ( 1.000000000000000000, 0.8099185496503389370, 1.000000000000000000),
 ( 1.000000000000000000, 0.8026556248207100674, 1.000000000000000000),
 ( 1.000000000000000000, 0.7864057361306107108, 1.000000000000000000),
 ( 1.000000000000000000, 0.7820376696873353461, 1.000000000000000000),
 ( 1.000000000000000000, 0.7712304172370865185, 1.000000000000000000),
 ( 1.000000000000000000, 0.7693781127550674004, 1.000000000000000000),
 ( 1.000000000000000000, 0.7693828318334674510, 1.000000000000000000),
 ( 1.000000000000000000, 0.7713025106554596277, 1.000000000000000000),
 ( 1.000000000000000000, 0.7820120509638822659, 1.000000000000000000),
 ( 1.000000000000000000, 0.7865355379946432635, 1.000000000000000000),
 ( 1.000000000000000000, 0.8025478250466264729, 1.000000000000000000),
 ( 1.000000000000000000, 0.8098425558904723820, 1.000000000000000000),
 ( 1.000000000000000000, 0.8320142513982312638, 1.000000000000000000),
 ( 1.000000000000000000, 0.8496692043554369134, 1.000000000000000000),
 ( 1.000000000000000000, 0.8509629433917196284, 1.000000000000000000) ) ) 
 REPRESENTATION_ITEM ( '' )  SURFACE ( )  );
#59570=VERTEX_POINT ( 'NONE', #187827 ) ;
#59602=CARTESIAN_POINT ( 'NONE',  ( -4.288887917185465248, 14.55258240538958425, 11.16905078721341837 ) ) ;
#59638=DIRECTION ( 'NONE',  ( 0.000000000000000000, 0.000000000000000000, -1.000000000000000000 ) ) ;
#59649=CARTESIAN_POINT ( 'NONE',  ( 11.48243876534946217, 11.37999999999999901, -3.200000000000001510 ) ) ;
#59654=SURFACE_STYLE_FILL_AREA ( #104153 ) ;
#59666=EDGE_LOOP ( 'NONE', ( #171321, #54544, #72722, #110004 ) ) ;
#59669=CARTESIAN_POINT ( 'NONE',  ( 11.01135777277262306, 12.59375064782103948, 1.399999999999998357 ) ) ;
#59671=CARTESIAN_POINT ( 'NONE',  ( 11.48767021851168124, 9.769957725361692269, -3.470194894594655910 ) ) ;
#59686=DIRECTION ( 'NONE',  ( 0.000000000000000000, 1.000000000000000000, 0.000000000000000000 ) ) ;
#59695=ADVANCED_FACE ( 'NONE', ( #122941 ), #121856, .T. ) ;
#59721=LINE ( 'NONE', #189716, #9641 ) ;
#59729=AXIS2_PLACEMENT_3D ( 'NONE', #198660, #130570, #48202 ) ;
#59739=CARTESIAN_POINT ( 'NONE',  ( 7.308564027072312008, 14.53708027256903712, 9.465002577604847644 ) ) ;
#59741=ORIENTED_EDGE ( 'NONE', *, *, #144973, .T. ) ;
#59764=AXIS2_PLACEMENT_3D ( 'NONE', #166529, #136180, #135120 ) ;
#59780=( NAMED_UNIT ( * ) SI_UNIT ( $, .STERADIAN. ) SOLID_ANGLE_UNIT ( ) );
#59788=CARTESIAN_POINT ( 'NONE',  ( 11.01135777277262306, 10.19999999999999929, -1.400000000000001910 ) ) ;
#59790=CIRCLE ( 'NONE', #70113, 0.5000000000000022204 ) ;
#59794=ORIENTED_EDGE ( 'NONE', *, *, #79457, .F. ) ;
#59801=CARTESIAN_POINT ( 'NONE',  ( 8.230252249265882725, 15.15998367271711622, 8.673456544423645553 ) ) ;
#59805=FILL_AREA_STYLE ('',( #91267 ) ) ;
#59807=CIRCLE ( 'NONE', #198315, 11.09999999999999964 ) ;
#59816=UNCERTAINTY_MEASURE_WITH_UNIT (LENGTH_MEASURE( 1.000000000000000082E-05 ), #155137, 'distance_accuracy_value', 'NONE');
#59827=EDGE_LOOP ( 'NONE', ( #183848, #92999, #36762, #117836, #179058, #23243, #32799, #202169 ) ) ;
#59882=LINE ( 'NONE', #58818, #14563 ) ;
#59912=CARTESIAN_POINT ( 'NONE',  ( -11.97178994924802353, 12.22000006202794609, 0.8322011300497199615 ) ) ;
#59920=STYLED_ITEM ( 'NONE', ( #170797 ), #30374 ) ;
#59922=CARTESIAN_POINT ( 'NONE',  ( -11.52469724861193967, 11.37999993351231254, -3.346365485506884063 ) ) ;
#59926=CARTESIAN_POINT ( 'NONE',  ( -11.52463353791760348, 12.21999999999998110, 3.346594096177640143 ) ) ;
#59933=CARTESIAN_POINT ( 'NONE',  ( 9.428250952287722697, 13.54490846161957585, -7.423481931054030092 ) ) ;
#59951=AXIS2_PLACEMENT_3D ( 'NONE', #39590, #72065, #105694 ) ;
#59952=CARTESIAN_POINT ( 'NONE',  ( 8.358788729863725564, 13.10643031998909258, -8.536585299322529963 ) ) ;
#59960=ORIENTED_EDGE ( 'NONE', *, *, #84325, .F. ) ;
#59968=DIRECTION ( 'NONE',  ( 0.000000000000000000, -1.000000000000000000, 0.000000000000000000 ) ) ;
#59990=EDGE_CURVE ( 'NONE', #152119, #127188, #211563, .T. ) ;
#60012=CARTESIAN_POINT ( 'NONE',  ( -6.671583288098690723, 14.00000000000246381, 9.747470831330483421 ) ) ;
#60024=( GEOMETRIC_REPRESENTATION_CONTEXT ( 3 ) GLOBAL_UNCERTAINTY_ASSIGNED_CONTEXT ( ( #123041 ) ) GLOBAL_UNIT_ASSIGNED_CONTEXT ( ( #21195, #88372, #184777 ) ) REPRESENTATION_CONTEXT ( 'NONE', 'WORKASPACE' ) );
#60041=FILL_AREA_STYLE_COLOUR ( '', #19622 ) ;
#60052=CARTESIAN_POINT ( 'NONE',  ( -10.71870444596734195, 5.124999999999999112, 5.395310463726811001 ) ) ;
#60059=CARTESIAN_POINT ( 'NONE',  ( 10.00008462853139690, 14.27679787173769910, 7.523198333661912152 ) ) ;
#60089=CARTESIAN_POINT ( 'NONE',  ( -11.68462027884434917, 8.171766027648200037, -4.455682980299036089 ) ) ;
#60091=AXIS2_PLACEMENT_3D ( 'NONE', #198380, #18571, #86784 ) ;
#60095=MECHANICAL_DESIGN_GEOMETRIC_PRESENTATION_REPRESENTATION('',(#91194),#49729);
#60097=AXIS2_PLACEMENT_3D ( 'NONE', #36074, #186597, #134688 ) ;
#60105=FILL_AREA_STYLE_COLOUR ( '', #118455 ) ;
#60111=ORIENTED_EDGE ( 'NONE', *, *, #187238, .T. ) ;
#60117=CARTESIAN_POINT ( 'NONE',  ( 11.15024502828561559, 9.129283359492950112, 4.439156027159579132 ) ) ;
#60132=EDGE_CURVE ( 'NONE', #163314, #135251, #144497, .T. ) ;
#60154=EDGE_CURVE ( 'NONE', #149077, #4563, #149245, .T. ) ;
#60180=ORIENTED_EDGE ( 'NONE', *, *, #23157, .F. ) ;
#60194=B_SPLINE_CURVE_WITH_KNOTS ( 'NONE', 3,
 ( #45978, #178102, #112099, #29718, #95800, #161856 ),
 .UNSPECIFIED., .F., .F.,
 ( 4, 2, 4 ),
 ( 0.000000000000000000, 0.0003239988925529259205, 0.0006479977851058518409 ),
 .UNSPECIFIED. ) ;
#60202=CARTESIAN_POINT ( 'NONE',  ( -10.99298880388840338, 6.209297407268072888, -6.173882299569079635 ) ) ;
#60205=ORIENTED_EDGE ( 'NONE', *, *, #197807, .F. ) ;
#60207=PLANE ( 'NONE',  #21397 ) ;
#60230=ORIENTED_EDGE ( 'NONE', *, *, #12290, .T. ) ;
#60232=CARTESIAN_POINT ( 'NONE',  ( -15.75000000000000000, 13.39999999999998259, 1.399999999999998579 ) ) ;
#60243=STYLED_ITEM ( 'NONE', ( #59096 ), #185241 ) ;
#60244=PRESENTATION_STYLE_ASSIGNMENT (( #9365 ) ) ;
#60272=CARTESIAN_POINT ( 'NONE',  ( -11.43209210103587914, 13.65596075983916080, -3.649125173352125273 ) ) ;
#60277=CARTESIAN_POINT ( 'NONE',  ( -10.76260246389097297, 4.190717020667873882, -6.707086991120802644 ) ) ;
#60282=VERTEX_POINT ( 'NONE', #134187 ) ;
#60291=CARTESIAN_POINT ( 'NONE',  ( 0.000000000000000000, 19.00000000000000000, -12.00000000000000178 ) ) ;
#60341=CARTESIAN_POINT ( 'NONE',  ( 11.99988598803232875, 6.571561536565357464, 0.5026004568578228415 ) ) ;
#60354=CARTESIAN_POINT ( 'NONE',  ( -11.92619526913700057, 12.57218333338755123, 1.328859060402684644 ) ) ;
#60357=ORIENTED_EDGE ( 'NONE', *, *, #80161, .T. ) ;
#60376=CARTESIAN_POINT ( 'NONE',  ( -10.29981080141455685, 4.865373709629901455, 6.164441567520336562 ) ) ;
#60383=ORIENTED_EDGE ( 'NONE', *, *, #135546, .F. ) ;
#60392=( NAMED_UNIT ( * ) PLANE_ANGLE_UNIT ( ) SI_UNIT ( $, .RADIAN. ) );
#60415=CARTESIAN_POINT ( 'NONE',  ( 9.218433053458319648, 14.16038166358193884, -7.683070978493945269 ) ) ;
#60416=TOROIDAL_SURFACE ( 'NONE', #25776, 12.18000000000000149, 0.5000000000000008882 ) ;
#60448=CIRCLE ( 'NONE', #5223, 11.95586206896558146 ) ;
#60468=CARTESIAN_POINT ( 'NONE',  ( 10.28744933574984799, 12.75976789843056203, -6.941907919544356709 ) ) ;
#60477=ORIENTED_EDGE ( 'NONE', *, *, #132683, .F. ) ;
#60508=CARTESIAN_POINT ( 'NONE',  ( -10.95308175811721085, 12.30000000000000071, -1.800000000000001155 ) ) ;
#60516=EDGE_CURVE ( 'NONE', #201330, #204988, #167855, .T. ) ;
#60539=CARTESIAN_POINT ( 'NONE',  ( -10.84194200455609725, 4.687741901903320851, 5.144714966584626126 ) ) ;
#60543=ORIENTED_EDGE ( 'NONE', *, *, #94600, .T. ) ;
#60549=CYLINDRICAL_SURFACE ( 'NONE', #23312, 0.07999999999999998779 ) ;
#60551=DIRECTION ( 'NONE',  ( -0.000000000000000000, 0.000000000000000000, -1.000000000000000000 ) ) ;
#60605=AXIS2_PLACEMENT_3D ( 'NONE', #143948, #78883, #145006 ) ;
#60606=DIRECTION ( 'NONE',  ( 0.000000000000000000, 1.000000000000000000, 0.000000000000000000 ) ) ;
#60618=CARTESIAN_POINT ( 'NONE',  ( -9.587704862635016312, 4.026159954882873926, 6.671158199369250141 ) ) ;
#60632=ORIENTED_EDGE ( 'NONE', *, *, #176386, .F. ) ;
#60652=ADVANCED_FACE ( 'NONE', ( #140601 ), #121193, .F. ) ;
#60686=FACE_OUTER_BOUND ( 'NONE', #195532, .T. ) ;
#60716=FACE_OUTER_BOUND ( 'NONE', #178809, .T. ) ;
#60731=CARTESIAN_POINT ( 'NONE',  ( 11.01135777277262306, 12.69999999999998153, 1.399999999999998579 ) ) ;
#60737=ADVANCED_FACE ( 'NONE', ( #114991 ), #45692, .F. ) ;
#60741=ORIENTED_EDGE ( 'NONE', *, *, #123262, .T. ) ;
#60749=ORIENTED_EDGE ( 'NONE', *, *, #83855, .F. ) ;
#60758=CARTESIAN_POINT ( 'NONE',  ( 9.410656278130334229, 14.12788591601509758, 8.484697815724119963 ) ) ;
#60772=EDGE_CURVE ( 'NONE', #4563, #48008, #20518, .T. ) ;
#60773=CARTESIAN_POINT ( 'NONE',  ( 11.86687215968023601, 12.49057787694218824, 1.056395335932121871 ) ) ;
#60778=ORIENTED_EDGE ( 'NONE', *, *, #117565, .F. ) ;
#60789=CARTESIAN_POINT ( 'NONE',  ( -10.50000000000000000, 12.69999999999999929, -3.600000000000000977 ) ) ;
#60799=ADVANCED_FACE ( 'NONE', ( #110737 ), #28351, .F. ) ;
#60805=( LENGTH_UNIT ( ) NAMED_UNIT ( * ) SI_UNIT ( .MILLI., .METRE. ) );
#60810=ORIENTED_EDGE ( 'NONE', *, *, #7913, .T. ) ;
#60814=CARTESIAN_POINT ( 'NONE',  ( -9.766653781993813510, 4.463134066693873692, -6.897859727666959095 ) ) ;
#60834=DIRECTION ( 'NONE',  ( 0.000000000000000000, 0.000000000000000000, -1.000000000000000000 ) ) ;
#60868=UNCERTAINTY_MEASURE_WITH_UNIT (LENGTH_MEASURE( 1.000000000000000082E-05 ), #184179, 'distance_accuracy_value', 'NONE');
#60871=EDGE_CURVE ( 'NONE', #142717, #34845, #87093, .T. ) ;
#60872=DIRECTION ( 'NONE',  ( 0.000000000000000000, 0.000000000000000000, 1.000000000000000000 ) ) ;
#60896=MECHANICAL_DESIGN_GEOMETRIC_PRESENTATION_REPRESENTATION('',(#33216),#19282);
#60927=CARTESIAN_POINT ( 'NONE',  ( 11.33772463945037146, 10.89999999999998259, 3.599999999999999201 ) ) ;
#60934=CARTESIAN_POINT ( 'NONE',  ( -1.499999999999963141, 7.750000000000000000, 10.99818166789402341 ) ) ;
#60939=CARTESIAN_POINT ( 'NONE',  ( 11.33772465723203915, 11.00868300734825667, -3.600000000000076472 ) ) ;
#60976=ORIENTED_EDGE ( 'NONE', *, *, #122928, .F. ) ;
#61000=ORIENTED_EDGE ( 'NONE', *, *, #45759, .T. ) ;
#61005=CARTESIAN_POINT ( 'NONE',  ( 11.95247249465994166, 7.720304541436361134, -1.088600100142860017 ) ) ;
#61012=CARTESIAN_POINT ( 'NONE',  ( 10.50000000000000178, 10.19999999999999929, -3.600000000000000977 ) ) ;
#61024=CARTESIAN_POINT ( 'NONE',  ( 11.74001039742577923, 6.813547096158895755, 0.9622183096568183158 ) ) ;
#61029=EDGE_LOOP ( 'NONE', ( #181679, #7994, #48012, #110704 ) ) ;
#61031=ORIENTED_EDGE ( 'NONE', *, *, #108300, .F. ) ;
#61039=LINE ( 'NONE', #179071, #171447 ) ;
#61040=LINE ( 'NONE', #197165, #27178 ) ;
#61080=CARTESIAN_POINT ( 'NONE',  ( -11.07651133989102554, 5.830166859442025284, -4.512497092989907976 ) ) ;
#61112=PRESENTATION_STYLE_ASSIGNMENT (( #143474 ) ) ;
#61121=CARTESIAN_POINT ( 'NONE',  ( -10.71870444596734195, 5.124999999999999112, 5.395310463726811001 ) ) ;
#61128=CARTESIAN_POINT ( 'NONE',  ( 8.806674072578211110, 13.38234123322611779, 7.683694639725048958 ) ) ;
#61134=ORIENTED_EDGE ( 'NONE', *, *, #161956, .F. ) ;
#61161=CARTESIAN_POINT ( 'NONE',  ( -11.69243366784185945, 8.407932920124673970, 1.097391832464843286 ) ) ;
#61167=MECHANICAL_DESIGN_GEOMETRIC_PRESENTATION_REPRESENTATION('',(#202924),#151150);
#61175=CARTESIAN_POINT ( 'NONE',  ( -15.75000000000000000, 10.90000000000000036, -0.7000000000000009548 ) ) ;
#61181=ORIENTED_EDGE ( 'NONE', *, *, #100659, .T. ) ;
#61188=CARTESIAN_POINT ( 'NONE',  ( 11.97491505176683724, 7.682034517632803983, 0.8879925087013592622 ) ) ;
#61190=EDGE_CURVE ( 'NONE', #106229, #7968, #53121, .T. ) ;
#61220=ADVANCED_FACE ( 'NONE', ( #117119 ), #118191, .F. ) ;
#61226=COLOUR_RGB ( '', 0.09019608, 0.27058824, 0.51372549) ;
#61239=CARTESIAN_POINT ( 'NONE',  ( -10.91033920341459229, 4.885615726745597520, 4.996448585388895580 ) ) ;
#61247=CARTESIAN_POINT ( 'NONE',  ( -10.63109271062926275, 5.887865540153549127, -5.475652048317233955 ) ) ;
#61277=CARTESIAN_POINT ( 'NONE',  ( -11.34338453707543515, 5.310936115193626961, -5.661293933977025183 ) ) ;
#61293=ORIENTED_EDGE ( 'NONE', *, *, #171367, .F. ) ;
#61353=CARTESIAN_POINT ( 'NONE',  ( -9.348596576284975868, 2.999985932080179829, -7.001940380475246251 ) ) ;
#61354=AXIS2_PLACEMENT_3D ( 'NONE', #101677, #167747, #19347 ) ;
#61360=EDGE_LOOP ( 'NONE', ( #175217, #176093, #57799, #153828, #75425, #134572 ) ) ;
#61426=VERTEX_POINT ( 'NONE', #205762 ) ;
#61435=( BOUNDED_SURFACE ( )  B_SPLINE_SURFACE ( 3, 2, ( 
 ( #158286, #78079, #178799 ),
 ( #160403, #144204, #210200 ),
 ( #30415, #159333, #45604 ),
 ( #58638, #111721, #177729 ),
 ( #124791, #190751, #97554 ),
 ( #132201, #49843, #196109 ) ),
 .UNSPECIFIED., .F., .F., .T. ) 
 B_SPLINE_SURFACE_WITH_KNOTS ( ( 4, 2, 4 ),
 ( 3, 3 ),
 ( 0.000000000000000000, 0.0003754689591423961527, 0.0007509379182847923054 ),
 ( 0.000000000000000000, 1.000000000000000000 ),
 .UNSPECIFIED. ) 
 GEOMETRIC_REPRESENTATION_ITEM ( )  RATIONAL_B_SPLINE_SURFACE ( (
 ( 1.000000000000000000, 0.7071067811865475727, 1.000000000000000000),
 ( 1.000000000000000000, 0.7018599272024182989, 1.000000000000000000),
 ( 1.000000000000000000, 0.6927733177260235742, 1.000000000000000000),
 ( 1.000000000000000000, 0.6772007068873748814, 1.000000000000000000),
 ( 1.000000000000000000, 0.6709974581637003777, 1.000000000000000000),
 ( 1.000000000000000000, 0.6711954675835484219, 1.000000000000000000) ) ) 
 REPRESENTATION_ITEM ( '' )  SURFACE ( )  );
#61441=VERTEX_POINT ( 'NONE', #93114 ) ;
#61446=CARTESIAN_POINT ( 'NONE',  ( 10.36569475343129731, 9.168110967066926520, -6.000526395088528808 ) ) ;
#61449=PRESENTATION_STYLE_ASSIGNMENT (( #144880 ) ) ;
#61453=CARTESIAN_POINT ( 'NONE',  ( -7.138471902074302378, 15.51981486752699446, 9.655967197029408311 ) ) ;
#61487=CARTESIAN_POINT ( 'NONE',  ( 8.865490439548599610, 14.65774821460601274, -8.021509641190812445 ) ) ;
#61499=MECHANICAL_DESIGN_GEOMETRIC_PRESENTATION_REPRESENTATION('',(#154890),#40802);
#61508=EDGE_CURVE ( 'NONE', #75373, #210434, #125674, .T. ) ;
#61513=CARTESIAN_POINT ( 'NONE',  ( 0.000000000000000000, 11.37999999999998302, 0.000000000000000000 ) ) ;
#61529=CARTESIAN_POINT ( 'NONE',  ( 8.432907547770344792, 13.95827226627088180, -8.537830883650524783 ) ) ;
#61533=CARTESIAN_POINT ( 'NONE',  ( 11.91292854676725987, 13.61481529673029556, 1.446370920797347415 ) ) ;
#61538=CARTESIAN_POINT ( 'NONE',  ( 10.15942246637696655, 13.50131128642754952, -7.248264454434499626 ) ) ;
#61570=EDGE_CURVE ( 'NONE', #39641, #121817, #116123, .T. ) ;
#61590=LINE ( 'NONE', #193716, #202155 ) ;
#61594=PRESENTATION_STYLE_ASSIGNMENT (( #13890 ) ) ;
#61608=TOROIDAL_SURFACE ( 'NONE', #179297, 11.92000000000000171, 0.08000000000000000167 ) ;
#61646=STYLED_ITEM ( 'NONE', ( #193556 ), #106360 ) ;
#61654=( NAMED_UNIT ( * ) PLANE_ANGLE_UNIT ( ) SI_UNIT ( $, .RADIAN. ) );
#61662=CARTESIAN_POINT ( 'NONE',  ( 11.81905481421901705, 12.34264344382731871, 1.592167362352177262 ) ) ;
#61679=DIRECTION ( 'NONE',  ( -0.000000000000000000, -1.000000000000000000, -0.000000000000000000 ) ) ;
#61680=CARTESIAN_POINT ( 'NONE',  ( 11.84100621633422179, 11.11041574223334649, 1.444132586618105174 ) ) ;
#61687=CARTESIAN_POINT ( 'NONE',  ( 0.008622056077349157799, 14.55305231409391808, 11.95585894185517084 ) ) ;
#61688=EDGE_CURVE ( 'NONE', #154255, #149077, #17815, .T. ) ;
#61742=CARTESIAN_POINT ( 'NONE',  ( -1.673882606082500946, 14.48013547004651436, 11.91749650979550701 ) ) ;
#61759=AXIS2_PLACEMENT_3D ( 'NONE', #59457, #22668, #122428 ) ;
#61764=DIRECTION ( 'NONE',  ( 0.000000000000000000, 0.000000000000000000, -1.000000000000000000 ) ) ;
#61777=CARTESIAN_POINT ( 'NONE',  ( 11.55950211276791428, 12.22000000000000064, -3.221476510067115662 ) ) ;
#61789=VERTEX_POINT ( 'NONE', #177550 ) ;
#61795=CARTESIAN_POINT ( 'NONE',  ( -11.84668730067608600, 10.19999999999998153, 1.399999999999998579 ) ) ;
#61813=CARTESIAN_POINT ( 'NONE',  ( 0.000000000000000000, 11.37999999999999901, 0.000000000000000000 ) ) ;
#61828=CARTESIAN_POINT ( 'NONE',  ( -11.94105721237523099, 13.40000000000000036, 1.187919463087248273 ) ) ;
#61852=CARTESIAN_POINT ( 'NONE',  ( 0.000000000000000000, 4.000007913748540922, 0.000000000000000000 ) ) ;
#61859=DIRECTION ( 'NONE',  ( 0.000000000000000000, 0.000000000000000000, -1.000000000000000000 ) ) ;
#61886=CARTESIAN_POINT ( 'NONE',  ( -10.49167095263963034, 5.343775707538782171, -5.730694126968528757 ) ) ;
#61909=CARTESIAN_POINT ( 'NONE',  ( -11.89197816957260478, 13.79999999999999893, -0.8055420615339585755 ) ) ;
#61914=CIRCLE ( 'NONE', #155301, 0.07999999999999998779 ) ;
#61919=ORIENTED_EDGE ( 'NONE', *, *, #207872, .F. ) ;
#61923=DIRECTION ( 'NONE',  ( 1.000000000000000000, -0.000000000000000000, -0.000000000000000000 ) ) ;
#61955=UNCERTAINTY_MEASURE_WITH_UNIT (LENGTH_MEASURE( 1.000000000000000082E-05 ), #41497, 'distance_accuracy_value', 'NONE');
#61984=VERTEX_POINT ( 'NONE', #212147 ) ;
#61990=ORIENTED_EDGE ( 'NONE', *, *, #168278, .F. ) ;
#62009=CARTESIAN_POINT ( 'NONE',  ( -11.55950211276791428, 13.87999999999998302, 3.221476510067114329 ) ) ;
#62044=( NAMED_UNIT ( * ) PLANE_ANGLE_UNIT ( ) SI_UNIT ( $, .RADIAN. ) );
#62088=( NAMED_UNIT ( * ) PLANE_ANGLE_UNIT ( ) SI_UNIT ( $, .RADIAN. ) );
#62100=CARTESIAN_POINT ( 'NONE',  ( 9.639237905258834616, 11.95699723271644466, -8.657004797785544881 ) ) ;
#62106=VERTEX_POINT ( 'NONE', #202009 ) ;
#62154=CARTESIAN_POINT ( 'NONE',  ( 0.000000000000000000, 0.08000000000000020983, 11.92000000000000171 ) ) ;
#62158=CARTESIAN_POINT ( 'NONE',  ( -1.878313713278110919, 15.99999999999692335, 12.68000002627077905 ) ) ;
#62159=CARTESIAN_POINT ( 'NONE',  ( 0.000000000000000000, 0.08000000000000020983, 0.000000000000000000 ) ) ;
#62179=( NAMED_UNIT ( * ) SI_UNIT ( $, .STERADIAN. ) SOLID_ANGLE_UNIT ( ) );
#62182=EDGE_CURVE ( 'NONE', #54188, #182367, #154375, .T. ) ;
#62187=DIRECTION ( 'NONE',  ( 0.000000000000000000, 0.000000000000000000, -1.000000000000000000 ) ) ;
#62201=CARTESIAN_POINT ( 'NONE',  ( 8.800298414079730236, 13.41797088714002761, -7.691148693810730741 ) ) ;
#62204=CARTESIAN_POINT ( 'NONE',  ( 8.342299507848510487, 13.15171158923614669, 8.537531030106581653 ) ) ;
#62235=CARTESIAN_POINT ( 'NONE',  ( -10.78227258717170578, 6.269840026405313793, 4.500979083849748541 ) ) ;
#62250=CARTESIAN_POINT ( 'NONE',  ( -9.494322903035145700, 14.66521395919849624, 7.339005329529387112 ) ) ;
#62257=CARTESIAN_POINT ( 'NONE',  ( 11.13873122529103554, 9.084116728910979432, 4.468116630735651462 ) ) ;
#62308=CARTESIAN_POINT ( 'NONE',  ( -11.57163011835881328, 7.018793155873597200, 3.185446920310014640 ) ) ;
#62316=CARTESIAN_POINT ( 'NONE',  ( -11.04678362031243388, 7.051902476693844513, -4.575054176827851649 ) ) ;
#62329=ORIENTED_EDGE ( 'NONE', *, *, #161282, .F. ) ;
#62346=CARTESIAN_POINT ( 'NONE',  ( -11.79409034920973021, 4.782243044590097192, -4.941202808084400822 ) ) ;
#62349=ORIENTED_EDGE ( 'NONE', *, *, #16160, .F. ) ;
#62364=CARTESIAN_POINT ( 'NONE',  ( 11.55950211276791428, 13.88000000000000078, -3.221476510067115662 ) ) ;
#62407=CARTESIAN_POINT ( 'NONE',  ( -11.55950211276791428, 13.88000000000000078, -3.221476510067114329 ) ) ;
#62412=CARTESIAN_POINT ( 'NONE',  ( -9.470156251935129887, 4.005132839944305800, -6.837168546664702085 ) ) ;
#62427=EDGE_CURVE ( 'NONE', #201330, #86850, #766, .T. ) ;
#62433=CARTESIAN_POINT ( 'NONE',  ( 0.000000000000000000, 19.00000000000000000, 0.000000000000000000 ) ) ;
#62453=UNCERTAINTY_MEASURE_WITH_UNIT (LENGTH_MEASURE( 1.000000000000000082E-05 ), #7370, 'distance_accuracy_value', 'NONE');
#62461=CIRCLE ( 'NONE', #41771, 0.07999999999999998779 ) ;
#62506=DIRECTION ( 'NONE',  ( 0.000000000000000000, 9.023263958591316185E-17, -1.000000000000000000 ) ) ;
#62508=FILL_AREA_STYLE ('',( #210883 ) ) ;
#62511=CARTESIAN_POINT ( 'NONE',  ( -10.50060100873255031, 5.377693802073530982, 5.808388628131299747 ) ) ;
#62537=DIRECTION ( 'NONE',  ( 0.000000000000000000, 0.000000000000000000, 1.000000000000000000 ) ) ;
#62546=CARTESIAN_POINT ( 'NONE',  ( 6.902720183911292828, 15.44694763437295570, -9.761920501353822388 ) ) ;
#62570=CARTESIAN_POINT ( 'NONE',  ( -10.39336823037077195, 4.932734307774878424, -5.330979603150785451 ) ) ;
#62585=CARTESIAN_POINT ( 'NONE',  ( 9.984004359900959358, 9.817747272193987129, -6.683988694658842711 ) ) ;
#62594=CARTESIAN_POINT ( 'NONE',  ( 12.12244102266335233, 8.055895858565015999, 3.199560920820632148 ) ) ;
#62603=ORIENTED_EDGE ( 'NONE', *, *, #97745, .T. ) ;
#62609=CARTESIAN_POINT ( 'NONE',  ( 0.06970548857354719186, 14.49233334675339080, 11.99964040467434145 ) ) ;
#62623=CARTESIAN_POINT ( 'NONE',  ( -9.470156251935129887, 4.005132839944305800, -6.837168546664702085 ) ) ;
#62647=CARTESIAN_POINT ( 'NONE',  ( -11.71730914997697326, 8.541829549342406125, -2.386335717864155104 ) ) ;
#62650=VECTOR ( 'NONE', #41214, 1000.000000000000000 ) ;
#62696=CARTESIAN_POINT ( 'NONE',  ( -11.86239285000045918, 9.719999999999998863, -1.812080536912752837 ) ) ;
#62705=DIRECTION ( 'NONE',  ( 3.491481338843133355E-15, 0.000000000000000000, 1.000000000000000000 ) ) ;
#62707=DIRECTION ( 'NONE',  ( 1.000000000000000000, -0.000000000000000000, -0.000000000000000000 ) ) ;
#62746=VERTEX_POINT ( 'NONE', #148542 ) ;
#62806=VERTEX_POINT ( 'NONE', #132320 ) ;
#62812=VECTOR ( 'NONE', #35170, 1000.000000000000000 ) ;
#62830=CARTESIAN_POINT ( 'NONE',  ( 11.35573736746281348, 12.48729585586717761, -3.554362808847921773 ) ) ;
#62832=CARTESIAN_POINT ( 'NONE',  ( 1.250000000000037526, 8.500000000000000000, -12.00100000000000122 ) ) ;
#62850=CARTESIAN_POINT ( 'NONE',  ( -11.07124251632621537, 11.29999999999999716, -0.8054525327832626758 ) ) ;
#62861=CYLINDRICAL_SURFACE ( 'NONE', #2101, 0.3999999999999997446 ) ;
#62889=B_SPLINE_CURVE_WITH_KNOTS ( 'NONE', 3,
 ( #147949, #65583, #78662, #211856, #97084, #48329 ),
 .UNSPECIFIED., .F., .F.,
 ( 4, 2, 4 ),
 ( 0.000000000000000000, 0.0003168911866439334075, 0.0006337823732878668150 ),
 .UNSPECIFIED. ) ;
#62891=DIRECTION ( 'NONE',  ( 0.000000000000000000, 1.000000000000000000, 0.000000000000000000 ) ) ;
#62908=DIRECTION ( 'NONE',  ( 1.000000000000000000, -0.000000000000000000, -0.000000000000000000 ) ) ;
#62915=AXIS2_PLACEMENT_3D ( 'NONE', #160490, #78165, #46764 ) ;
#62916=CYLINDRICAL_SURFACE ( 'NONE', #70747, 0.08000000000000020983 ) ;
#62926=VECTOR ( 'NONE', #36774, 1000.000000000000000 ) ;
#62933=DIRECTION ( 'NONE',  ( 0.000000000000000000, 0.000000000000000000, -1.000000000000000000 ) ) ;
#62966=MECHANICAL_DESIGN_GEOMETRIC_PRESENTATION_REPRESENTATION('',(#146024),#187434);
#62976=DIRECTION ( 'NONE',  ( 1.000000000000000000, -0.000000000000000000, -0.000000000000000000 ) ) ;
#62997=UNCERTAINTY_MEASURE_WITH_UNIT (LENGTH_MEASURE( 1.000000000000000082E-05 ), #177344, 'distance_accuracy_value', 'NONE');
#63045=( GEOMETRIC_REPRESENTATION_CONTEXT ( 3 ) GLOBAL_UNCERTAINTY_ASSIGNED_CONTEXT ( ( #110460 ) ) GLOBAL_UNIT_ASSIGNED_CONTEXT ( ( #176010, #27602, #128405 ) ) REPRESENTATION_CONTEXT ( 'NONE', 'WORKASPACE' ) );
#63047=( GEOMETRIC_REPRESENTATION_CONTEXT ( 3 ) GLOBAL_UNCERTAINTY_ASSIGNED_CONTEXT ( ( #27045 ) ) GLOBAL_UNIT_ASSIGNED_CONTEXT ( ( #109827, #93527, #11166 ) ) REPRESENTATION_CONTEXT ( 'NONE', 'WORKASPACE' ) );
#63071=FACE_OUTER_BOUND ( 'NONE', #14497, .T. ) ;
#63078=EDGE_CURVE ( 'NONE', #116100, #140668, #197925, .T. ) ;
#63088=( NAMED_UNIT ( * ) PLANE_ANGLE_UNIT ( ) SI_UNIT ( $, .RADIAN. ) );
#63108=EDGE_CURVE ( 'NONE', #176917, #81409, #58880, .T. ) ;
#63133=DIRECTION ( 'NONE',  ( -0.000000000000000000, -1.000000000000000000, -0.000000000000000000 ) ) ;
#63135=AXIS2_PLACEMENT_3D ( 'NONE', #23661, #24726, #186159 ) ;
#63143=CARTESIAN_POINT ( 'NONE',  ( 11.63470271956841806, 8.257786514500919495, -2.967717102421748798 ) ) ;
#63150=CARTESIAN_POINT ( 'NONE',  ( -15.75000000000000000, 12.69999999999999929, 0.6999999999999992895 ) ) ;
#63160=CARTESIAN_POINT ( 'NONE',  ( 9.245776177298674625, 13.11974810171090056, -9.005675837709214093 ) ) ;
#63163=ORIENTED_EDGE ( 'NONE', *, *, #68346, .T. ) ;
#63184=CARTESIAN_POINT ( 'NONE',  ( -10.57214848667379314, 5.653292861472692721, 5.679042682613224535 ) ) ;
#63213=CARTESIAN_POINT ( 'NONE',  ( -3.796053574492347593, 14.00000000000182254, 12.24940615670329080 ) ) ;
#63217=CIRCLE ( 'NONE', #191224, 12.00000000000000178 ) ;
#63230=VERTEX_POINT ( 'NONE', #71038 ) ;
#63255=DIRECTION ( 'NONE',  ( 0.000000000000000000, -1.445602896647338917E-16, 1.000000000000000000 ) ) ;
#63259=CARTESIAN_POINT ( 'NONE',  ( 8.597817685116813990, 14.01748360710000085, -7.912049044921352525 ) ) ;
#63262=CARTESIAN_POINT ( 'NONE',  ( 8.771848968578403571, 13.55328059063308999, 7.722295445558531313 ) ) ;
#63296=CARTESIAN_POINT ( 'NONE',  ( -11.19349454483825212, 5.612381422204108183, 3.868266946477203927 ) ) ;
#63315=ORIENTED_EDGE ( 'NONE', *, *, #5255, .F. ) ;
#63322=CARTESIAN_POINT ( 'NONE',  ( 11.28449857580347526, 8.706470588888119977, 3.935098853210270420 ) ) ;
#63328=( GEOMETRIC_REPRESENTATION_CONTEXT ( 3 ) GLOBAL_UNCERTAINTY_ASSIGNED_CONTEXT ( ( #181522 ) ) GLOBAL_UNIT_ASSIGNED_CONTEXT ( ( #154558, #85275, #134068 ) ) REPRESENTATION_CONTEXT ( 'NONE', 'WORKASPACE' ) );
#63350=CIRCLE ( 'NONE', #1001, 0.07999999999999998779 ) ;
#63362=CIRCLE ( 'NONE', #52991, 0.08000000000000014044 ) ;
#63374=CARTESIAN_POINT ( 'NONE',  ( 11.48243876534946217, 9.799999999999998934, -3.200000000000001510 ) ) ;
#63375=CARTESIAN_POINT ( 'NONE',  ( -11.67636001396849998, 7.338531100771467308, 2.777371759657221162 ) ) ;
#63387=SURFACE_STYLE_USAGE ( .BOTH. , #144677 ) ;
#63403=CARTESIAN_POINT ( 'NONE',  ( 0.000000000000000000, 12.30000000000000071, 0.000000000000000000 ) ) ;
#63414=CARTESIAN_POINT ( 'NONE',  ( -12.06798728936711385, 5.701251286509326555, 4.345411722927631004 ) ) ;
#63418=CARTESIAN_POINT ( 'NONE',  ( -15.75000000000000000, 12.29999999999998295, 3.199999999999997957 ) ) ;
#63443=CARTESIAN_POINT ( 'NONE',  ( -1.500000000000039524, 8.500000000000000000, -10.89724735885167739 ) ) ;
#63484=CARTESIAN_POINT ( 'NONE',  ( -10.12724049293007766, 3.240713040256745003, -5.870485300885818880 ) ) ;
#63494=EDGE_CURVE ( 'NONE', #181120, #183276, #139288, .T. ) ;
#63581=CARTESIAN_POINT ( 'NONE',  ( 10.89083482556480575, 8.284139440907676288, -4.931153283774001750 ) ) ;
#63589=CIRCLE ( 'NONE', #170727, 0.5000000000000005551 ) ;
#63597=B_SPLINE_CURVE_WITH_KNOTS ( 'NONE', 3,
 ( #122415, #53047, #22658, #40012, #123486, #88769 ),
 .UNSPECIFIED., .F., .F.,
 ( 4, 2, 4 ),
 ( 0.001916662113439827810, 0.002237152494173779652, 0.002557642874907731494 ),
 .UNSPECIFIED. ) ;
#63610=FILL_AREA_STYLE_COLOUR ( '', #193117 ) ;
#63622=CARTESIAN_POINT ( 'NONE',  ( 7.501393976679871400, 15.44052946730700349, -9.372683453397971931 ) ) ;
#63647=DIRECTION ( 'NONE',  ( 0.000000000000000000, 1.000000000000000000, 0.000000000000000000 ) ) ;
#63648=CARTESIAN_POINT ( 'NONE',  ( -10.10707714348148301, 4.359868340440408829, -5.857196085253971063 ) ) ;
#63649=CARTESIAN_POINT ( 'NONE',  ( 9.452953268198900361, 3.481540744127369802, 7.393265152228856607 ) ) ;
#63663=CARTESIAN_POINT ( 'NONE',  ( 8.880206826883428661, 12.81886467739263402, -8.003364354211651488 ) ) ;
#63672=CARTESIAN_POINT ( 'NONE',  ( 10.32570460010716396, 11.37497670666806826, 7.285500311179339938 ) ) ;
#63680=PRESENTATION_STYLE_ASSIGNMENT (( #160118 ) ) ;
#63711=CARTESIAN_POINT ( 'NONE',  ( -9.367496996292747014, 15.51845925588232333, -7.500000001629758550 ) ) ;
#63792=AXIS2_PLACEMENT_3D ( 'NONE', #95712, #198490, #195324 ) ;
#63821=CARTESIAN_POINT ( 'NONE',  ( 0.000000000000000000, 13.87999999999998302, 0.000000000000000000 ) ) ;
#63839=( GEOMETRIC_REPRESENTATION_CONTEXT ( 3 ) GLOBAL_UNCERTAINTY_ASSIGNED_CONTEXT ( ( #149286 ) ) GLOBAL_UNIT_ASSIGNED_CONTEXT ( ( #76691, #205618, #159022 ) ) REPRESENTATION_CONTEXT ( 'NONE', 'WORKASPACE' ) );
#63863=AXIS2_PLACEMENT_3D ( 'NONE', #88787, #170009, #137539 ) ;
#63899=CARTESIAN_POINT ( 'NONE',  ( 11.48767021851168124, 12.26995772536169227, -3.470194894594655910 ) ) ;
#63919=CARTESIAN_POINT ( 'NONE',  ( -11.04536101718726293, 11.00581159806359288, -1.100000000000000311 ) ) ;
#63931=DIRECTION ( 'NONE',  ( 0.000000000000000000, 0.000000000000000000, -1.000000000000000000 ) ) ;
#63932=PLANE ( 'NONE',  #16988 ) ;
#63936=B_SPLINE_CURVE_WITH_KNOTS ( 'NONE', 3,
 ( #204294, #172917, #42925, #171832, #106890, #24492, #90603, #156663, #142567, #158786, #10383, #8255 ),
 .UNSPECIFIED., .F., .F.,
 ( 4, 2, 2, 2, 2, 4 ),
 ( 4.249187360970357138E-18, 0.0007306567756924711851, 0.001095985163538703254, 0.001461313551384934998, 0.002191970327077403472, 0.002922627102769872164 ),
 .UNSPECIFIED. ) ;
#63945=LINE ( 'NONE', #49827, #142946 ) ;
#63955=CARTESIAN_POINT ( 'NONE',  ( -11.86145016429273191, 10.90000000000000036, 1.099999999999996758 ) ) ;
#63957=CARTESIAN_POINT ( 'NONE',  ( 11.86239285000045740, 11.37999999999999901, -1.812080536912752837 ) ) ;
#63964=CARTESIAN_POINT ( 'NONE',  ( -11.95485154007906914, 9.001110132796746655, 0.3045117111943428934 ) ) ;
#63985=( NAMED_UNIT ( * ) PLANE_ANGLE_UNIT ( ) SI_UNIT ( $, .RADIAN. ) );
#64008=DIRECTION ( 'NONE',  ( 0.000000000000000000, 0.000000000000000000, -1.000000000000000000 ) ) ;
#64016=CARTESIAN_POINT ( 'NONE',  ( -9.670288946796535612, 4.446955533403587069, -7.032531191595068343 ) ) ;
#64039=CARTESIAN_POINT ( 'NONE',  ( -11.44786932348540986, 12.29999999999998295, 3.303370173849762725 ) ) ;
#64050=EDGE_CURVE ( 'NONE', #202127, #193425, #79432, .T. ) ;
#64052=SURFACE_SIDE_STYLE ('',( #197233 ) ) ;
#64085=CARTESIAN_POINT ( 'NONE',  ( 11.86239285000045740, 9.719999999999998863, -1.812080536912752837 ) ) ;
#64100=VERTEX_POINT ( 'NONE', #190426 ) ;
#64106=ORIENTED_EDGE ( 'NONE', *, *, #128500, .F. ) ;
#64143=CARTESIAN_POINT ( 'NONE',  ( -11.94655611907590220, 11.15200944546904083, 1.134828163062136852 ) ) ;
#64145=EDGE_CURVE ( 'NONE', #76712, #136086, #118543, .T. ) ;
#64172=PRESENTATION_STYLE_ASSIGNMENT (( #82535 ) ) ;
#64174=CARTESIAN_POINT ( 'NONE',  ( 11.97302537858596061, 11.29875989808017245, -0.8111997896467566527 ) ) ;
#64185=ORIENTED_EDGE ( 'NONE', *, *, #51352, .T. ) ;
#64186=CIRCLE ( 'NONE', #212890, 11.92000000000000171 ) ;
#64197=LINE ( 'NONE', #52203, #194398 ) ;
#64206=CARTESIAN_POINT ( 'NONE',  ( 9.117697077525853899, 4.000007913748542698, -7.299999999891275237 ) ) ;
#64223=PLANE ( 'NONE',  #119212 ) ;
#64233=CARTESIAN_POINT ( 'NONE',  ( 13.00510994571362033, 6.785533762518828560, -2.157135041233587902 ) ) ;
#64250=CARTESIAN_POINT ( 'NONE',  ( -11.92619526913699879, 10.89999999999998259, 1.328859060402684644 ) ) ;
#64259=EDGE_CURVE ( 'NONE', #37868, #54318, #204528, .T. ) ;
#64268=VECTOR ( 'NONE', #118263, 1000.000000000000000 ) ;
#64280=EDGE_CURVE ( 'NONE', #26907, #172406, #25237, .T. ) ;
#64288=DIRECTION ( 'NONE',  ( 0.000000000000000000, -1.000000000000000000, 0.000000000000000000 ) ) ;
#64292=CARTESIAN_POINT ( 'NONE',  ( -15.75000000000000000, 10.19999999999999929, -1.400000000000001910 ) ) ;
#64310=MECHANICAL_DESIGN_GEOMETRIC_PRESENTATION_REPRESENTATION('',(#36620),#202667);
#64326=VECTOR ( 'NONE', #107516, 1000.000000000000000 ) ;
#64329=CARTESIAN_POINT ( 'NONE',  ( 0.000000000000000000, 3.999999999999996447, 0.000000000000000000 ) ) ;
#64333=CARTESIAN_POINT ( 'NONE',  ( 10.13422073961230119, 13.69230262657890762, -7.310424441678322616 ) ) ;
#64336=CARTESIAN_POINT ( 'NONE',  ( 9.077897083885416052, 13.43124749139993312, 9.116240771241983509 ) ) ;
#64365=CARTESIAN_POINT ( 'NONE',  ( -12.06809232949933275, 5.701620653239091396, -4.345812045493805620 ) ) ;
#64382=CARTESIAN_POINT ( 'NONE',  ( -9.404345922957899617, 14.49023946781299621, 7.453791880843827933 ) ) ;
#64390=VECTOR ( 'NONE', #47160, 1000.000000000000000 ) ;
#64391=CARTESIAN_POINT ( 'NONE',  ( 11.21998530456308174, 8.824241765716642760, 4.114255910918044989 ) ) ;
#64400=DIRECTION ( 'NONE',  ( 0.8594130494132222742, -0.03761243564701257508, -0.5098965730253202100 ) ) ;
#64401=( BOUNDED_SURFACE ( )  B_SPLINE_SURFACE ( 3, 2, ( 
 ( #96565, #194024, #111791 ),
 ( #126995, #208136, #94431 ),
 ( #177796, #80281, #93364 ),
 ( #9944, #142123, #10999 ),
 ( #146380, #213452, #15261 ),
 ( #134398, #166866, #1132 ) ),
 .UNSPECIFIED., .F., .F., .F. ) 
 B_SPLINE_SURFACE_WITH_KNOTS ( ( 4, 2, 4 ),
 ( 3, 3 ),
 ( 0.000000000000000000, 0.0003766365702389426712, 0.0007532731404778853423 ),
 ( 0.000000000000000000, 1.000000000000000000 ),
 .UNSPECIFIED. ) 
 GEOMETRIC_REPRESENTATION_ITEM ( )  RATIONAL_B_SPLINE_SURFACE ( (
 ( 1.000000000000000000, 0.7452309222762957264, 1.000000000000000000),
 ( 1.000000000000000000, 0.7451892422669569305, 1.000000000000000000),
 ( 1.000000000000000000, 0.7429606254241488683, 1.000000000000000000),
 ( 1.000000000000000000, 0.7311462761262982335, 1.000000000000000000),
 ( 1.000000000000000000, 0.7212257702793296588, 1.000000000000000000),
 ( 1.000000000000000000, 0.7071067811865551223, 1.000000000000000000) ) ) 
 REPRESENTATION_ITEM ( '' )  SURFACE ( )  );
#64419=CARTESIAN_POINT ( 'NONE',  ( 11.01135777277262306, 13.39999999999998259, 1.399999999999998579 ) ) ;
#64421=CIRCLE ( 'NONE', #119830, 11.09999999999999964 ) ;
#64429=CARTESIAN_POINT ( 'NONE',  ( -3.530618963777973907, 14.55202870305305929, -11.43095565162720284 ) ) ;
#64441=CARTESIAN_POINT ( 'NONE',  ( -11.91788789707409713, 8.018247624035817367, 1.065403267925175701 ) ) ;
#64449=CARTESIAN_POINT ( 'NONE',  ( -11.90461463783674390, 8.893589831543669888, 1.538977259646465701 ) ) ;
#64473=DIRECTION ( 'NONE',  ( 0.000000000000000000, 1.000000000000000000, 0.000000000000000000 ) ) ;
#64483=ORIENTED_EDGE ( 'NONE', *, *, #48444, .F. ) ;
#64506=CARTESIAN_POINT ( 'NONE',  ( -4.783564408578051541, 15.44696316110051804, 10.96618341542351160 ) ) ;
#64543=CARTESIAN_POINT ( 'NONE',  ( -11.41381675112453564, 13.53005666089993397, -3.704697986577182522 ) ) ;
#64549=CARTESIAN_POINT ( 'NONE',  ( -11.84668730067608600, 10.90000000000000036, -1.400000000000001910 ) ) ;
#64568=CARTESIAN_POINT ( 'NONE',  ( -11.91294103507080315, 13.61460089956407060, 1.446263142085468134 ) ) ;
#64587=FILL_AREA_STYLE_COLOUR ( '', #69412 ) ;
#64610=B_SPLINE_CURVE_WITH_KNOTS ( 'NONE', 3,
 ( #144044, #142970, #61680, #10777, #174391, #158131 ),
 .UNSPECIFIED., .F., .F.,
 ( 4, 2, 4 ),
 ( 0.000000000000000000, 0.0003172254002810711735, 0.0006344508005621423471 ),
 .UNSPECIFIED. ) ;
#64652=DIRECTION ( 'NONE',  ( 1.000000000000000000, -0.000000000000000000, -0.000000000000000000 ) ) ;
#64653=ADVANCED_FACE ( 'NONE', ( #207775 ), #77032, .T. ) ;
#64677=CARTESIAN_POINT ( 'NONE',  ( 9.348761378620913831, 13.52553930298125273, -7.449808453853660417 ) ) ;
#64679=( GEOMETRIC_REPRESENTATION_CONTEXT ( 3 ) GLOBAL_UNCERTAINTY_ASSIGNED_CONTEXT ( ( #166345 ) ) GLOBAL_UNIT_ASSIGNED_CONTEXT ( ( #173248, #75722, #76775 ) ) REPRESENTATION_CONTEXT ( 'NONE', 'WORKASPACE' ) );
#64700=ADVANCED_FACE ( 'NONE', ( #120218 ), #7445, .T. ) ;
#64702=CARTESIAN_POINT ( 'NONE',  ( -10.98545788874447915, 11.25743779547922507, 1.592267205258850460 ) ) ;
#64724=EDGE_LOOP ( 'NONE', ( #136945, #131415, #143734, #73139 ) ) ;
#64726=SURFACE_STYLE_USAGE ( .BOTH. , #80986 ) ;
#64727=CARTESIAN_POINT ( 'NONE',  ( 9.276887557417550667, 13.43425136904641271, -6.782796418722834453 ) ) ;
#64738=CARTESIAN_POINT ( 'NONE',  ( -11.89197415570408900, 12.30000000000000249, 0.8055989572471813354 ) ) ;
#64739=CARTESIAN_POINT ( 'NONE',  ( 7.610320672457040914, 14.45631463746157408, -9.278899351044326949 ) ) ;
#64747=CARTESIAN_POINT ( 'NONE',  ( 0.07926560469698022693, 14.48280592990708726, 11.99972816967717293 ) ) ;
#64761=CARTESIAN_POINT ( 'NONE',  ( -9.812680342707254866, 4.108039100808300148, -6.337802944732694677 ) ) ;
#64764=CARTESIAN_POINT ( 'NONE',  ( -9.407146676474756219, 15.38250095867105216, 7.348982780145517424 ) ) ;
#64804=ORIENTED_EDGE ( 'NONE', *, *, #71437, .F. ) ;
#64844=LINE ( 'NONE', #885, #142884 ) ;
#64871=DIRECTION ( 'NONE',  ( -0.000000000000000000, -1.000000000000000000, -0.000000000000000000 ) ) ;
#64878=CARTESIAN_POINT ( 'NONE',  ( -11.84668730067608600, 12.69999999999998153, 1.399999999999998579 ) ) ;
#64893=CARTESIAN_POINT ( 'NONE',  ( 0.000000000000000000, 8.500000000000000000, 0.000000000000000000 ) ) ;
#64903=AXIS2_PLACEMENT_3D ( 'NONE', #101132, #37210, #169346 ) ;
#64932=CARTESIAN_POINT ( 'NONE',  ( 7.679921558703143525, 14.45948583456419101, 9.166094091849766201 ) ) ;
#64951=CARTESIAN_POINT ( 'NONE',  ( 11.89317557362571698, 11.26275843837589186, 1.599935658896036283 ) ) ;
#64968=EDGE_CURVE ( 'NONE', #76787, #155586, #184145, .T. ) ;
#64981=CYLINDRICAL_SURFACE ( 'NONE', #195866, 0.3999999999999997446 ) ;
#65021=ORIENTED_EDGE ( 'NONE', *, *, #141919, .T. ) ;
#65135=ORIENTED_EDGE ( 'NONE', *, *, #63108, .T. ) ;
#65156=B_SPLINE_CURVE_WITH_KNOTS ( 'NONE', 3,
 ( #129374, #130431, #44857, #176969, #45921, #160716 ),
 .UNSPECIFIED., .F., .F.,
 ( 4, 2, 4 ),
 ( 0.000000000000000000, 0.0003845013059668469482, 0.0007690026119336938965 ),
 .UNSPECIFIED. ) ;
#65177=CARTESIAN_POINT ( 'NONE',  ( -11.96217875511318240, 11.32854366578976624, 0.9561995067075053090 ) ) ;
#65179=CARTESIAN_POINT ( 'NONE',  ( 11.49978884755361008, 11.24270821162803813, -3.429452816445331731 ) ) ;
#65198=ORIENTED_EDGE ( 'NONE', *, *, #171659, .T. ) ;
#65207=DIRECTION ( 'NONE',  ( 0.000000000000000000, 0.000000000000000000, 1.000000000000000000 ) ) ;
#65248=TOROIDAL_SURFACE ( 'NONE', #106763, 11.92000000000000171, 0.08000000000000000167 ) ;
#65249=CARTESIAN_POINT ( 'NONE',  ( -11.84104725192624130, 9.990164625485826733, -1.443823348526935169 ) ) ;
#65256=SURFACE_STYLE_FILL_AREA ( #147612 ) ;
#65268=CARTESIAN_POINT ( 'NONE',  ( 9.781847885788174324, 12.99548848723393490, -8.037988007782987054 ) ) ;
#65315=CARTESIAN_POINT ( 'NONE',  ( -11.94594309014493483, 8.080894294948576473, -0.5280401589721170907 ) ) ;
#65318=CARTESIAN_POINT ( 'NONE',  ( 0.000000000000000000, 0.000000000000000000, 11.92000000000000171 ) ) ;
#65357=B_SPLINE_CURVE_WITH_KNOTS ( 'NONE', 3,
 ( #177038, #128380, #161866, #132582, #168243, #18771, #84855, #2508 ),
 .UNSPECIFIED., .F., .F.,
 ( 4, 2, 2, 4 ),
 ( -5.999999997803333335E-08, 0.001024127516013730770, 0.001536221274020587195, 0.002048315032027443836 ),
 .UNSPECIFIED. ) ;
#65363=CARTESIAN_POINT ( 'NONE',  ( 7.459519926035591553, 16.00000000000000000, -10.25508784514941318 ) ) ;
#65371=ORIENTED_EDGE ( 'NONE', *, *, #126509, .T. ) ;
#65396=CARTESIAN_POINT ( 'NONE',  ( -11.04433755984576848, 5.142917986253679352, 4.203129294766247526 ) ) ;
#65423=CARTESIAN_POINT ( 'NONE',  ( 1.474414414893375769, 7.826756755319755676, -10.64843978026286386 ) ) ;
#65473=CARTESIAN_POINT ( 'NONE',  ( -11.51744110290411882, 7.078546551862022085, -3.212469843298280114 ) ) ;
#65481=( GEOMETRIC_REPRESENTATION_CONTEXT ( 3 ) GLOBAL_UNCERTAINTY_ASSIGNED_CONTEXT ( ( #12623 ) ) GLOBAL_UNIT_ASSIGNED_CONTEXT ( ( #103543, #197829, #100337 ) ) REPRESENTATION_CONTEXT ( 'NONE', 'WORKASPACE' ) );
#65482=FACE_OUTER_BOUND ( 'NONE', #212336, .T. ) ;
#65485=( NAMED_UNIT ( * ) SI_UNIT ( $, .STERADIAN. ) SOLID_ANGLE_UNIT ( ) );
#65515=B_SPLINE_CURVE_WITH_KNOTS ( 'NONE', 3,
 ( #30775, #28629, #126207, #96854, #13429, #145624 ),
 .UNSPECIFIED., .F., .F.,
 ( 4, 2, 4 ),
 ( 0.000000000000000000, 0.5000000000000000000, 1.000000000000000000 ),
 .UNSPECIFIED. ) ;
#65519=ORIENTED_EDGE ( 'NONE', *, *, #90049, .T. ) ;
#65533=CARTESIAN_POINT ( 'NONE',  ( -10.56536251450128994, 12.34038937450521800, 3.404319718479181578 ) ) ;
#65534=CARTESIAN_POINT ( 'NONE',  ( 11.55950211276791784, 13.80000000000000071, -3.221476510067116550 ) ) ;
#65540=SURFACE_STYLE_FILL_AREA ( #15733 ) ;
#65550=CARTESIAN_POINT ( 'NONE',  ( 9.518502046417468776, 4.418053365869078597, 7.307953274077197747 ) ) ;
#65577=LINE ( 'NONE', #64549, #200122 ) ;
#65583=CARTESIAN_POINT ( 'NONE',  ( -11.80247861663003484, 12.30000000000000071, -1.695431928471868632 ) ) ;
#65595=CARTESIAN_POINT ( 'NONE',  ( -11.92051736251533534, 13.65180243792676862, 1.381800029228856808 ) ) ;
#65612=PRESENTATION_STYLE_ASSIGNMENT (( #16872 ) ) ;
#65616=CARTESIAN_POINT ( 'NONE',  ( 11.07790593930098311, 11.29999999999999893, 0.6999999999999992895 ) ) ;
#65671=UNCERTAINTY_MEASURE_WITH_UNIT (LENGTH_MEASURE( 1.000000000000000082E-05 ), #151307, 'distance_accuracy_value', 'NONE');
#65673=SURFACE_STYLE_FILL_AREA ( #51601 ) ;
#65675=DIRECTION ( 'NONE',  ( 0.000000000000000000, 0.000000000000000000, -1.000000000000000000 ) ) ;
#65706=ADVANCED_FACE ( 'NONE', ( #205727 ), #57364, .F. ) ;
#65710=CARTESIAN_POINT ( 'NONE',  ( 11.94105721237523277, 10.19999999999999929, -1.187919463087248939 ) ) ;
#65727=AXIS2_PLACEMENT_3D ( 'NONE', #123026, #91514, #70935 ) ;
#65730=ORIENTED_EDGE ( 'NONE', *, *, #197971, .F. ) ;
#65739=CARTESIAN_POINT ( 'NONE',  ( -9.348526197514022584, 4.999985930147239799, -7.001887667968696327 ) ) ;
#65740=CARTESIAN_POINT ( 'NONE',  ( 9.681502918193430673, 4.134753598976697475, 7.090028296829109067 ) ) ;
#65764=CARTESIAN_POINT ( 'NONE',  ( 9.553701449168967130, 11.68847306586624768, 6.138592618161210268 ) ) ;
#65773=DIRECTION ( 'NONE',  ( 0.000000000000000000, 0.000000000000000000, 1.000000000000000000 ) ) ;
#65778=CARTESIAN_POINT ( 'NONE',  ( 11.80247861663003484, 11.30000000000000249, -1.695431928471867966 ) ) ;
#65788=CARTESIAN_POINT ( 'NONE',  ( 9.476364758792197307, 3.602180318966379247, -7.289720839516039774 ) ) ;
#65796=DIRECTION ( 'NONE',  ( 0.000000000000000000, 0.000000000000000000, 1.000000000000000000 ) ) ;
#65850=CYLINDRICAL_SURFACE ( 'NONE', #2590, 0.3999999999999997446 ) ;
#65872=DIRECTION ( 'NONE',  ( 0.000000000000000000, -7.228014483236694583E-17, 1.000000000000000000 ) ) ;
#65909=DIRECTION ( 'NONE',  ( 0.000000000000000000, 0.000000000000000000, -1.000000000000000000 ) ) ;
#65969=LINE ( 'NONE', #130032, #201853 ) ;
#65973=AXIS2_PLACEMENT_3D ( 'NONE', #66800, #34332, #83077 ) ;
#66024=ORIENTED_EDGE ( 'NONE', *, *, #81633, .T. ) ;
#66028=CARTESIAN_POINT ( 'NONE',  ( -9.348561386651960348, 4.000000000000000888, 7.001914024036569373 ) ) ;
#66040=VECTOR ( 'NONE', #42219, 1000.000000000000000 ) ;
#66051=FACE_OUTER_BOUND ( 'NONE', #11529, .T. ) ;
#66075=CARTESIAN_POINT ( 'NONE',  ( 11.97929049433705373, 12.22000000000000064, -0.7046979865771834106 ) ) ;
#66096=CIRCLE ( 'NONE', #45434, 0.07999999999999998779 ) ;
#66099=FACE_OUTER_BOUND ( 'NONE', #27170, .T. ) ;
#66139=ADVANCED_FACE ( 'NONE', ( #106706 ), #77186, .T. ) ;
#66171=CARTESIAN_POINT ( 'NONE',  ( 11.86145016429273191, 13.40000000000000036, 1.099999999999996758 ) ) ;
#66179=VERTEX_POINT ( 'NONE', #169511 ) ;
#66211=CARTESIAN_POINT ( 'NONE',  ( 1.250000000000037526, 8.500000000000000000, 12.00100000000000122 ) ) ;
#66223=VERTEX_POINT ( 'NONE', #40600 ) ;
#66231=CARTESIAN_POINT ( 'NONE',  ( -11.78331023100045627, 12.30000000000000071, -1.800000000000001155 ) ) ;
#66243=B_SPLINE_CURVE_WITH_KNOTS ( 'NONE', 3,
 ( #137832, #105339, #86931, #123796, #172458, #135693 ),
 .UNSPECIFIED., .F., .F.,
 ( 4, 2, 4 ),
 ( 0.000000000000000000, 0.0003258677429877278493, 0.0006517354859754556987 ),
 .UNSPECIFIED. ) ;
#66250=VERTEX_POINT ( 'NONE', #10209 ) ;
#66261=VERTEX_POINT ( 'NONE', #12334 ) ;
#66268=EDGE_CURVE ( 'NONE', #72818, #154255, #127263, .T. ) ;
#66272=CARTESIAN_POINT ( 'NONE',  ( 0.01853512708399032358, 14.54363643945355555, 11.97163374478178710 ) ) ;
#66312=ADVANCED_FACE ( 'NONE', ( #157553 ), #190027, .F. ) ;
#66314=FILL_AREA_STYLE ('',( #103119 ) ) ;
#66324=CARTESIAN_POINT ( 'NONE',  ( 9.545480790392691262, 12.19169623295751315, -8.744449518525772902 ) ) ;
#66332=B_SPLINE_CURVE_WITH_KNOTS ( 'NONE', 3,
 ( #140216, #107755, #75188, #158575, #89315, #125090 ),
 .UNSPECIFIED., .F., .F.,
 ( 4, 2, 4 ),
 ( 0.000000000000000000, 0.0003779448103413554443, 0.0007558896206827108886 ),
 .UNSPECIFIED. ) ;
#66337=CARTESIAN_POINT ( 'NONE',  ( -15.75000000000000000, 9.799999999999998934, -0.7000000000000009548 ) ) ;
#66341=COLOUR_RGB ( '', 0.72549020, 0.75294118, 0.79215686) ;
#66343=CARTESIAN_POINT ( 'NONE',  ( 11.48243876534946217, 11.29999999999999893, -3.200000000000001510 ) ) ;
#66365=CARTESIAN_POINT ( 'NONE',  ( 0.000000000000000000, 13.79999999999999893, 0.000000000000000000 ) ) ;
#66381=AXIS2_PLACEMENT_3D ( 'NONE', #40785, #154522, #138279 ) ;
#66401=DIRECTION ( 'NONE',  ( 0.000000000000000000, -0.000000000000000000, 1.000000000000000000 ) ) ;
#66402=CIRCLE ( 'NONE', #156436, 0.08000000000000020983 ) ;
#66421=CARTESIAN_POINT ( 'NONE',  ( 10.12759493444457171, 13.73870611316562851, -7.322964122302763279 ) ) ;
#66441=ORIENTED_EDGE ( 'NONE', *, *, #81363, .F. ) ;
#66466=DIRECTION ( 'NONE',  ( 0.000000000000000000, 0.000000000000000000, 1.000000000000000000 ) ) ;
#66493=CARTESIAN_POINT ( 'NONE',  ( 11.78331023100045627, 12.30000000000000071, -1.800000000000001155 ) ) ;
#66495=AXIS2_PLACEMENT_3D ( 'NONE', #108486, #28231, #78042 ) ;
#66526=CARTESIAN_POINT ( 'NONE',  ( -11.86145017031081217, 12.59418046486151077, -1.100000000000000533 ) ) ;
#66528=CARTESIAN_POINT ( 'NONE',  ( -11.45615580362692221, 6.921991398061194900, -3.423271987478961886 ) ) ;
#66538=CARTESIAN_POINT ( 'NONE',  ( -11.59482873632621036, 8.292847044363275799, 2.925048987524553556 ) ) ;
#66553=AXIS2_PLACEMENT_3D ( 'NONE', #52151, #2295, #85708 ) ;
#66554=CARTESIAN_POINT ( 'NONE',  ( -11.94105721237523099, 10.19999999999999929, -1.187919463087249827 ) ) ;
#66582=DIRECTION ( 'NONE',  ( 1.000000000000000000, -0.000000000000000000, -0.000000000000000000 ) ) ;
#66665=FILL_AREA_STYLE_COLOUR ( '', #91814 ) ;
#66671=UNCERTAINTY_MEASURE_WITH_UNIT (LENGTH_MEASURE( 1.000000000000000082E-05 ), #76426, 'distance_accuracy_value', 'NONE');
#66698=CARTESIAN_POINT ( 'NONE',  ( -10.85768919388902809, 5.702095803505641491, 6.451939001899068771 ) ) ;
#66709=CARTESIAN_POINT ( 'NONE',  ( 11.55950211276791251, 13.88000000000000078, -3.221476510067114329 ) ) ;
#66722=ORIENTED_EDGE ( 'NONE', *, *, #99349, .F. ) ;
#66766=ORIENTED_EDGE ( 'NONE', *, *, #96671, .F. ) ;
#66800=CARTESIAN_POINT ( 'NONE',  ( 11.33772463945036790, 12.69999999999999929, -3.680000000000001048 ) ) ;
#66815=CARTESIAN_POINT ( 'NONE',  ( 10.35782045828010745, 9.182042646633135519, 6.014258400289742568 ) ) ;
#66827=CARTESIAN_POINT ( 'NONE',  ( 11.15461176689735012, 7.620380504396416121, -0.7938402394984110932 ) ) ;
#66837=CARTESIAN_POINT ( 'NONE',  ( 7.585545081070966589, 14.47801472900905395, -9.241967501645218519 ) ) ;
#66840=EDGE_CURVE ( 'NONE', #105543, #144349, #177537, .T. ) ;
#66856=CARTESIAN_POINT ( 'NONE',  ( -15.75000000000000000, 13.39999999999998259, 3.599999999999999201 ) ) ;
#66862=ORIENTED_EDGE ( 'NONE', *, *, #180960, .T. ) ;
#66889=B_SPLINE_CURVE_WITH_KNOTS ( 'NONE', 3,
 ( #70056, #149199, #53843, #167586, #67912, #18109 ),
 .UNSPECIFIED., .F., .F.,
 ( 4, 2, 4 ),
 ( 0.000000000000000000, 0.0003778774010236167534, 0.0007557548020472335069 ),
 .UNSPECIFIED. ) ;
#66895=EDGE_LOOP ( 'NONE', ( #196862, #137191, #160667, #78121 ) ) ;
#66939=CARTESIAN_POINT ( 'NONE',  ( -11.86145017354119879, 10.09514365543875769, 1.099999999999996980 ) ) ;
#66957=CARTESIAN_POINT ( 'NONE',  ( 11.55950211276791251, 12.29999999999998472, 3.221476510067111665 ) ) ;
#66969=EDGE_CURVE ( 'NONE', #28791, #56620, #179698, .T. ) ;
#66970=CARTESIAN_POINT ( 'NONE',  ( -10.62873463776380056, 11.29999999999999893, -3.200000000000001510 ) ) ;
#66990=( NAMED_UNIT ( * ) PLANE_ANGLE_UNIT ( ) SI_UNIT ( $, .RADIAN. ) );
#67012=SURFACE_SIDE_STYLE ('',( #103823 ) ) ;
#67013=AXIS2_PLACEMENT_3D ( 'NONE', #98911, #194264, #97855 ) ;
#67080=CARTESIAN_POINT ( 'NONE',  ( 11.88156762547253997, 9.720000084540316720, -1.686557021358706443 ) ) ;
#67082=( BOUNDED_SURFACE ( )  B_SPLINE_SURFACE ( 3, 2, ( 
 ( #32774, #14368, #131398 ),
 ( #180097, #115157, #52225 ),
 ( #65249, #133512, #118353 ),
 ( #197395, #97796, #80459 ),
 ( #147603, #146557, #181152 ),
 ( #182206, #213621, #164904 ) ),
 .UNSPECIFIED., .F., .F., .T. ) 
 B_SPLINE_SURFACE_WITH_KNOTS ( ( 4, 2, 4 ),
 ( 3, 3 ),
 ( 0.000000000000000000, 0.0003766365702389428338, 0.0007532731404778856676 ),
 ( 0.000000000000000000, 1.000000000000000000 ),
 .UNSPECIFIED. ) 
 GEOMETRIC_REPRESENTATION_ITEM ( )  RATIONAL_B_SPLINE_SURFACE ( (
 ( 1.000000000000000000, 0.7452309222762957264, 1.000000000000000000),
 ( 1.000000000000000000, 0.7451892422672021787, 1.000000000000000000),
 ( 1.000000000000000000, 0.7429606254238220187, 1.000000000000000000),
 ( 1.000000000000000000, 0.7311462761266275256, 1.000000000000000000),
 ( 1.000000000000000000, 0.7212257702790848546, 1.000000000000000000),
 ( 1.000000000000000000, 0.7071067811865551223, 1.000000000000000000) ) ) 
 REPRESENTATION_ITEM ( '' )  SURFACE ( )  );
#67096=CARTESIAN_POINT ( 'NONE',  ( 8.737618474220361975, 14.93717167570155446, 8.231545548724737316 ) ) ;
#67100=DIRECTION ( 'NONE',  ( 1.000000000000000000, -0.000000000000000000, -0.000000000000000000 ) ) ;
#67111=ORIENTED_EDGE ( 'NONE', *, *, #98727, .T. ) ;
#67113=ORIENTED_EDGE ( 'NONE', *, *, #152281, .T. ) ;
#67119=STYLED_ITEM ( 'NONE', ( #152830 ), #2404 ) ;
#67127=CARTESIAN_POINT ( 'NONE',  ( -11.59427420681528709, 8.291911680476573565, -2.926947285362574203 ) ) ;
#67130=CARTESIAN_POINT ( 'NONE',  ( 9.508009452561562824, 4.000000000000000888, -7.612500000000001599 ) ) ;
#67145=SURFACE_STYLE_FILL_AREA ( #79163 ) ;
#67165=CIRCLE ( 'NONE', #18645, 11.09999999999999964 ) ;
#67171=EDGE_LOOP ( 'NONE', ( #178781, #47894, #203844, #135507 ) ) ;
#67177=FILL_AREA_STYLE ('',( #200384 ) ) ;
#67178=DIRECTION ( 'NONE',  ( -0.000000000000000000, -1.000000000000000000, -0.000000000000000000 ) ) ;
#67180=CARTESIAN_POINT ( 'NONE',  ( 0.000000000000000000, 19.00000000000000000, -12.00000000000000178 ) ) ;
#67181=EDGE_CURVE ( 'NONE', #158693, #119038, #200171, .T. ) ;
#67194=DIRECTION ( 'NONE',  ( 0.000000000000000000, 0.000000000000000000, -1.000000000000000000 ) ) ;
#67232=MECHANICAL_DESIGN_GEOMETRIC_PRESENTATION_REPRESENTATION('',(#174599),#75939);
#67257=VERTEX_POINT ( 'NONE', #69098 ) ;
#67324=CARTESIAN_POINT ( 'NONE',  ( -0.8965429266985017742, 15.44733976321393953, -11.92417820654543448 ) ) ;
#67325=CARTESIAN_POINT ( 'NONE',  ( 11.94105721237522921, 10.90000000000000036, -1.187919463087248939 ) ) ;
#67353=CARTESIAN_POINT ( 'NONE',  ( -11.48243876534946040, 12.30000000000000071, -3.200000000000001510 ) ) ;
#67376=CARTESIAN_POINT ( 'NONE',  ( -11.78039045457385292, 4.728130269440308453, 4.968650233931813709 ) ) ;
#67379=SURFACE_SIDE_STYLE ('',( #199526 ) ) ;
#67390=CARTESIAN_POINT ( 'NONE',  ( 10.81010058466664425, 10.31570469300483950, 6.498163104334348183 ) ) ;
#67402=CARTESIAN_POINT ( 'NONE',  ( -0.8997935122536572239, 14.48154075026818965, 12.00000000000000000 ) ) ;
#67404=FACE_OUTER_BOUND ( 'NONE', #18670, .T. ) ;
#67434=ADVANCED_FACE ( 'NONE', ( #890 ), #51757, .T. ) ;
#67439=CARTESIAN_POINT ( 'NONE',  ( -9.748930057865852206, 3.057420161666833280, -6.444087955423147385 ) ) ;
#67466=( NAMED_UNIT ( * ) PLANE_ANGLE_UNIT ( ) SI_UNIT ( $, .RADIAN. ) );
#67488=CARTESIAN_POINT ( 'NONE',  ( 8.346583974317809407, 13.15480872911727594, -8.542606490713003708 ) ) ;
#67497=EDGE_CURVE ( 'NONE', #139854, #209617, #174747, .T. ) ;
#67507=CARTESIAN_POINT ( 'NONE',  ( 10.59763834280244232, 12.29999999999999893, -3.303285708550596222 ) ) ;
#67518=CARTESIAN_POINT ( 'NONE',  ( -10.99931038725301846, 6.873658557531565627, -3.960823121322395224 ) ) ;
#67549=FACE_OUTER_BOUND ( 'NONE', #124933, .T. ) ;
#67561=CARTESIAN_POINT ( 'NONE',  ( 11.84101807917483740, 9.989784997391206289, 1.444039656437077657 ) ) ;
#67603=CARTESIAN_POINT ( 'NONE',  ( -11.33454210411463059, 7.665656903368001096, 3.947969875293493747 ) ) ;
#67615=ADVANCED_FACE ( 'NONE', ( #114501 ), #27847, .T. ) ;
#67616=MECHANICAL_DESIGN_GEOMETRIC_PRESENTATION_REPRESENTATION('',(#195536),#81430);
#67621=TOROIDAL_SURFACE ( 'NONE', #95204, 11.92000000000000171, 0.08000000000000000167 ) ;
#67700=ORIENTED_EDGE ( 'NONE', *, *, #55489, .F. ) ;
#67738=EDGE_CURVE ( 'NONE', #210434, #179460, #192715, .T. ) ;
#67764=CARTESIAN_POINT ( 'NONE',  ( 0.6674790882332717334, 15.00000000000000888, -11.66566053519550827 ) ) ;
#67766=CARTESIAN_POINT ( 'NONE',  ( -10.60630588279735242, 5.715763139788331948, 4.896273837757428637 ) ) ;
#67789=ORIENTED_EDGE ( 'NONE', *, *, #79325, .F. ) ;
#67796=UNCERTAINTY_MEASURE_WITH_UNIT (LENGTH_MEASURE( 1.000000000000000082E-05 ), #49934, 'distance_accuracy_value', 'NONE');
#67810=AXIS2_PLACEMENT_3D ( 'NONE', #28240, #166770, #51958 ) ;
#67817=MECHANICAL_DESIGN_GEOMETRIC_PRESENTATION_REPRESENTATION('',(#199581),#137138);
#67840=CARTESIAN_POINT ( 'NONE',  ( 11.94650005372638013, 9.948972996623616893, -1.135399707157281890 ) ) ;
#67868=CARTESIAN_POINT ( 'NONE',  ( -10.87107728089202752, 4.495199002972934288, -4.557510466808897043 ) ) ;
#67887=CARTESIAN_POINT ( 'NONE',  ( 11.84050473577397966, 6.857368744533671290, -1.964541968951881490 ) ) ;
#67891=ORIENTED_EDGE ( 'NONE', *, *, #171810, .T. ) ;
#67896=EDGE_LOOP ( 'NONE', ( #174478, #125021, #75552, #106237 ) ) ;
#67899=CARTESIAN_POINT ( 'NONE',  ( 9.997100500050640548, 9.889488447269407345, -5.009837084036856680 ) ) ;
#67912=CARTESIAN_POINT ( 'NONE',  ( -11.88168329227126563, 12.22000000000000064, -1.685799833707130269 ) ) ;
#67939=CARTESIAN_POINT ( 'NONE',  ( 0.000000000000000000, 1.016439536705160407E-16, 11.18000000000000149 ) ) ;
#67955=AXIS2_PLACEMENT_3D ( 'NONE', #152392, #156674, #135094 ) ;
#67971=CARTESIAN_POINT ( 'NONE',  ( 0.000000000000000000, 13.88000000000000078, 0.000000000000000000 ) ) ;
#67973=B_SPLINE_CURVE_WITH_KNOTS ( 'NONE', 3,
 ( #118276, #19633, #183206, #50015, #100887, #33757 ),
 .UNSPECIFIED., .F., .F.,
 ( 4, 2, 4 ),
 ( 0.000000000000000000, 0.0003172254002810696557, 0.0006344508005621393113 ),
 .UNSPECIFIED. ) ;
#68008=CARTESIAN_POINT ( 'NONE',  ( -11.94980361723156292, 10.09761943414563845, 1.099999926404457984 ) ) ;
#68019=UNCERTAINTY_MEASURE_WITH_UNIT (LENGTH_MEASURE( 1.000000000000000082E-05 ), #72500, 'distance_accuracy_value', 'NONE');
#68025=CARTESIAN_POINT ( 'NONE',  ( 10.92268642758943642, 8.218322760642331914, -4.985627623770443329 ) ) ;
#68058=UNCERTAINTY_MEASURE_WITH_UNIT (LENGTH_MEASURE( 1.000000000000000082E-05 ), #89298, 'distance_accuracy_value', 'NONE');
#68069=ADVANCED_FACE ( 'NONE', ( #151202 ), #176372, .T. ) ;
#68107=CARTESIAN_POINT ( 'NONE',  ( 8.621587210660656808, 13.70538846753250795, 8.347036492328824053 ) ) ;
#68124=EDGE_CURVE ( 'NONE', #198880, #200740, #115316, .T. ) ;
#68167=SURFACE_STYLE_USAGE ( .BOTH. , #134299 ) ;
#68169=CARTESIAN_POINT ( 'NONE',  ( -10.55163518180063242, 5.124035624933899413, 7.011265714045999076 ) ) ;
#68173=( BOUNDED_SURFACE ( )  B_SPLINE_SURFACE ( 3, 2, ( 
 ( #3659, #51392, #200800 ),
 ( #16724, #50320, #102259 ),
 ( #68670, #184564, #149962 ),
 ( #183506, #198675, #151032 ),
 ( #66526, #19928, #165133 ),
 ( #82809, #132669, #54581 ) ),
 .UNSPECIFIED., .F., .F., .T. ) 
 B_SPLINE_SURFACE_WITH_KNOTS ( ( 4, 2, 4 ),
 ( 3, 3 ),
 ( 0.000000000000000000, 0.0003754689591423961527, 0.0007509379182847923054 ),
 ( 0.000000000000000000, 1.000000000000000000 ),
 .UNSPECIFIED. ) 
 GEOMETRIC_REPRESENTATION_ITEM ( )  RATIONAL_B_SPLINE_SURFACE ( (
 ( 1.000000000000000000, 0.7071067811865475727, 1.000000000000000000),
 ( 1.000000000000000000, 0.7018599272026954106, 1.000000000000000000),
 ( 1.000000000000000000, 0.6927733177256546471, 1.000000000000000000),
 ( 1.000000000000000000, 0.6772007068877438085, 1.000000000000000000),
 ( 1.000000000000000000, 0.6709974581634233770, 1.000000000000000000),
 ( 1.000000000000000000, 0.6711954675835484219, 1.000000000000000000) ) ) 
 REPRESENTATION_ITEM ( '' )  SURFACE ( )  );
#68187=CARTESIAN_POINT ( 'NONE',  ( 0.000000000000000000, 15.00041888085534758, 0.000000000000000000 ) ) ;
#68195=CARTESIAN_POINT ( 'NONE',  ( -10.49167095263961613, 5.343775707538777731, -5.730694126968513658 ) ) ;
#68213=B_SPLINE_CURVE_WITH_KNOTS ( 'NONE', 3,
 ( #36831, #118162, #184147, #102914, #20575, #86659 ),
 .UNSPECIFIED., .F., .F.,
 ( 4, 2, 4 ),
 ( 0.000000000000000000, 0.0003172254002810694388, 0.0006344508005621388776 ),
 .UNSPECIFIED. ) ;
#68215=CARTESIAN_POINT ( 'NONE',  ( 0.000000000000000000, 12.30000000000000071, 0.000000000000000000 ) ) ;
#68216=FACE_OUTER_BOUND ( 'NONE', #97335, .T. ) ;
#68227=SURFACE_STYLE_USAGE ( .BOTH. , #119196 ) ;
#68238=CARTESIAN_POINT ( 'NONE',  ( -11.97929049433705551, 11.29999999999999893, 0.7046979865771804130 ) ) ;
#68247=FILL_AREA_STYLE_COLOUR ( '', #133929 ) ;
#68248=CARTESIAN_POINT ( 'NONE',  ( -10.79163161203180543, 4.451778906049931095, 5.251089395658656400 ) ) ;
#68259=ORIENTED_EDGE ( 'NONE', *, *, #173988, .F. ) ;
#68268=CARTESIAN_POINT ( 'NONE',  ( -8.767665818636368513, 15.44694762192558279, 8.178568214798543679 ) ) ;
#68271=STYLED_ITEM ( 'NONE', ( #40424 ), #101103 ) ;
#68301=AXIS2_PLACEMENT_3D ( 'NONE', #103734, #54979, #173010 ) ;
#68305=EDGE_CURVE ( 'NONE', #209617, #93151, #210758, .T. ) ;
#68317=DIRECTION ( 'NONE',  ( 0.000000000000000000, 0.000000000000000000, -1.000000000000000000 ) ) ;
#68318=CARTESIAN_POINT ( 'NONE',  ( -9.348561386651960348, 4.000000000000000888, 7.001914024036569373 ) ) ;
#68346=EDGE_CURVE ( 'NONE', #61789, #173182, #187304, .T. ) ;
#68347=CARTESIAN_POINT ( 'NONE',  ( 11.86145016429273191, 10.09412123665269689, 1.099999999999996758 ) ) ;
#68354=CARTESIAN_POINT ( 'NONE',  ( 11.07790593930098311, 12.30000000000000071, 0.6999999999999992895 ) ) ;
#68369=CARTESIAN_POINT ( 'NONE',  ( -10.85972809853354093, 4.659267788818126199, -5.106963847164690762 ) ) ;
#68375=CARTESIAN_POINT ( 'NONE',  ( -11.91294103507081026, 12.48539910043594503, -1.446263142085586262 ) ) ;
#68384=VECTOR ( 'NONE', #89043, 1000.000000000000000 ) ;
#68396=DIRECTION ( 'NONE',  ( -0.000000000000000000, -1.000000000000000000, -0.000000000000000000 ) ) ;
#68402=CARTESIAN_POINT ( 'NONE',  ( 0.000000000000000000, 8.500000000000000000, 0.000000000000000000 ) ) ;
#68434=ADVANCED_FACE ( 'NONE', ( #83871 ), #68173, .T. ) ;
#68435=CARTESIAN_POINT ( 'NONE',  ( 9.508009452561562824, 4.000000000000000888, 7.612500000000001599 ) ) ;
#68439=VECTOR ( 'NONE', #142730, 1000.000000000000000 ) ;
#68443=EDGE_LOOP ( 'NONE', ( #144118, #197274, #1825, #32053 ) ) ;
#68455=CARTESIAN_POINT ( 'NONE',  ( -11.31087111570240467, 5.182330806778288057, -5.726608797552268371 ) ) ;
#68457=CARTESIAN_POINT ( 'NONE',  ( -15.75000000000000000, 13.39999999999998259, 1.799999999999999600 ) ) ;
#68468=CARTESIAN_POINT ( 'NONE',  ( 11.15162045555251957, 9.712998552558403276, 5.837063001226317382 ) ) ;
#68475=CARTESIAN_POINT ( 'NONE',  ( -10.50000000000000533, 13.50709944181895139, 3.599999999999998312 ) ) ;
#68507=DIRECTION ( 'NONE',  ( -0.7806247490453480653, -4.396526966619892032E-05, 0.6249999993959538536 ) ) ;
#68519=CARTESIAN_POINT ( 'NONE',  ( -11.86691703139814535, 7.727552885927400084, -1.800178980557079367 ) ) ;
#68534=ORIENTED_EDGE ( 'NONE', *, *, #175999, .T. ) ;
#68543=FILL_AREA_STYLE ('',( #133612 ) ) ;
#68564=CARTESIAN_POINT ( 'NONE',  ( 8.830611090300100940, 13.64794954589311082, -9.281763806552183027 ) ) ;
#68572=DIRECTION ( 'NONE',  ( 1.224643483124941457E-16, 0.002327115863041261980, 0.9999972922622142324 ) ) ;
#68592=CARTESIAN_POINT ( 'NONE',  ( -10.50659947519749693, 5.359800460605414152, -5.105385958519358169 ) ) ;
#68595=CIRCLE ( 'NONE', #144735, 0.08000000000000040412 ) ;
#68614=CARTESIAN_POINT ( 'NONE',  ( -9.404393214968951753, 15.50974221445264156, 7.453732458498741664 ) ) ;
#68619=CARTESIAN_POINT ( 'NONE',  ( -15.75000000000000000, 10.90000000000000036, 1.099999999999996758 ) ) ;
#68625=CARTESIAN_POINT ( 'NONE',  ( 11.94105721237522921, 13.40000000000000036, -1.187919463087248939 ) ) ;
#68630=CARTESIAN_POINT ( 'NONE',  ( 8.213877987985293672, 14.20293839921164469, -8.687862046754464274 ) ) ;
#68635=CARTESIAN_POINT ( 'NONE',  ( -11.92619525870747665, 11.02622296793678025, 1.328859154005173959 ) ) ;
#68660=EDGE_CURVE ( 'NONE', #13289, #148685, #63589, .T. ) ;
#68661=CARTESIAN_POINT ( 'NONE',  ( -4.369846591600387242, 14.55265095719298252, -11.13739096725714894 ) ) ;
#68668=CARTESIAN_POINT ( 'NONE',  ( -15.75000000000000000, 13.40000000000000036, -0.7000000000000009548 ) ) ;
#68670=CARTESIAN_POINT ( 'NONE',  ( -11.88237264505823987, 12.34322961531690410, -0.9087825512663008087 ) ) ;
#68680=CARTESIAN_POINT ( 'NONE',  ( -11.29625252127160628, 7.648179254756541035, 3.920601804043121419 ) ) ;
#68683=SURFACE_SIDE_STYLE ('',( #117525 ) ) ;
#68710=ORIENTED_EDGE ( 'NONE', *, *, #6564, .F. ) ;
#68716=ORIENTED_EDGE ( 'NONE', *, *, #191917, .F. ) ;
#68729=CARTESIAN_POINT ( 'NONE',  ( -10.51595811585100648, 13.61340346008145019, -3.553980774159643197 ) ) ;
#68777=CARTESIAN_POINT ( 'NONE',  ( 0.000000000000000000, 0.08000000000000020983, 0.000000000000000000 ) ) ;
#68795=CARTESIAN_POINT ( 'NONE',  ( -11.80251051724219202, 13.79999999999998295, 1.695257889419070851 ) ) ;
#68798=DIRECTION ( 'NONE',  ( -1.000000000000000000, 5.578174157656879309E-15, -1.224646799147768099E-16 ) ) ;
#68818=CARTESIAN_POINT ( 'NONE',  ( 0.000000000000000000, 14.55305236562704252, -11.95586206896551928 ) ) ;
#68846=CARTESIAN_POINT ( 'NONE',  ( -10.61922739175395236, 7.618143447610075114, 4.514851702475597861 ) ) ;
#68869=ORIENTED_EDGE ( 'NONE', *, *, #98123, .T. ) ;
#68877=CARTESIAN_POINT ( 'NONE',  ( -15.75000000000000000, 12.69999999999998153, 1.399999999999998579 ) ) ;
#68893=DIRECTION ( 'NONE',  ( 0.000000000000000000, 0.000000000000000000, -1.000000000000000000 ) ) ;
#68896=STYLED_ITEM ( 'NONE', ( #11962 ), #10478 ) ;
#68911=ORIENTED_EDGE ( 'NONE', *, *, #113819, .F. ) ;
#68915=( NAMED_UNIT ( * ) SI_UNIT ( $, .STERADIAN. ) SOLID_ANGLE_UNIT ( ) );
#68934=ORIENTED_EDGE ( 'NONE', *, *, #3938, .T. ) ;
#68942=CARTESIAN_POINT ( 'NONE',  ( -11.94105721237523099, 11.02740390989733221, -1.187919463087249827 ) ) ;
#68945=CARTESIAN_POINT ( 'NONE',  ( -11.05174500248992331, 4.511067306307721125, -6.216760965876352962 ) ) ;
#68952=CARTESIAN_POINT ( 'NONE',  ( 8.790098660144264997, 13.29414747594432455, 8.101455065885630802 ) ) ;
#68956=PRESENTATION_STYLE_ASSIGNMENT (( #84165 ) ) ;
#68963=CARTESIAN_POINT ( 'NONE',  ( 11.05588078634535698, 8.012831956445918280, -4.553764956315686341 ) ) ;
#68975=PLANE ( 'NONE',  #192592 ) ;
#68976=CARTESIAN_POINT ( 'NONE',  ( 9.262488864310125081, 13.63671387857607975, 6.830742452943137089 ) ) ;
#68988=CARTESIAN_POINT ( 'NONE',  ( 8.628817749835317130, 13.71606850217345119, -8.341300610551938277 ) ) ;
#69019=FILL_AREA_STYLE_COLOUR ( '', #50257 ) ;
#69029=AXIS2_PLACEMENT_3D ( 'NONE', #35072, #16685, #32963 ) ;
#69038=DIRECTION ( 'NONE',  ( 1.000000000000000000, -0.000000000000000000, -0.000000000000000000 ) ) ;
#69098=CARTESIAN_POINT ( 'NONE',  ( 11.94105721237523277, 10.90000000000000036, -1.187919463087249827 ) ) ;
#69128=CARTESIAN_POINT ( 'NONE',  ( 11.94105721237522921, 13.52740390989733221, 1.187919463087248273 ) ) ;
#69137=DIRECTION ( 'NONE',  ( 2.486899575160350966E-14, 0.000000000000000000, -1.000000000000000000 ) ) ;
#69142=EDGE_CURVE ( 'NONE', #77381, #147625, #134586, .T. ) ;
#69148=FACE_OUTER_BOUND ( 'NONE', #14547, .T. ) ;
#69155=ADVANCED_FACE ( 'NONE', ( #183290 ), #198459, .F. ) ;
#69227=EDGE_CURVE ( 'NONE', #135649, #66179, #172030, .T. ) ;
#69232=ORIENTED_EDGE ( 'NONE', *, *, #25480, .T. ) ;
#69234=( LENGTH_UNIT ( ) NAMED_UNIT ( * ) SI_UNIT ( .MILLI., .METRE. ) );
#69235=CARTESIAN_POINT ( 'NONE',  ( -9.706334639731263536, 5.108299517166001280, 6.477055075394225092 ) ) ;
#69237=CARTESIAN_POINT ( 'NONE',  ( -15.75000000000000000, 10.19999999999998153, 1.399999999999998579 ) ) ;
#69243=DIRECTION ( 'NONE',  ( 0.000000000000000000, 1.000000000000000000, 0.000000000000000000 ) ) ;
#69244=FACE_OUTER_BOUND ( 'NONE', #131664, .T. ) ;
#69267=ORIENTED_EDGE ( 'NONE', *, *, #147671, .F. ) ;
#69276=FACE_BOUND ( 'NONE', #161351, .T. ) ;
#69277=( NAMED_UNIT ( * ) PLANE_ANGLE_UNIT ( ) SI_UNIT ( $, .RADIAN. ) );
#69283=SURFACE_SIDE_STYLE ('',( #73572 ) ) ;
#69301=CARTESIAN_POINT ( 'NONE',  ( -11.88237264505823987, 11.25677038468317015, 0.9087825512662228711 ) ) ;
#69311=CARTESIAN_POINT ( 'NONE',  ( -9.758911886679570102, 3.481540744127374243, 6.987834039733272107 ) ) ;
#69319=CARTESIAN_POINT ( 'NONE',  ( -11.33772463945043540, 12.69999999999999041, -3.600000000000078693 ) ) ;
#69331=CARTESIAN_POINT ( 'NONE',  ( 0.000000000000000000, 13.79999999999999893, 0.000000000000000000 ) ) ;
#69382=CARTESIAN_POINT ( 'NONE',  ( -10.49071307728992153, 3.038037579769635066, 7.129592439487457689 ) ) ;
#69392=( GEOMETRIC_REPRESENTATION_CONTEXT ( 3 ) GLOBAL_UNCERTAINTY_ASSIGNED_CONTEXT ( ( #26803 ) ) GLOBAL_UNIT_ASSIGNED_CONTEXT ( ( #181442, #16792, #53579 ) ) REPRESENTATION_CONTEXT ( 'NONE', 'WORKASPACE' ) );
#69412=COLOUR_RGB ( '', 0.66274510, 0.83137255, 0.94901961) ;
#69414=CARTESIAN_POINT ( 'NONE',  ( -9.523390464577085268, 15.37761368573234044, -7.301111590705639642 ) ) ;
#69419=ADVANCED_FACE ( 'NONE', ( #125853 ), #177705, .T. ) ;
#69440=B_SPLINE_CURVE_WITH_KNOTS ( 'NONE', 3,
 ( #51714, #64738, #1849, #84192, #150279, #32248 ),
 .UNSPECIFIED., .F., .F.,
 ( 4, 2, 4 ),
 ( 0.000000000000000000, 0.0003155923098472858596, 0.0006311846196945720446 ),
 .UNSPECIFIED. ) ;
#69441=CARTESIAN_POINT ( 'NONE',  ( -11.88172094500852971, 12.22000005601549688, -1.685553348215899083 ) ) ;
#69510=DIRECTION ( 'NONE',  ( -2.664535259100375697E-15, 0.000000000000000000, 1.000000000000000000 ) ) ;
#69515=EDGE_CURVE ( 'NONE', #149864, #195844, #118996, .T. ) ;
#69518=CARTESIAN_POINT ( 'NONE',  ( -11.97594889418004804, 7.449136658168690417, 0.9368335759953716479 ) ) ;
#69531=CARTESIAN_POINT ( 'NONE',  ( 9.691970092379245116, 13.38142374607198803, 8.152522038325429321 ) ) ;
#69573=ORIENTED_EDGE ( 'NONE', *, *, #7569, .F. ) ;
#69579=CARTESIAN_POINT ( 'NONE',  ( -10.19097401674926395, 4.476076320095182304, 5.708917106338025960 ) ) ;
#69630=CARTESIAN_POINT ( 'NONE',  ( 9.412040618821951199, 14.12872955391332930, -8.482482427019883531 ) ) ;
#69649=ORIENTED_EDGE ( 'NONE', *, *, #71209, .T. ) ;
#69678=EDGE_CURVE ( 'NONE', #179460, #158767, #105037, .T. ) ;
#69682=CARTESIAN_POINT ( 'NONE',  ( 11.78331023100045627, 13.79999999999999893, -1.800000000000001155 ) ) ;
#69689=CARTESIAN_POINT ( 'NONE',  ( 10.70618812723756719, 9.877096652175534786, -5.429715724251639841 ) ) ;
#69695=ORIENTED_EDGE ( 'NONE', *, *, #170541, .T. ) ;
#69702=EDGE_LOOP ( 'NONE', ( #167911, #132865, #64185, #26725, #167796, #43357, #180089, #214044 ) ) ;
#69729=CARTESIAN_POINT ( 'NONE',  ( 9.365395945939138045, 13.54490846161957585, -7.373992051513669210 ) ) ;
#69745=LINE ( 'NONE', #136921, #159989 ) ;
#69746=CARTESIAN_POINT ( 'NONE',  ( -11.52494907509597155, 8.147870201683055313, 3.187903436646419397 ) ) ;
#69749=DIRECTION ( 'NONE',  ( 1.000000000000000000, -0.000000000000000000, -0.000000000000000000 ) ) ;
#69763=LINE ( 'NONE', #84970, #173402 ) ;
#69782=CARTESIAN_POINT ( 'NONE',  ( 11.84668730067608600, 12.69999999999999929, -1.400000000000001910 ) ) ;
#69836=DIRECTION ( 'NONE',  ( 0.000000000000000000, -1.000000000000000000, 0.000000000000000000 ) ) ;
#69855=( NAMED_UNIT ( * ) PLANE_ANGLE_UNIT ( ) SI_UNIT ( $, .RADIAN. ) );
#69873=CARTESIAN_POINT ( 'NONE',  ( -15.75000000000000000, 10.19999999999999929, -3.200000000000001510 ) ) ;
#69906=CARTESIAN_POINT ( 'NONE',  ( 1.000000047849771034, 14.00000000000001066, -11.64874984998672325 ) ) ;
#69908=CARTESIAN_POINT ( 'NONE',  ( -11.14389002924298566, 7.220603907090449525, 3.549113525960188031 ) ) ;
#69936=ORIENTED_EDGE ( 'NONE', *, *, #142608, .T. ) ;
#69949=PRESENTATION_STYLE_ASSIGNMENT (( #3877 ) ) ;
#69975=EDGE_LOOP ( 'NONE', ( #71381, #83342, #198970, #92651 ) ) ;
#70005=ORIENTED_EDGE ( 'NONE', *, *, #194044, .F. ) ;
#70010=CARTESIAN_POINT ( 'NONE',  ( -10.80887392267048241, 4.296486016114100082, -4.677321330754881323 ) ) ;
#70020=CARTESIAN_POINT ( 'NONE',  ( -11.14389002924298566, 7.220603907090449525, 3.549113525960188031 ) ) ;
#70024=ORIENTED_EDGE ( 'NONE', *, *, #121129, .F. ) ;
#70026=B_SPLINE_CURVE_WITH_KNOTS ( 'NONE', 3,
 ( #178231, #194465, #111156, #95929, #98056, #177155 ),
 .UNSPECIFIED., .F., .F.,
 ( 4, 2, 4 ),
 ( 0.000000000000000000, 0.0003767643964918268649, 0.0007535287929836534046 ),
 .UNSPECIFIED. ) ;
#70027=CARTESIAN_POINT ( 'NONE',  ( 11.75000478245984503, 6.934949167590856334, -2.448457861207594455 ) ) ;
#70039=CARTESIAN_POINT ( 'NONE',  ( 9.392804560491793353, 11.17150285567701928, -6.982157407287515660 ) ) ;
#70052=CARTESIAN_POINT ( 'NONE',  ( -1.539565250226320312E-10, 15.46908218388475831, -12.00000000000000533 ) ) ;
#70054=ORIENTED_EDGE ( 'NONE', *, *, #56757, .T. ) ;
#70055=EDGE_CURVE ( 'NONE', #116248, #54188, #132726, .T. ) ;
#70056=CARTESIAN_POINT ( 'NONE',  ( -11.92619526913699879, 12.69999999999999929, -1.328859060402686199 ) ) ;
#70058=CARTESIAN_POINT ( 'NONE',  ( 0.000000000000000000, 3.481540744127368914, 0.000000000000000000 ) ) ;
#70067=DIRECTION ( 'NONE',  ( 1.000000000000000000, -0.000000000000000000, -0.000000000000000000 ) ) ;
#70095=( NAMED_UNIT ( * ) PLANE_ANGLE_UNIT ( ) SI_UNIT ( $, .RADIAN. ) );
#70112=FACE_OUTER_BOUND ( 'NONE', #94121, .T. ) ;
#70113=AXIS2_PLACEMENT_3D ( 'NONE', #202948, #104417, #108481 ) ;
#70133=VECTOR ( 'NONE', #184778, 1000.000000000000000 ) ;
#70164=( LENGTH_UNIT ( ) NAMED_UNIT ( * ) SI_UNIT ( .MILLI., .METRE. ) );
#70201=SURFACE_STYLE_USAGE ( .BOTH. , #122278 ) ;
#70204=CARTESIAN_POINT ( 'NONE',  ( -9.604686356149279902, 3.481548657788669843, -7.193747284969073341 ) ) ;
#70219=EDGE_CURVE ( 'NONE', #9929, #157346, #135577, .T. ) ;
#70223=DIRECTION ( 'NONE',  ( -0.1510067114093955887, 0.000000000000000000, 0.9885327375000383388 ) ) ;
#70239=CARTESIAN_POINT ( 'NONE',  ( 0.000000000000000000, 0.08000000000000020983, 0.000000000000000000 ) ) ;
#70247=B_SPLINE_CURVE_WITH_KNOTS ( 'NONE', 3,
 ( #64085, #96610, #112904, #79266, #46790, #113975 ),
 .UNSPECIFIED., .F., .F.,
 ( 4, 2, 4 ),
 ( 0.000000000000000000, 0.0003779448103413554443, 0.0007558896206827108886 ),
 .UNSPECIFIED. ) ;
#70248=CARTESIAN_POINT ( 'NONE',  ( -11.78331023100045627, 9.799999999999982947, 1.799999999999999600 ) ) ;
#70301=CARTESIAN_POINT ( 'NONE',  ( -10.41980074470002648, 5.020554563858687480, 5.279403930596816785 ) ) ;
#70308=DIRECTION ( 'NONE',  ( 0.000000000000000000, 0.000000000000000000, 1.000000000000000000 ) ) ;
#70309=CARTESIAN_POINT ( 'NONE',  ( -11.41381675112459959, 10.89999999999999325, 3.704697986577257129 ) ) ;
#70312=ADVANCED_FACE ( 'NONE', ( #57444 ), #105147, .F. ) ;
#70338=FACE_OUTER_BOUND ( 'NONE', #139530, .T. ) ;
#70348=DIRECTION ( 'NONE',  ( -0.000000000000000000, 1.000000000000000000, 0.000000000000000000 ) ) ;
#70367=CARTESIAN_POINT ( 'NONE',  ( -11.86145016429273191, 10.90000000000000036, 1.099999999999996980 ) ) ;
#70375=SURFACE_STYLE_FILL_AREA ( #67177 ) ;
#70383=CARTESIAN_POINT ( 'NONE',  ( -11.41381676900480713, 12.56958039977600983, -3.704697931490059215 ) ) ;
#70402=VERTEX_POINT ( 'NONE', #91030 ) ;
#70403=DIRECTION ( 'NONE',  ( 0.9632918427306580433, 0.000000000000000000, 0.2684563758389303945 ) ) ;
#70407=FILL_AREA_STYLE_COLOUR ( '', #197785 ) ;
#70414=CIRCLE ( 'NONE', #191495, 0.08000000000000014044 ) ;
#70443=CARTESIAN_POINT ( 'NONE',  ( -11.16150260363039060, 4.727604019697102977, 6.014961758122009172 ) ) ;
#70447=EDGE_CURVE ( 'NONE', #213959, #135649, #92102, .T. ) ;
#70448=CARTESIAN_POINT ( 'NONE',  ( -1.313174662617411670, 8.310476012147654856, 10.86148356754324595 ) ) ;
#70458=CARTESIAN_POINT ( 'NONE',  ( 10.62873463776380056, 11.29999999999999893, -3.200000000000001510 ) ) ;
#70461=ORIENTED_EDGE ( 'NONE', *, *, #154010, .T. ) ;
#70473=CARTESIAN_POINT ( 'NONE',  ( -9.342889098753607513, 14.55305243632841616, -7.460114340563301916 ) ) ;
#70476=EDGE_CURVE ( 'NONE', #103981, #15788, #204726, .T. ) ;
#70484=CARTESIAN_POINT ( 'NONE',  ( 11.88234649872613602, 13.75660782916751579, 0.9090484974825158160 ) ) ;
#70494=CARTESIAN_POINT ( 'NONE',  ( -10.24908409314513236, 3.786466850380959759, -6.156910069284049492 ) ) ;
#70524=CARTESIAN_POINT ( 'NONE',  ( -3.090415204605499344, 15.44821195424843019, -11.55764624973227228 ) ) ;
#70527=EDGE_LOOP ( 'NONE', ( #22245, #209205, #205261, #150083 ) ) ;
#70535=ORIENTED_EDGE ( 'NONE', *, *, #101745, .F. ) ;
#70540=FACE_BOUND ( 'NONE', #88471, .T. ) ;
#70546=CARTESIAN_POINT ( 'NONE',  ( 1.734723475976807094E-15, 14.99962766111844736, 11.68000013863625774 ) ) ;
#70552=ORIENTED_EDGE ( 'NONE', *, *, #70219, .T. ) ;
#70556=SURFACE_STYLE_FILL_AREA ( #21802 ) ;
#70560=LINE ( 'NONE', #87912, #30061 ) ;
#70585=ADVANCED_FACE ( 'NONE', ( #8680 ), #10700, .T. ) ;
#70591=CARTESIAN_POINT ( 'NONE',  ( 11.57394138716773213, 8.953477593029530723, 4.723522898263817993 ) ) ;
#70623=VECTOR ( 'NONE', #197970, 1000.000000000000000 ) ;
#70644=CARTESIAN_POINT ( 'NONE',  ( -1.349890321011286476, 8.200329036966257590, -10.79298809153609540 ) ) ;
#70698=EDGE_CURVE ( 'NONE', #35130, #124966, #76428, .T. ) ;
#70707=CARTESIAN_POINT ( 'NONE',  ( 11.92619526913699701, 13.40000000000000036, -1.328859060402686199 ) ) ;
#70743=CARTESIAN_POINT ( 'NONE',  ( -11.92619526913699524, 13.52780024161488370, 1.328859060402684866 ) ) ;
#70747=AXIS2_PLACEMENT_3D ( 'NONE', #109621, #129084, #61859 ) ;
#70754=CARTESIAN_POINT ( 'NONE',  ( 11.86239285000045740, 13.88000000000000078, -1.812080536912752837 ) ) ;
#70797=LINE ( 'NONE', #136910, #91710 ) ;
#70824=CARTESIAN_POINT ( 'NONE',  ( -11.97929049433705373, 9.719999999999998863, -0.7046979865771834106 ) ) ;
#70854=CARTESIAN_POINT ( 'NONE',  ( -9.984936468205201976, 4.580882523742140222, 6.662390435242588893 ) ) ;
#70855=CARTESIAN_POINT ( 'NONE',  ( -0.04705280706217805642, 15.48512687740116611, 11.99263203770169817 ) ) ;
#70864=CARTESIAN_POINT ( 'NONE',  ( -9.604686356149274573, 3.481540744127369802, 7.193747284969079558 ) ) ;
#70888=B_SPLINE_CURVE_WITH_KNOTS ( 'NONE', 3,
 ( #92805, #64543, #60272, #44047, #76519, #62407 ),
 .UNSPECIFIED., .F., .F.,
 ( 4, 2, 4 ),
 ( 0.000000000000000000, 0.0003844267940947831432, 0.0007688535881895662864 ),
 .UNSPECIFIED. ) ;
#70893=CARTESIAN_POINT ( 'NONE',  ( -3.796053574492273874, 15.00000000000182077, 12.24940615670316468 ) ) ;
#70897=DIRECTION ( 'NONE',  ( 0.000000000000000000, -1.000000000000000000, 0.000000000000000000 ) ) ;
#70927=SURFACE_STYLE_FILL_AREA ( #4847 ) ;
#70935=DIRECTION ( 'NONE',  ( 0.000000000000000000, 0.000000000000000000, -1.000000000000000000 ) ) ;
#70949=UNCERTAINTY_MEASURE_WITH_UNIT (LENGTH_MEASURE( 1.000000000000000082E-05 ), #108005, 'distance_accuracy_value', 'NONE');
#70950=CARTESIAN_POINT ( 'NONE',  ( 8.718062746983862965, 13.27486625357122563, -8.129070176819260141 ) ) ;
#70976=CARTESIAN_POINT ( 'NONE',  ( -9.986107380900749675, 5.615474669794299878, -5.966265754238714969 ) ) ;
#70984=CARTESIAN_POINT ( 'NONE',  ( -11.06305611892948448, 9.842384604456084318, 0.9079708613958296093 ) ) ;
#70986=VERTEX_POINT ( 'NONE', #177601 ) ;
#71005=CARTESIAN_POINT ( 'NONE',  ( 10.72102920343737331, 9.918789484241997911, 5.400078146547925506 ) ) ;
#71007=DIRECTION ( 'NONE',  ( 0.2684563758389248433, 0.000000000000000000, -0.9632918427306597087 ) ) ;
#71035=AXIS2_PLACEMENT_3D ( 'NONE', #101531, #35452, #99404 ) ;
#71038=CARTESIAN_POINT ( 'NONE',  ( 11.86239285000045740, 9.719999999999998863, -1.812080536912752837 ) ) ;
#71050=DIRECTION ( 'NONE',  ( 0.000000000000000000, -1.000000000000000000, 0.000000000000000000 ) ) ;
#71073=EDGE_LOOP ( 'NONE', ( #152504, #24156, #140977, #110899 ) ) ;
#71075=ORIENTED_EDGE ( 'NONE', *, *, #60772, .T. ) ;
#71080=CIRCLE ( 'NONE', #129952, 0.5000000000000013323 ) ;
#71081=CARTESIAN_POINT ( 'NONE',  ( -10.32224513571693869, 3.007486591634276341, -7.366906358548013678 ) ) ;
#71085=STYLED_ITEM ( 'NONE', ( #4014 ), #136888 ) ;
#71093=DIRECTION ( 'NONE',  ( -0.000000000000000000, -1.000000000000000000, -0.000000000000000000 ) ) ;
#71097=VERTEX_POINT ( 'NONE', #145130 ) ;
#71099=CARTESIAN_POINT ( 'NONE',  ( 11.48869292188783753, 7.332629663034461842, 3.321605222796156998 ) ) ;
#71123=CARTESIAN_POINT ( 'NONE',  ( -3.101842508592871361, 15.51993578035203569, -11.60075130052193337 ) ) ;
#71124=ORIENTED_EDGE ( 'NONE', *, *, #58112, .F. ) ;
#71135=EDGE_CURVE ( 'NONE', #99531, #156687, #38391, .T. ) ;
#71151=DIRECTION ( 'NONE',  ( -1.000000000000000000, 0.000000000000000000, 0.000000000000000000 ) ) ;
#71168=DIRECTION ( 'NONE',  ( -0.000000000000000000, 1.000000000000000000, 9.023263958591317418E-17 ) ) ;
#71174=ORIENTED_EDGE ( 'NONE', *, *, #113105, .F. ) ;
#71209=EDGE_CURVE ( 'NONE', #36899, #25291, #59113, .T. ) ;
#71226=ORIENTED_EDGE ( 'NONE', *, *, #74380, .T. ) ;
#71249=ORIENTED_EDGE ( 'NONE', *, *, #9318, .T. ) ;
#71252=FILL_AREA_STYLE_COLOUR ( '', #123459 ) ;
#71261=PRESENTATION_STYLE_ASSIGNMENT (( #103800 ) ) ;
#71310=STYLED_ITEM ( 'NONE', ( #153162 ), #16025 ) ;
#71328=CARTESIAN_POINT ( 'NONE',  ( 1.250000000000037526, 8.500000000000000000, -10.97907099895068583 ) ) ;
#71368=CARTESIAN_POINT ( 'NONE',  ( 9.729489633724101694, 13.21513059140455759, -8.104625967152696120 ) ) ;
#71369=CARTESIAN_POINT ( 'NONE',  ( -10.73969341588288628, 4.108126672274917013, 4.807887712954548753 ) ) ;
#71373=COLOUR_RGB ( '', 0.40784314, 0.44705882, 0.49803922) ;
#71381=ORIENTED_EDGE ( 'NONE', *, *, #57852, .T. ) ;
#71385=CARTESIAN_POINT ( 'NONE',  ( -9.305047016969982820, 15.51845925588232333, 7.450000000803896683 ) ) ;
#71412=EDGE_CURVE ( 'NONE', #207604, #185122, #150912, .T. ) ;
#71413=FILL_AREA_STYLE_COLOUR ( '', #105951 ) ;
#71437=EDGE_CURVE ( 'NONE', #61441, #198330, #18263, .T. ) ;
#71439=CARTESIAN_POINT ( 'NONE',  ( -11.94105721839851952, 11.02698343341132947, 1.187919402540718927 ) ) ;
#71482=CARTESIAN_POINT ( 'NONE',  ( -11.01135777277262129, 10.19999999999998153, 1.399999999999998579 ) ) ;
#71517=CARTESIAN_POINT ( 'NONE',  ( -9.979842676043658045, 5.589819607760296627, 5.978770845575332338 ) ) ;
#71526=ORIENTED_EDGE ( 'NONE', *, *, #155462, .T. ) ;
#71549=CARTESIAN_POINT ( 'NONE',  ( -9.585855168744716437, 14.76561575556795347, -7.219146574477996126 ) ) ;
#71560=MECHANICAL_DESIGN_GEOMETRIC_PRESENTATION_REPRESENTATION('',(#175337),#92341);
#71570=CARTESIAN_POINT ( 'NONE',  ( -9.902774762303035772, 3.558546654280230204, -6.781965751223174799 ) ) ;
#71577=CARTESIAN_POINT ( 'NONE',  ( -11.92619526913700057, 10.07218333338755301, 1.328859060402684644 ) ) ;
#71581=CARTESIAN_POINT ( 'NONE',  ( 11.41176686791169104, 13.75950803486853680, -3.404018756831829418 ) ) ;
#71592=ORIENTED_EDGE ( 'NONE', *, *, #157187, .F. ) ;
#71621=SURFACE_STYLE_USAGE ( .BOTH. , #152896 ) ;
#71637=CARTESIAN_POINT ( 'NONE',  ( -10.43059700200766216, 5.377693802073528317, 5.769666037277090709 ) ) ;
#71650=CARTESIAN_POINT ( 'NONE',  ( -11.50375155617990686, 6.427325993555151662, 3.051984382272954210 ) ) ;
#71651=CIRCLE ( 'NONE', #26670, 12.00000000000000178 ) ;
#71653=DIRECTION ( 'NONE',  ( -0.000000000000000000, -1.000000000000000000, -0.000000000000000000 ) ) ;
#71662=CARTESIAN_POINT ( 'NONE',  ( 9.728550251279687089, 13.21449840343153426, 8.106492410889076794 ) ) ;
#71678=DIRECTION ( 'NONE',  ( 1.000000000000000000, -0.000000000000000000, -0.000000000000000000 ) ) ;
#71682=STYLED_ITEM ( 'NONE', ( #121220 ), #101631 ) ;
#71689=AXIS2_PLACEMENT_3D ( 'NONE', #39876, #104882, #154688 ) ;
#71720=( LENGTH_UNIT ( ) NAMED_UNIT ( * ) SI_UNIT ( .MILLI., .METRE. ) );
#71744=( LENGTH_UNIT ( ) NAMED_UNIT ( * ) SI_UNIT ( .MILLI., .METRE. ) );
#71762=LINE ( 'NONE', #142158, #24524 ) ;
#71780=CARTESIAN_POINT ( 'NONE',  ( 11.52460864928264783, 9.719999999999982876, 3.346683403123522638 ) ) ;
#71813=CARTESIAN_POINT ( 'NONE',  ( 7.594853421417097294, 15.38634441068472469, 9.235122635145186720 ) ) ;
#71891=AXIS2_PLACEMENT_3D ( 'NONE', #33030, #486, #127428 ) ;
#71897=DIRECTION ( 'NONE',  ( 1.000000000000000000, -0.000000000000000000, -0.000000000000000000 ) ) ;
#71898=DIRECTION ( 'NONE',  ( 7.993605777301127091E-15, 0.000000000000000000, 1.000000000000000000 ) ) ;
#71902=ORIENTED_EDGE ( 'NONE', *, *, #204332, .T. ) ;
#71912=CARTESIAN_POINT ( 'NONE',  ( -11.41381675112459781, 10.19999999999998863, -3.704697986577260682 ) ) ;
#71924=CARTESIAN_POINT ( 'NONE',  ( -15.75000000000000000, 12.30000000000000071, 0.6999999999999992895 ) ) ;
#71934=DIRECTION ( 'NONE',  ( -1.000000000000000000, 0.000000000000000000, 0.000000000000000000 ) ) ;
#71942=AXIS2_PLACEMENT_3D ( 'NONE', #18437, #179897, #64008 ) ;
#72011=CARTESIAN_POINT ( 'NONE',  ( 8.961696533999443659, 14.59015583931033611, 8.974872064516899783 ) ) ;
#72042=EDGE_CURVE ( 'NONE', #204338, #48843, #42029, .T. ) ;
#72046=CARTESIAN_POINT ( 'NONE',  ( -11.31903982423144051, 5.215113036472975416, 5.710294617915439019 ) ) ;
#72048=EDGE_CURVE ( 'NONE', #120109, #211752, #3545, .T. ) ;
#72065=DIRECTION ( 'NONE',  ( 0.000000000000000000, 1.000000000000000000, 0.000000000000000000 ) ) ;
#72075=ORIENTED_EDGE ( 'NONE', *, *, #73178, .T. ) ;
#72087=FACE_OUTER_BOUND ( 'NONE', #199318, .T. ) ;
#72107=ADVANCED_FACE ( 'NONE', ( #145937 ), #112541, .T. ) ;
#72125=CARTESIAN_POINT ( 'NONE',  ( 11.97181042169640897, 9.720000000000000639, 0.8318531151397160484 ) ) ;
#72129=LINE ( 'NONE', #138236, #8290 ) ;
#72155=CARTESIAN_POINT ( 'NONE',  ( -11.73097396203126763, 4.534521666694462105, -5.066462175338618756 ) ) ;
#72164=CARTESIAN_POINT ( 'NONE',  ( -10.99931038725301846, 6.873658557531565627, -3.960823121322395224 ) ) ;
#72189=CARTESIAN_POINT ( 'NONE',  ( -9.361942704757863609, 15.42902520494341445, 7.422992708136421314 ) ) ;
#72192=CARTESIAN_POINT ( 'NONE',  ( -0.9005501737259363759, 15.44694762897113627, -11.95586207050005889 ) ) ;
#72194=ORIENTED_EDGE ( 'NONE', *, *, #29854, .T. ) ;
#72206=( NAMED_UNIT ( * ) PLANE_ANGLE_UNIT ( ) SI_UNIT ( $, .RADIAN. ) );
#72239=CARTESIAN_POINT ( 'NONE',  ( -9.857748099689047194, 5.276144085703439401, -6.217795349555793827 ) ) ;
#72256=CARTESIAN_POINT ( 'NONE',  ( -9.305047017915315521, 14.48154074413197989, -7.449999999623174496 ) ) ;
#72257=ORIENTED_EDGE ( 'NONE', *, *, #16992, .F. ) ;
#72282=EDGE_CURVE ( 'NONE', #18470, #102205, #166414, .T. ) ;
#72298=VERTEX_POINT ( 'NONE', #129741 ) ;
#72333=SURFACE_STYLE_FILL_AREA ( #88622 ) ;
#72343=COLOUR_RGB ( '', 0.40784314, 0.44705882, 0.49803922) ;
#72370=ADVANCED_FACE ( 'NONE', ( #93981 ), #95041, .F. ) ;
#72374=FACE_OUTER_BOUND ( 'NONE', #209383, .T. ) ;
#72412=ORIENTED_EDGE ( 'NONE', *, *, #211218, .T. ) ;
#72425=CARTESIAN_POINT ( 'NONE',  ( 11.48806469435255551, 13.83089772872449075, -3.468902948106704631 ) ) ;
#72427=CARTESIAN_POINT ( 'NONE',  ( -11.91826849282518630, 10.19999999999998153, 1.399999999999996581 ) ) ;
#72443=CARTESIAN_POINT ( 'NONE',  ( -11.86687215968023601, 13.60942212305781851, 1.056395335932115209 ) ) ;
#72445=CARTESIAN_POINT ( 'NONE',  ( -9.410012541129075814, 4.000000000000001776, 6.919867902370715917 ) ) ;
#72457=AXIS2_PLACEMENT_3D ( 'NONE', #70058, #6129, #203265 ) ;
#72475=CARTESIAN_POINT ( 'NONE',  ( -5.995010725448016053, 14.48115586884916439, 10.40486773299997658 ) ) ;
#72500=( LENGTH_UNIT ( ) NAMED_UNIT ( * ) SI_UNIT ( .MILLI., .METRE. ) );
#72501=DIRECTION ( 'NONE',  ( 0.000000000000000000, 0.000000000000000000, 1.000000000000000000 ) ) ;
#72514=EDGE_CURVE ( 'NONE', #83956, #180747, #207662, .T. ) ;
#72517=CARTESIAN_POINT ( 'NONE',  ( -11.97302537858628213, 11.29875989808049930, 0.8111997896468087221 ) ) ;
#72546=CARTESIAN_POINT ( 'NONE',  ( -15.75000000000000000, 12.69999999999998153, 3.599999999999999201 ) ) ;
#72561=CARTESIAN_POINT ( 'NONE',  ( 11.89835103415199313, 11.32893085832465729, -1.561208891256347986 ) ) ;
#72562=CARTESIAN_POINT ( 'NONE',  ( 9.904496571399500127, 11.51333640295184857, 6.696881809148281128 ) ) ;
#72588=CARTESIAN_POINT ( 'NONE',  ( 11.55950211276791251, 12.22000000000000064, -3.221476510067114329 ) ) ;
#72593=CARTESIAN_POINT ( 'NONE',  ( -10.24086661081948435, 5.004020940043352184, 7.476643068812830251 ) ) ;
#72597=UNCERTAINTY_MEASURE_WITH_UNIT (LENGTH_MEASURE( 1.000000000000000082E-05 ), #129868, 'distance_accuracy_value', 'NONE');
#72638=CARTESIAN_POINT ( 'NONE',  ( 11.94105722165067895, 13.52582762082958823, 1.187919369849770534 ) ) ;
#72648=DIRECTION ( 'NONE',  ( -0.000000000000000000, 1.000000000000000000, 0.000000000000000000 ) ) ;
#72653=CARTESIAN_POINT ( 'NONE',  ( 11.80251051724250821, 12.29999999999998295, 1.695257889419128361 ) ) ;
#72684=ORIENTED_EDGE ( 'NONE', *, *, #4041, .T. ) ;
#72712=( NAMED_UNIT ( * ) PLANE_ANGLE_UNIT ( ) SI_UNIT ( $, .RADIAN. ) );
#72717=FACE_OUTER_BOUND ( 'NONE', #189445, .T. ) ;
#72718=( GEOMETRIC_REPRESENTATION_CONTEXT ( 3 ) GLOBAL_UNCERTAINTY_ASSIGNED_CONTEXT ( ( #102330 ) ) GLOBAL_UNIT_ASSIGNED_CONTEXT ( ( #77369, #160759, #26479 ) ) REPRESENTATION_CONTEXT ( 'NONE', 'WORKASPACE' ) );
#72720=ORIENTED_EDGE ( 'NONE', *, *, #120570, .T. ) ;
#72722=ORIENTED_EDGE ( 'NONE', *, *, #130589, .F. ) ;
#72732=DIRECTION ( 'NONE',  ( 0.000000000000000000, 0.000000000000000000, 1.000000000000000000 ) ) ;
#72733=CARTESIAN_POINT ( 'NONE',  ( -10.99878419127389684, 6.872217442641685103, 3.961452310287494338 ) ) ;
#72745=EDGE_CURVE ( 'NONE', #97721, #140594, #118148, .T. ) ;
#72759=ORIENTED_EDGE ( 'NONE', *, *, #147648, .F. ) ;
#72761=CARTESIAN_POINT ( 'NONE',  ( -9.367496997601300279, 15.00000000000599343, 7.499999999995378808 ) ) ;
#72766=CARTESIAN_POINT ( 'NONE',  ( -11.94105721237523099, 13.40000000000000036, 1.187919463087248273 ) ) ;
#72801=CARTESIAN_POINT ( 'NONE',  ( 10.50000000000000178, 0.000000000000000000, -3.600000000000002309 ) ) ;
#72818=VERTEX_POINT ( 'NONE', #41504 ) ;
#72823=CIRCLE ( 'NONE', #41786, 12.00000000000000178 ) ;
#72839=CARTESIAN_POINT ( 'NONE',  ( 9.367381717114165340, 13.89470468729395947, 7.500780834020892129 ) ) ;
#72843=CARTESIAN_POINT ( 'NONE',  ( -11.86145016429273191, 12.59412123665269512, -1.100000000000000089 ) ) ;
#72858=ORIENTED_EDGE ( 'NONE', *, *, #80683, .T. ) ;
#72859=VERTEX_POINT ( 'NONE', #106535 ) ;
#72896=EDGE_CURVE ( 'NONE', #114917, #40498, #122836, .T. ) ;
#72905=CARTESIAN_POINT ( 'NONE',  ( -5.995690701609899698, 14.53061816844956411, -10.40446499585326912 ) ) ;
#72909=DIRECTION ( 'NONE',  ( -0.7806247498001041007, 0.000000000000000000, 0.6249999999996198596 ) ) ;
#72931=EDGE_CURVE ( 'NONE', #95365, #83422, #5824, .T. ) ;
#72959=CARTESIAN_POINT ( 'NONE',  ( -11.49966000274973155, 11.24232845564734617, -3.429881629453017222 ) ) ;
#72969=VECTOR ( 'NONE', #141236, 1000.000000000000000 ) ;
#72974=CARTESIAN_POINT ( 'NONE',  ( -11.43190902327453529, 13.65522128257853396, 3.649704988378119186 ) ) ;
#72988=CARTESIAN_POINT ( 'NONE',  ( -4.386105069058221950, 14.48107186960593573, -11.17860366124935645 ) ) ;
#72999=CARTESIAN_POINT ( 'NONE',  ( 9.681502974757661306, 4.134313097118687885, -7.090028219590201353 ) ) ;
#73005=CARTESIAN_POINT ( 'NONE',  ( 10.62873463776380056, 11.29999999999998117, 3.199999999999997957 ) ) ;
#73008=AXIS2_PLACEMENT_3D ( 'NONE', #178415, #45224, #126539 ) ;
#73012=DIRECTION ( 'NONE',  ( -0.000000000000000000, -1.000000000000000000, -0.000000000000000000 ) ) ;
#73030=B_SPLINE_CURVE_WITH_KNOTS ( 'NONE', 3,
 ( #39343, #37205, #88095, #38276, #121746, #202879, #153094, #120672, #103279, #135786, #168274, #102209, #187714, #71813, #19875, #201810, #4669, #199686 ),
 .UNSPECIFIED., .F., .F.,
 ( 4, 2, 2, 2, 2, 2, 2, 2, 4 ),
 ( -5.999999996874655676E-08, 0.0005266833517349315576, 0.001053426703469831751, 0.001580170055204731944, 0.002106913406939632354, 0.002633656758674532763, 0.003160400110409432740, 0.003687143462144333150, 0.004213886813879233993 ),
 .UNSPECIFIED. ) ;
#73079=CARTESIAN_POINT ( 'NONE',  ( 11.17802523721653252, 8.279090859639403277, 4.430515473113522340 ) ) ;
#73086=CARTESIAN_POINT ( 'NONE',  ( 7.430330521100947827, 15.94469773494527765, 9.016016616261696370 ) ) ;
#73106=CARTESIAN_POINT ( 'NONE',  ( 11.86145017031048177, 10.09418046486144505, 1.099999999999996980 ) ) ;
#73110=CARTESIAN_POINT ( 'NONE',  ( 11.01135777277262306, 12.69999999999999929, -1.400000000000001910 ) ) ;
#73119=CARTESIAN_POINT ( 'NONE',  ( -11.65681998539108655, 6.358950688113277572, -4.978640985104797245 ) ) ;
#73126=CARTESIAN_POINT ( 'NONE',  ( 10.95308175811721085, 11.29999999999998117, 1.799999999999999600 ) ) ;
#73139=ORIENTED_EDGE ( 'NONE', *, *, #77470, .F. ) ;
#73146=FACE_OUTER_BOUND ( 'NONE', #33716, .T. ) ;
#73178=EDGE_CURVE ( 'NONE', #9929, #197638, #177897, .T. ) ;
#73215=ORIENTED_EDGE ( 'NONE', *, *, #63494, .F. ) ;
#73222=VERTEX_POINT ( 'NONE', #62009 ) ;
#73224=STYLED_ITEM ( 'NONE', ( #174756 ), #74771 ) ;
#73237=CARTESIAN_POINT ( 'NONE',  ( -11.41048919578708443, 9.369870944694024928, -1.242167297096143264 ) ) ;
#73245=VERTEX_POINT ( 'NONE', #60934 ) ;
#73253=ORIENTED_EDGE ( 'NONE', *, *, #124080, .F. ) ;
#73255=DIRECTION ( 'NONE',  ( 0.000000000000000000, 0.000000000000000000, 1.000000000000000000 ) ) ;
#73256=( GEOMETRIC_REPRESENTATION_CONTEXT ( 3 ) GLOBAL_UNCERTAINTY_ASSIGNED_CONTEXT ( ( #199953 ) ) GLOBAL_UNIT_ASSIGNED_CONTEXT ( ( #135717, #67466, #82677 ) ) REPRESENTATION_CONTEXT ( 'NONE', 'WORKASPACE' ) );
#73315=CARTESIAN_POINT ( 'NONE',  ( -9.956244568750863166, 5.504298494775027528, -6.025958004757996811 ) ) ;
#73320=DIRECTION ( 'NONE',  ( 0.1510067114093955887, 0.000000000000000000, 0.9885327375000383388 ) ) ;
#73322=ORIENTED_EDGE ( 'NONE', *, *, #196415, .T. ) ;
#73332=EDGE_LOOP ( 'NONE', ( #45231, #46646, #185314, #58899 ) ) ;
#73378=DIRECTION ( 'NONE',  ( 0.7806247497997951257, 0.000000000000000000, -0.6250000000000058842 ) ) ;
#73381=CARTESIAN_POINT ( 'NONE',  ( 11.41381675112459959, 12.69999999999997087, 3.704697986577257129 ) ) ;
#73402=ORIENTED_EDGE ( 'NONE', *, *, #206408, .T. ) ;
#73412=DIRECTION ( 'NONE',  ( -0.000000000000000000, -1.000000000000000000, -0.000000000000000000 ) ) ;
#73419=CARTESIAN_POINT ( 'NONE',  ( 11.94105722165067895, 11.02582762082958467, 1.187919369849770534 ) ) ;
#73521=CARTESIAN_POINT ( 'NONE',  ( -11.96535697748088900, 13.75262667064456856, 0.9148528286453682101 ) ) ;
#73523=CARTESIAN_POINT ( 'NONE',  ( -10.64985034906098882, 4.117567600086831980, 6.884957259278849051 ) ) ;
#73529=CARTESIAN_POINT ( 'NONE',  ( -11.81907076198602802, 11.25731224596479052, -1.592066415281275349 ) ) ;
#73555=STYLED_ITEM ( 'NONE', ( #69949 ), #128748 ) ;
#73563=FILL_AREA_STYLE_COLOUR ( '', #19457 ) ;
#73572=SURFACE_STYLE_FILL_AREA ( #105033 ) ;
#73578=CARTESIAN_POINT ( 'NONE',  ( -11.78331023100045627, 11.29999999999999893, -1.800000000000001155 ) ) ;
#73579=DIRECTION ( 'NONE',  ( -0.000000000000000000, 1.000000000000000000, 0.000000000000000000 ) ) ;
#73585=CARTESIAN_POINT ( 'NONE',  ( 0.08053691275167890185, 14.48195938056239385, 11.99972973886013961 ) ) ;
#73603=CARTESIAN_POINT ( 'NONE',  ( -11.07123366811363852, 11.30000000000000071, 0.8055925608785192704 ) ) ;
#73634=VERTEX_POINT ( 'NONE', #184261 ) ;
#73637=CIRCLE ( 'NONE', #153117, 0.07999999999999933553 ) ;
#73641=CARTESIAN_POINT ( 'NONE',  ( 10.35124615470471277, 10.47624511309397199, -5.983076183620329225 ) ) ;
#73671=CARTESIAN_POINT ( 'NONE',  ( -10.80846816847880909, 4.295462489797631456, 4.678010962757586100 ) ) ;
#73690=ORIENTED_EDGE ( 'NONE', *, *, #21981, .T. ) ;
#73722=CARTESIAN_POINT ( 'NONE',  ( -8.117903383641394299, 14.55181945421660927, 8.822823676310077801 ) ) ;
#73728=CARTESIAN_POINT ( 'NONE',  ( -11.91294103507080315, 11.11460089956407060, 1.446263142085468134 ) ) ;
#73729=CARTESIAN_POINT ( 'NONE',  ( 11.89844258446855285, 12.27147310670036973, 1.560502987793273233 ) ) ;
#73730=DIRECTION ( 'NONE',  ( 0.05872483221476459958, 0.000000000000000000, 0.9982742078614211811 ) ) ;
#73737=CARTESIAN_POINT ( 'NONE',  ( 11.44789321844504215, 13.79999999999999893, -3.303298730975399167 ) ) ;
#73755=EDGE_CURVE ( 'NONE', #8935, #208480, #67973, .T. ) ;
#73757=LINE ( 'NONE', #121531, #33310 ) ;
#73793=CARTESIAN_POINT ( 'NONE',  ( -11.86239285000046095, 13.80000000000000249, -1.812080536912752837 ) ) ;
#73798=CIRCLE ( 'NONE', #97945, 11.09999999999999964 ) ;
#73808=FACE_OUTER_BOUND ( 'NONE', #36198, .T. ) ;
#73809=CARTESIAN_POINT ( 'NONE',  ( -10.71030397718323890, 6.055815897892919075, -4.668189396100475008 ) ) ;
#73812=CARTESIAN_POINT ( 'NONE',  ( -11.41108574530292863, 9.841631446223672697, 3.405883542057530633 ) ) ;
#73824=ADVANCED_FACE ( 'NONE', ( #166974 ), #121582, .T. ) ;
#73825=CARTESIAN_POINT ( 'NONE',  ( 11.89942855770814312, 12.30000000000000071, 0.6999999999999992895 ) ) ;
#73839=CARTESIAN_POINT ( 'NONE',  ( -11.01135777277262129, 10.19999999999999929, -1.400000000000001910 ) ) ;
#73844=ADVANCED_FACE ( 'NONE', ( #150732 ), #191527, .T. ) ;
#73859=CARTESIAN_POINT ( 'NONE',  ( 11.92045683181315674, 13.65275927879483042, 1.382340670101856350 ) ) ;
#73873=ORIENTED_EDGE ( 'NONE', *, *, #204859, .T. ) ;
#73875=EDGE_CURVE ( 'NONE', #45206, #106547, #106822, .T. ) ;
#73905=( LENGTH_UNIT ( ) NAMED_UNIT ( * ) SI_UNIT ( .MILLI., .METRE. ) );
#73912=SURFACE_SIDE_STYLE ('',( #157307 ) ) ;
#73926=CARTESIAN_POINT ( 'NONE',  ( 8.032759536594785033, 15.33864185422659787, 8.916444764510272236 ) ) ;
#73951=EDGE_CURVE ( 'NONE', #30509, #143616, #66096, .T. ) ;
#73964=CIRCLE ( 'NONE', #153593, 0.5000000000000006661 ) ;
#73981=EDGE_LOOP ( 'NONE', ( #78916, #171636, #187609, #203768 ) ) ;
#73985=CARTESIAN_POINT ( 'NONE',  ( -10.47476631618627252, 5.237304525980054137, 5.169966676860812349 ) ) ;
#73990=CARTESIAN_POINT ( 'NONE',  ( -1.790679264613934007, 14.55177512361720460, -11.85442263018568099 ) ) ;
#74008=ADVANCED_FACE ( 'NONE', ( #58541 ), #213657, .T. ) ;
#74029=EDGE_CURVE ( 'NONE', #19630, #97098, #44632, .T. ) ;
#74053=VERTEX_POINT ( 'NONE', #135833 ) ;
#74059=ORIENTED_EDGE ( 'NONE', *, *, #164392, .T. ) ;
#74077=CARTESIAN_POINT ( 'NONE',  ( 8.729527388974888780, 11.83892083880631851, -8.258113299037200150 ) ) ;
#74082=CARTESIAN_POINT ( 'NONE',  ( -11.41381676900480713, 10.06958039977600627, -3.704697931490059215 ) ) ;
#74086=ORIENTED_EDGE ( 'NONE', *, *, #27372, .T. ) ;
#74094=CARTESIAN_POINT ( 'NONE',  ( 9.681420877353952292, 3.865149423709351328, -7.090140323037471326 ) ) ;
#74104=FILL_AREA_STYLE_COLOUR ( '', #121171 ) ;
#74142=DIRECTION ( 'NONE',  ( -0.000000000000000000, 1.000000000000000000, 9.023263958591317418E-17 ) ) ;
#74169=AXIS2_PLACEMENT_3D ( 'NONE', #48513, #15968, #65773 ) ;
#74180=CARTESIAN_POINT ( 'NONE',  ( 8.983524160790528512, 13.98338966858836940, -7.957451094343901410 ) ) ;
#74187=CARTESIAN_POINT ( 'NONE',  ( 9.060091309786827196, 14.48005966906119646, 7.135690472246977833 ) ) ;
#74219=CARTESIAN_POINT ( 'NONE',  ( -11.38508626655161216, 5.468933214068770532, 5.576081633246319669 ) ) ;
#74226=SURFACE_STYLE_FILL_AREA ( #170643 ) ;
#74231=CIRCLE ( 'NONE', #87988, 0.07999999999999998779 ) ;
#74247=DIRECTION ( 'NONE',  ( 0.000000000000000000, 0.000000000000000000, 1.000000000000000000 ) ) ;
#74257=FACE_BOUND ( 'NONE', #9375, .T. ) ;
#74276=CARTESIAN_POINT ( 'NONE',  ( 0.000000000000000000, 13.79999999999999893, 0.000000000000000000 ) ) ;
#74294=CARTESIAN_POINT ( 'NONE',  ( -9.340724465469246951, 14.55305236562982962, -7.462818192253934946 ) ) ;
#74320=AXIS2_PLACEMENT_3D ( 'NONE', #8575, #73579, #107218 ) ;
#74333=CARTESIAN_POINT ( 'NONE',  ( -11.40891844150367618, 9.366729182080655747, 1.257950088934312705 ) ) ;
#74335=VECTOR ( 'NONE', #159243, 1000.000000000000000 ) ;
#74374=FILL_AREA_STYLE_COLOUR ( '', #146188 ) ;
#74380=EDGE_CURVE ( 'NONE', #55552, #37994, #128538, .T. ) ;
#74394=EDGE_CURVE ( 'NONE', #149864, #97098, #183783, .T. ) ;
#74404=CARTESIAN_POINT ( 'NONE',  ( 1.416786528094139630, 7.999640415717689912, 11.00953083556808387 ) ) ;
#74409=CARTESIAN_POINT ( 'NONE',  ( -11.19531657929523583, 4.806608400964729633, -5.951317567608690240 ) ) ;
#74415=EDGE_LOOP ( 'NONE', ( #191386, #131176, #176473, #202133 ) ) ;
#74418=CARTESIAN_POINT ( 'NONE',  ( 11.41157692552970460, 11.25910337086998148, 3.404533818002359880 ) ) ;
#74465=CARTESIAN_POINT ( 'NONE',  ( 9.305047017613611970, 4.518467169708414666, -7.450000000000005507 ) ) ;
#74478=CIRCLE ( 'NONE', #122960, 0.08000000000000014044 ) ;
#74483=B_SPLINE_CURVE_WITH_KNOTS ( 'NONE', 3,
 ( #29255, #110569, #174459, #12981, #140908, #211178 ),
 .UNSPECIFIED., .F., .F.,
 ( 4, 2, 4 ),
 ( 0.000000000000000000, 0.0003141553954499744054, 0.0006283107908999488109 ),
 .UNSPECIFIED. ) ;
#74486=CARTESIAN_POINT ( 'NONE',  ( 11.84668730067608244, 10.19999999999998153, 1.399999999999998357 ) ) ;
#74492=ORIENTED_EDGE ( 'NONE', *, *, #68305, .F. ) ;
#74496=FILL_AREA_STYLE_COLOUR ( '', #128632 ) ;
#74509=CARTESIAN_POINT ( 'NONE',  ( -10.91033749632886973, 4.885617943545219610, -4.996452313011736202 ) ) ;
#74514=ORIENTED_EDGE ( 'NONE', *, *, #27400, .T. ) ;
#74523=CARTESIAN_POINT ( 'NONE',  ( 9.428250952287722697, 13.54490846161957585, -7.423481931054030092 ) ) ;
#74525=LINE ( 'NONE', #40971, #88585 ) ;
#74535=LINE ( 'NONE', #9525, #54734 ) ;
#74538=AXIS2_PLACEMENT_3D ( 'NONE', #16819, #183600, #35207 ) ;
#74564=EDGE_CURVE ( 'NONE', #209385, #1117, #38323, .T. ) ;
#74586=DIRECTION ( 'NONE',  ( 0.000000000000000000, 1.000000000000000000, 0.000000000000000000 ) ) ;
#74600=CARTESIAN_POINT ( 'NONE',  ( 0.007338969819053441264, 14.55474275600908030, 11.95332390717406490 ) ) ;
#74601=( LENGTH_UNIT ( ) NAMED_UNIT ( * ) SI_UNIT ( .MILLI., .METRE. ) );
#74602=CARTESIAN_POINT ( 'NONE',  ( -11.66902918085182250, 4.335764935525111774, 5.185761432613135824 ) ) ;
#74618=VECTOR ( 'NONE', #191708, 1000.000000000000000 ) ;
#74630=CARTESIAN_POINT ( 'NONE',  ( -7.817119696385909755, 14.48014712537941406, 9.115431373065430165 ) ) ;
#74638=DIRECTION ( 'NONE',  ( -0.9486832980505139901, -0.3162277660168373861, 3.312310031615527941E-15 ) ) ;
#74642=FACE_OUTER_BOUND ( 'NONE', #16517, .T. ) ;
#74656=SURFACE_SIDE_STYLE ('',( #108291 ) ) ;
#74660=PRESENTATION_STYLE_ASSIGNMENT (( #191585 ) ) ;
#74664=EDGE_CURVE ( 'NONE', #95488, #31644, #187340, .T. ) ;
#74665=CARTESIAN_POINT ( 'NONE',  ( 0.000000000000000000, 4.000007913748540922, 1.105031132475055157E-32 ) ) ;
#74680=COLOUR_RGB ( '', 0.08235294, 0.09019608, 0.10196078) ;
#74681=SURFACE_SIDE_STYLE ('',( #8598 ) ) ;
#74682=EDGE_CURVE ( 'NONE', #114917, #45649, #88144, .T. ) ;
#74698=CARTESIAN_POINT ( 'NONE',  ( -3.492292736374302820, 15.44799614855975989, 11.44281500427524989 ) ) ;
#74745=AXIS2_PLACEMENT_3D ( 'NONE', #212815, #130597, #30906 ) ;
#74747=EDGE_LOOP ( 'NONE', ( #65021, #196594, #12735, #212142 ) ) ;
#74750=UNCERTAINTY_MEASURE_WITH_UNIT (LENGTH_MEASURE( 1.000000000000000082E-05 ), #117905, 'distance_accuracy_value', 'NONE');
#74762=CARTESIAN_POINT ( 'NONE',  ( 0.000000000000000000, 4.518459255872631530, 0.000000000000000000 ) ) ;
#74771=ADVANCED_FACE ( 'NONE', ( #171518 ), #122880, .T. ) ;
#74776=ORIENTED_EDGE ( 'NONE', *, *, #168724, .F. ) ;
#74777=( GEOMETRIC_REPRESENTATION_CONTEXT ( 3 ) GLOBAL_UNCERTAINTY_ASSIGNED_CONTEXT ( ( #154936 ) ) GLOBAL_UNIT_ASSIGNED_CONTEXT ( ( #44739, #62044, #147561 ) ) REPRESENTATION_CONTEXT ( 'NONE', 'WORKASPACE' ) );
#74781=MECHANICAL_DESIGN_GEOMETRIC_PRESENTATION_REPRESENTATION('',(#154403),#102443);
#74799=CARTESIAN_POINT ( 'NONE',  ( -5.919011879825667677, 14.55276648670623807, 10.39766294871059316 ) ) ;
#74810=CARTESIAN_POINT ( 'NONE',  ( 11.55950211276791251, 11.37999999999999901, -3.221476510067114329 ) ) ;
#74843=EDGE_CURVE ( 'NONE', #130986, #140091, #75096, .T. ) ;
#74865=PRESENTATION_STYLE_ASSIGNMENT (( #202700 ) ) ;
#74868=CARTESIAN_POINT ( 'NONE',  ( -11.87815913191694150, 13.80307820631414550, -1.708869976696544724 ) ) ;
#74882=DIRECTION ( 'NONE',  ( 0.000000000000000000, 0.000000000000000000, -1.000000000000000000 ) ) ;
#74885=CARTESIAN_POINT ( 'NONE',  ( 9.571964790107170273, 13.80900892610533859, 8.297589824372789025 ) ) ;
#74907=CARTESIAN_POINT ( 'NONE',  ( 1.333449616921242198, 8.249651149236383318, -11.01993490927446828 ) ) ;
#74978=CARTESIAN_POINT ( 'NONE',  ( -15.75000000000000000, 13.39999999999998259, 3.199999999999997957 ) ) ;
#74998=DIRECTION ( 'NONE',  ( 1.000000000000000000, -0.000000000000000000, -0.000000000000000000 ) ) ;
#75010=CARTESIAN_POINT ( 'NONE',  ( -8.752560982293191572, 13.99999996919062539, -9.356054898126068053 ) ) ;
#75052=CARTESIAN_POINT ( 'NONE',  ( -10.50659947519749693, 5.359800460605414152, -5.105385958519358169 ) ) ;
#75057=CARTESIAN_POINT ( 'NONE',  ( -7.120058533108549526, 14.48019278289345024, -9.669703555270844575 ) ) ;
#75061=CARTESIAN_POINT ( 'NONE',  ( -11.41157692552970815, 13.75910337086999746, -3.404533818002362100 ) ) ;
#75062=CARTESIAN_POINT ( 'NONE',  ( 0.000000000000000000, 14.55347103577515000, 0.000000000000000000 ) ) ;
#75065=ORIENTED_EDGE ( 'NONE', *, *, #137524, .T. ) ;
#75094=CARTESIAN_POINT ( 'NONE',  ( 11.92619526913699879, 10.19999999999999929, -1.328859060402686199 ) ) ;
#75095=EDGE_CURVE ( 'NONE', #93554, #31644, #120319, .T. ) ;
#75096=LINE ( 'NONE', #92444, #83604 ) ;
#75126=CARTESIAN_POINT ( 'NONE',  ( 9.843899315504291536, 11.91674516233577563, 6.865790592497620359 ) ) ;
#75133=CARTESIAN_POINT ( 'NONE',  ( -11.33772463945043718, 13.39999999999999147, 3.600000000000075140 ) ) ;
#75137=ORIENTED_EDGE ( 'NONE', *, *, #84764, .T. ) ;
#75144=CARTESIAN_POINT ( 'NONE',  ( 9.935043313833721967, 9.392192033208111468, 7.152792536608178153 ) ) ;
#75147=ORIENTED_EDGE ( 'NONE', *, *, #57540, .F. ) ;
#75150=EDGE_LOOP ( 'NONE', ( #154670, #57966, #79949, #66862 ) ) ;
#75152=ORIENTED_EDGE ( 'NONE', *, *, #94600, .F. ) ;
#75160=CARTESIAN_POINT ( 'NONE',  ( 9.651540038386254849, 3.878167290971859860, -7.130941910101068260 ) ) ;
#75188=CARTESIAN_POINT ( 'NONE',  ( 11.89829993707161471, 12.27080771748874177, -1.561606677374349772 ) ) ;
#75202=CARTESIAN_POINT ( 'NONE',  ( -9.898321827459618305, 15.00000000000623857, 7.924999999990495425 ) ) ;
#75205=ADVANCED_FACE ( 'NONE', ( #182025 ), #87149, .F. ) ;
#75248=CARTESIAN_POINT ( 'NONE',  ( -11.86239285000045918, 13.88000000000000078, -1.812080536912752837 ) ) ;
#75280=CARTESIAN_POINT ( 'NONE',  ( -11.58081452147585289, 6.132683923455591213, -5.154482061493088629 ) ) ;
#75283=CARTESIAN_POINT ( 'NONE',  ( -11.00605293250196226, 12.49074738641556870, -1.443095658425808114 ) ) ;
#75288=AXIS2_PLACEMENT_3D ( 'NONE', #125697, #60606, #46510 ) ;
#75316=SURFACE_STYLE_USAGE ( .BOTH. , #42844 ) ;
#75347=EDGE_CURVE ( 'NONE', #59570, #208182, #169589, .T. ) ;
#75357=SURFACE_STYLE_FILL_AREA ( #9284 ) ;
#75372=VECTOR ( 'NONE', #32811, 1000.000000000000000 ) ;
#75373=VERTEX_POINT ( 'NONE', #7060 ) ;
#75384=EDGE_CURVE ( 'NONE', #211051, #133272, #172807, .T. ) ;
#75398=CARTESIAN_POINT ( 'NONE',  ( -10.91435215633265621, 5.922423255477170301, -6.337208484649258899 ) ) ;
#75403=CARTESIAN_POINT ( 'NONE',  ( 9.276324370484291038, 11.45277045833113405, 7.615689369730119118 ) ) ;
#75415=SURFACE_STYLE_FILL_AREA ( #174010 ) ;
#75425=ORIENTED_EDGE ( 'NONE', *, *, #35088, .T. ) ;
#75469=CARTESIAN_POINT ( 'NONE',  ( -10.78926753850537423, 5.463497890167042570, -6.588879020148982413 ) ) ;
#75475=MECHANICAL_DESIGN_GEOMETRIC_PRESENTATION_REPRESENTATION('',(#206887),#186158);
#75535=CARTESIAN_POINT ( 'NONE',  ( 11.84101807917483740, 13.61021500260877559, -1.444039656437080543 ) ) ;
#75542=B_SPLINE_CURVE_WITH_KNOTS ( 'NONE', 3,
 ( #1379, #33901, #53356, #169242, #98922, #2441, #166045, #118425, #69579, #150878, #103182, #4571, #37102, #83715, #19778, #20830 ),
 .UNSPECIFIED., .F., .F.,
 ( 4, 2, 2, 2, 2, 2, 2, 4 ),
 ( 0.3501333200791456046, 0.3551713324458994903, 0.3602093448126533759, 0.3702853695461611472, 0.3803518226137216351, 0.3853850491475018791, 0.3879016624143920011, 0.3904182756812821231 ),
 .UNSPECIFIED. ) ;
#75543=DIRECTION ( 'NONE',  ( -1.000000000000000000, 0.000000000000000000, 0.000000000000000000 ) ) ;
#75552=ORIENTED_EDGE ( 'NONE', *, *, #75384, .T. ) ;
#75569=CARTESIAN_POINT ( 'NONE',  ( 11.97297122925985313, 11.29874920673088567, 0.8121202983519475449 ) ) ;
#75570=CARTESIAN_POINT ( 'NONE',  ( 8.790438134619869004, 13.29428800202395955, -8.101059483297389008 ) ) ;
#75588=CARTESIAN_POINT ( 'NONE',  ( 9.244366848620945376, 14.19092405134642298, -7.651760635101037877 ) ) ;
#75597=CARTESIAN_POINT ( 'NONE',  ( 11.44779963594995564, 10.19999999999997442, 3.600000000000075140 ) ) ;
#75599=EDGE_CURVE ( 'NONE', #139393, #175615, #10922, .T. ) ;
#75641=PRESENTATION_STYLE_ASSIGNMENT (( #155828 ) ) ;
#75644=CARTESIAN_POINT ( 'NONE',  ( 9.367496997597598352, 4.518459255872631530, 7.500000000000000000 ) ) ;
#75665=CARTESIAN_POINT ( 'NONE',  ( 9.681426354872456841, 13.43812210156014508, -8.165041025796162089 ) ) ;
#75666=CARTESIAN_POINT ( 'NONE',  ( -10.76112648294250462, 4.189587671054875173, 6.709456861673908534 ) ) ;
#75672=CARTESIAN_POINT ( 'NONE',  ( -11.78331023100045627, 11.29999999999999893, -1.800000000000001155 ) ) ;
#75689=CARTESIAN_POINT ( 'NONE',  ( 9.406473561382165727, 4.446947634372959257, -7.380697597781017194 ) ) ;
#75697=ORIENTED_EDGE ( 'NONE', *, *, #147938, .F. ) ;
#75704=CARTESIAN_POINT ( 'NONE',  ( 11.94655611907589865, 11.15200944546904083, -1.134828163062138628 ) ) ;
#75712=DIRECTION ( 'NONE',  ( 0.000000000000000000, 1.804652791718263484E-16, -1.000000000000000000 ) ) ;
#75722=( NAMED_UNIT ( * ) PLANE_ANGLE_UNIT ( ) SI_UNIT ( $, .RADIAN. ) );
#75728=CIRCLE ( 'NONE', #51622, 0.08000000000000020983 ) ;
#75732=CARTESIAN_POINT ( 'NONE',  ( -10.56357071321730778, 4.163828001052541694, 5.599134949294604979 ) ) ;
#75743=FILL_AREA_STYLE_COLOUR ( '', #205041 ) ;
#75762=DIRECTION ( 'NONE',  ( 1.000000000000000000, -0.000000000000000000, -0.000000000000000000 ) ) ;
#75763=( BOUNDED_SURFACE ( )  B_SPLINE_SURFACE ( 3, 2, ( 
 ( #109535, #23923, #175539 ),
 ( #5518, #90028, #147299 ),
 ( #81218, #64951, #15130 ),
 ( #112726, #127945, #178736 ),
 ( #27129, #95371, #111658 ),
 ( #31414, #160342, #79080 ) ),
 .UNSPECIFIED., .F., .F., .F. ) 
 B_SPLINE_SURFACE_WITH_KNOTS ( ( 4, 2, 4 ),
 ( 3, 3 ),
 ( 0.000000000000000000, 0.0003766405729503176413, 0.0007532811459006352826 ),
 ( 0.000000000000000000, 1.000000000000000000 ),
 .UNSPECIFIED. ) 
 GEOMETRIC_REPRESENTATION_ITEM ( )  RATIONAL_B_SPLINE_SURFACE ( (
 ( 1.000000000000000000, 0.7071067811865551223, 1.000000000000000000),
 ( 1.000000000000000000, 0.7211294902953071517, 1.000000000000000000),
 ( 1.000000000000000000, 0.7311181975231312302, 1.000000000000000000),
 ( 1.000000000000000000, 0.7429553055060466038, 1.000000000000000000),
 ( 1.000000000000000000, 0.7451698531058986719, 1.000000000000000000),
 ( 1.000000000000000000, 0.7452309222763021657, 1.000000000000000000) ) ) 
 REPRESENTATION_ITEM ( '' )  SURFACE ( )  );
#75775=( NAMED_UNIT ( * ) SI_UNIT ( $, .STERADIAN. ) SOLID_ANGLE_UNIT ( ) );
#75778=CARTESIAN_POINT ( 'NONE',  ( 11.95134215679451373, 7.565930823690049323, -0.2097427604813490720 ) ) ;
#75806=CARTESIAN_POINT ( 'NONE',  ( -0.08011315927826534455, 15.51845603285927488, 11.99973258290723699 ) ) ;
#75807=CARTESIAN_POINT ( 'NONE',  ( -10.37901820579008039, 4.889546506944066451, 5.358714317323078014 ) ) ;
#75813=FACE_OUTER_BOUND ( 'NONE', #7587, .T. ) ;
#75816=ORIENTED_EDGE ( 'NONE', *, *, #117680, .F. ) ;
#75824=( BOUNDED_CURVE ( )  B_SPLINE_CURVE ( 3, ( #117464, #1480, #65423, #132618 ),
 .UNSPECIFIED., .F., .T. ) 
 B_SPLINE_CURVE_WITH_KNOTS ( ( 4, 4 ),
 ( 4.845169979278623806, 4.852380668139161912 ),
 .UNSPECIFIED. ) 
 CURVE ( )  GEOMETRIC_REPRESENTATION_ITEM ( )  RATIONAL_B_SPLINE_CURVE ( ( 1.000000000000000000, 0.9999956671685397147, 0.9999956671685397147, 1.000000000000000000 ) ) 
 REPRESENTATION_ITEM ( '' )  );
#75826=CARTESIAN_POINT ( 'NONE',  ( -11.55950211276791428, 9.719999999999982876, 3.221476510067114329 ) ) ;
#75871=CARTESIAN_POINT ( 'NONE',  ( 11.89197415570408900, 13.79999999999999716, 0.8055989572471804472 ) ) ;
#75893=DIRECTION ( 'NONE',  ( 0.000000000000000000, 1.000000000000000000, 0.000000000000000000 ) ) ;
#75902=DIRECTION ( 'NONE',  ( 0.000000000000000000, 0.000000000000000000, -1.000000000000000000 ) ) ;
#75910=CARTESIAN_POINT ( 'NONE',  ( -1.734723475976807094E-15, 4.518467169708413778, -12.00000000000000178 ) ) ;
#75921=VERTEX_POINT ( 'NONE', #212742 ) ;
#75926=CARTESIAN_POINT ( 'NONE',  ( 9.367496997597594799, 3.481548657788670731, -7.500000000000007105 ) ) ;
#75932=ORIENTED_EDGE ( 'NONE', *, *, #113105, .T. ) ;
#75939=( GEOMETRIC_REPRESENTATION_CONTEXT ( 3 ) GLOBAL_UNCERTAINTY_ASSIGNED_CONTEXT ( ( #94223 ) ) GLOBAL_UNIT_ASSIGNED_CONTEXT ( ( #192647, #78899, #14949 ) ) REPRESENTATION_CONTEXT ( 'NONE', 'WORKASPACE' ) );
#75947=DIRECTION ( 'NONE',  ( -0.2684563758389304500, 0.000000000000000000, -0.9632918427306581544 ) ) ;
#75952=DIRECTION ( 'NONE',  ( -0.000000000000000000, -1.000000000000000000, 0.000000000000000000 ) ) ;
#75959=CARTESIAN_POINT ( 'NONE',  ( 11.97302537858650773, 12.30124010191982720, 0.8111997896468311486 ) ) ;
#75975=CARTESIAN_POINT ( 'NONE',  ( -10.51596412982177853, 12.48659081731577380, -3.553961965504329967 ) ) ;
#75992=CARTESIAN_POINT ( 'NONE',  ( 8.216319294035601573, 14.20048435439411882, 8.685543064379698919 ) ) ;
#75998=DIRECTION ( 'NONE',  ( 0.000000000000000000, 0.000000000000000000, 1.000000000000000000 ) ) ;
#76003=ORIENTED_EDGE ( 'NONE', *, *, #107910, .F. ) ;
#76035=EDGE_CURVE ( 'NONE', #86850, #37826, #44950, .T. ) ;
#76076=CARTESIAN_POINT ( 'NONE',  ( 10.50000000000000178, 12.69999999999999929, -3.600000000000000977 ) ) ;
#76100=CARTESIAN_POINT ( 'NONE',  ( -10.60583023524544544, 4.240113626697339377, 5.518324045435343272 ) ) ;
#76114=CARTESIAN_POINT ( 'NONE',  ( 11.84100621633422179, 13.61041574223334649, 1.444132586618105174 ) ) ;
#76115=DIRECTION ( 'NONE',  ( -0.000000000000000000, 1.000000000000000000, -0.000000000000000000 ) ) ;
#76119=ADVANCED_FACE ( 'NONE', ( #10279 ), #192221, .F. ) ;
#76129=CIRCLE ( 'NONE', #148799, 12.00000000000000178 ) ;
#76149=ORIENTED_EDGE ( 'NONE', *, *, #148914, .T. ) ;
#76173=CARTESIAN_POINT ( 'NONE',  ( -11.48767021851168124, 11.33004227463830738, -3.470194894594655910 ) ) ;
#76178=ORIENTED_EDGE ( 'NONE', *, *, #199418, .T. ) ;
#76184=CARTESIAN_POINT ( 'NONE',  ( 11.29023325225217533, 8.870178701907233787, -4.083937312904004635 ) ) ;
#76192=SURFACE_STYLE_FILL_AREA ( #10117 ) ;
#76201=CARTESIAN_POINT ( 'NONE',  ( 8.806674072578200452, 13.38234123322611602, 7.683694639725048958 ) ) ;
#76215=ADVANCED_FACE ( 'NONE', ( #14535 ), #28415, .T. ) ;
#76243=DIRECTION ( 'NONE',  ( 0.000000000000000000, 1.000000000000000000, 0.000000000000000000 ) ) ;
#76283=CARTESIAN_POINT ( 'NONE',  ( -11.01135777277262129, 0.000000000000000000, 1.399999999999998579 ) ) ;
#76303=CARTESIAN_POINT ( 'NONE',  ( -10.96643471353314503, 6.136560960136473675, 4.903152034993116359 ) ) ;
#76309=CARTESIAN_POINT ( 'NONE',  ( 7.320800350271525758, 15.00158243878686726, 10.35317514277968343 ) ) ;
#76342=CARTESIAN_POINT ( 'NONE',  ( -12.15542830485202153, 9.245334104615434256, -2.757920875862237775 ) ) ;
#76344=CARTESIAN_POINT ( 'NONE',  ( -11.01135777277262484, 12.59501355085106233, -1.400000000000001021 ) ) ;
#76346=( BOUNDED_CURVE ( )  B_SPLINE_CURVE ( 3, ( #206515, #74404, #188135, #124305 ),
 .UNSPECIFIED., .F., .T. ) 
 B_SPLINE_CURVE_WITH_KNOTS ( ( 4, 4 ),
 ( 4.576839133004759752, 4.599536981099443977 ),
 .UNSPECIFIED. ) 
 CURVE ( )  GEOMETRIC_REPRESENTATION_ITEM ( )  RATIONAL_B_SPLINE_CURVE ( ( 1.000000000000000000, 0.9999570677684579412, 0.9999570677684579412, 1.000000000000000000 ) ) 
 REPRESENTATION_ITEM ( '' )  );
#76366=CARTESIAN_POINT ( 'NONE',  ( 11.15514917209906365, 9.121482996107461716, -4.437425157417320243 ) ) ;
#76411=CARTESIAN_POINT ( 'NONE',  ( -11.07599756093943988, 5.827638661946632936, 4.513623486852267774 ) ) ;
#76426=( LENGTH_UNIT ( ) NAMED_UNIT ( * ) SI_UNIT ( .MILLI., .METRE. ) );
#76428=CIRCLE ( 'NONE', #180185, 11.92000000000000171 ) ;
#76439=EDGE_CURVE ( 'NONE', #136644, #169237, #80365, .T. ) ;
#76454=CARTESIAN_POINT ( 'NONE',  ( -10.93392920578941485, 5.995216197940580471, 6.296921006145307587 ) ) ;
#76519=CARTESIAN_POINT ( 'NONE',  ( -11.52463353791760348, 13.88000000000000256, -3.346594096177641475 ) ) ;
#76523=EDGE_CURVE ( 'NONE', #129981, #1117, #66402, .T. ) ;
#76525=CARTESIAN_POINT ( 'NONE',  ( -10.77321989194975416, 5.423924896255240213, -6.620653902763565135 ) ) ;
#76533=CARTESIAN_POINT ( 'NONE',  ( 11.33772463945037323, 11.00902469614648815, 3.599999999999998757 ) ) ;
#76577=CARTESIAN_POINT ( 'NONE',  ( -9.540655113774951346, 3.481548657788669843, -7.145788969735948015 ) ) ;
#76593=CARTESIAN_POINT ( 'NONE',  ( 9.444983200488291430, 11.02393056587705367, 7.408221049322018636 ) ) ;
#76619=ORIENTED_EDGE ( 'NONE', *, *, #201250, .T. ) ;
#76622=CARTESIAN_POINT ( 'NONE',  ( 11.04986227068298277, 13.60939997844336169, -1.056429153205399984 ) ) ;
#76623=CARTESIAN_POINT ( 'NONE',  ( 11.97929049433705373, 11.37999999999999901, 0.7046979865771804130 ) ) ;
#76624=CARTESIAN_POINT ( 'NONE',  ( 8.889571721160198337, 12.82189538422087693, -7.992081087592324273 ) ) ;
#76627=CARTESIAN_POINT ( 'NONE',  ( -9.604686356149278126, 4.469082183884762749, 7.193747284969080447 ) ) ;
#76631=CARTESIAN_POINT ( 'NONE',  ( -9.549101787676201880, 14.79376669176756387, -7.267872539543604127 ) ) ;
#76644=FILL_AREA_STYLE ('',( #7359 ) ) ;
#76653=DIRECTION ( 'NONE',  ( 0.000000000000000000, -1.000000000000000000, -9.023263958591317418E-17 ) ) ;
#76665=CARTESIAN_POINT ( 'NONE',  ( 9.368660915953467949, 13.69988896159187242, -7.498844331761238102 ) ) ;
#76685=EDGE_LOOP ( 'NONE', ( #71592, #33114, #1159, #105295, #60180 ) ) ;
#76691=( LENGTH_UNIT ( ) NAMED_UNIT ( * ) SI_UNIT ( .MILLI., .METRE. ) );
#76710=CARTESIAN_POINT ( 'NONE',  ( 11.92619526248521034, 13.52744613914163985, 1.328859120100916558 ) ) ;
#76712=VERTEX_POINT ( 'NONE', #143012 ) ;
#76715=CARTESIAN_POINT ( 'NONE',  ( 10.25134988613697828, 12.94137091940703499, -7.028098868429560220 ) ) ;
#76762=COLOUR_RGB ( '', 0.09019608, 0.27058824, 0.51372549) ;
#76768=CARTESIAN_POINT ( 'NONE',  ( -4.369225125877626681, 14.55265043571744421, 11.13763656838536953 ) ) ;
#76770=DIRECTION ( 'NONE',  ( 1.000000000000000000, -0.000000000000000000, -0.000000000000000000 ) ) ;
#76775=( NAMED_UNIT ( * ) SI_UNIT ( $, .STERADIAN. ) SOLID_ANGLE_UNIT ( ) );
#76787=VERTEX_POINT ( 'NONE', #57459 ) ;
#76805=EDGE_CURVE ( 'NONE', #187025, #140333, #38771, .T. ) ;
#76817=CARTESIAN_POINT ( 'NONE',  ( -11.92619526913699879, 10.19999999999999929, -1.328859060402686199 ) ) ;
#76823=ORIENTED_EDGE ( 'NONE', *, *, #150960, .F. ) ;
#76828=UNCERTAINTY_MEASURE_WITH_UNIT (LENGTH_MEASURE( 1.000000000000000082E-05 ), #12589, 'distance_accuracy_value', 'NONE');
#76830=CARTESIAN_POINT ( 'NONE',  ( 9.527355378288246968, 12.67468934319733442, 7.222524825386243741 ) ) ;
#76833=EDGE_CURVE ( 'NONE', #80409, #120419, #201384, .T. ) ;
#76841=ORIENTED_EDGE ( 'NONE', *, *, #98624, .T. ) ;
#76857=CARTESIAN_POINT ( 'NONE',  ( 11.52463353791759992, 12.22000000000000242, -3.346594096177641475 ) ) ;
#76858=DIRECTION ( 'NONE',  ( -0.000000000000000000, 1.000000000000000000, 0.000000000000000000 ) ) ;
#76945=MECHANICAL_DESIGN_GEOMETRIC_PRESENTATION_REPRESENTATION('',(#21717),#201543);
#76954=CARTESIAN_POINT ( 'NONE',  ( -11.84668730067608600, 10.90000000000000036, -1.400000000000001910 ) ) ;
#76979=CARTESIAN_POINT ( 'NONE',  ( 11.55950211276791251, 9.799999999999998934, -3.221476510067115662 ) ) ;
#77005=DIRECTION ( 'NONE',  ( 0.9885327375000381167, 0.000000000000000000, -0.1510067114093955609 ) ) ;
#77020=CARTESIAN_POINT ( 'NONE',  ( 1.500000000000065503, 7.750000000000000000, -10.99818166789400919 ) ) ;
#77032=TOROIDAL_SURFACE ( 'NONE', #153247, 11.92000000000000171, 0.08000000000000000167 ) ;
#77047=ORIENTED_EDGE ( 'NONE', *, *, #117837, .T. ) ;
#77058=ORIENTED_EDGE ( 'NONE', *, *, #39139, .F. ) ;
#77098=AXIS2_PLACEMENT_3D ( 'NONE', #57269, #74586, #140689 ) ;
#77103=ORIENTED_EDGE ( 'NONE', *, *, #188457, .T. ) ;
#77116=COLOUR_RGB ( '', 0.40784314, 0.44705882, 0.49803922) ;
#77125=UNCERTAINTY_MEASURE_WITH_UNIT (LENGTH_MEASURE( 1.000000000000000082E-05 ), #69234, 'distance_accuracy_value', 'NONE');
#77131=CARTESIAN_POINT ( 'NONE',  ( 11.92619526913699524, 10.07219975838508219, 1.328859060402684644 ) ) ;
#77174=CARTESIAN_POINT ( 'NONE',  ( -10.60630588279735242, 5.715763139788331948, 4.896273837757428637 ) ) ;
#77178=CARTESIAN_POINT ( 'NONE',  ( -4.386105057119274342, 14.48107186952841374, -11.17860366588836563 ) ) ;
#77186=TOROIDAL_SURFACE ( 'NONE', #115442, 11.18000000000000149, 0.08000000000000000167 ) ;
#77196=SURFACE_SIDE_STYLE ('',( #128187 ) ) ;
#77209=ORIENTED_EDGE ( 'NONE', *, *, #80428, .T. ) ;
#77269=CARTESIAN_POINT ( 'NONE',  ( 11.70309665408334254, 6.967153772763111874, -4.128557813934621734 ) ) ;
#77273=ORIENTED_EDGE ( 'NONE', *, *, #73755, .T. ) ;
#77303=CARTESIAN_POINT ( 'NONE',  ( -11.94980361723156292, 11.00238056585436119, -1.099999926404080064 ) ) ;
#77329=CARTESIAN_POINT ( 'NONE',  ( -11.48243876534946217, 13.79999999999998295, 3.199999999999997957 ) ) ;
#77341=CARTESIAN_POINT ( 'NONE',  ( 11.04986239659823433, 9.990607685143002570, -1.056426191432995765 ) ) ;
#77358=CARTESIAN_POINT ( 'NONE',  ( 11.48243876534946217, 9.719999999999982876, 3.199999999999997957 ) ) ;
#77360=SURFACE_SIDE_STYLE ('',( #159679 ) ) ;
#77369=( LENGTH_UNIT ( ) NAMED_UNIT ( * ) SI_UNIT ( .MILLI., .METRE. ) );
#77372=CARTESIAN_POINT ( 'NONE',  ( -11.43204722947019825, 12.44407245973826193, -3.649275849833183649 ) ) ;
#77375=CARTESIAN_POINT ( 'NONE',  ( 8.210650312929315575, 13.38009969560112999, 8.580131456927484024 ) ) ;
#77381=VERTEX_POINT ( 'NONE', #30293 ) ;
#77408=CARTESIAN_POINT ( 'NONE',  ( -11.19364298753552411, 5.612864353363596237, -3.868560769348357464 ) ) ;
#77413=COLOUR_RGB ( '', 0.31764706, 0.68627451, 0.89019608) ;
#77433=EDGE_LOOP ( 'NONE', ( #115908, #154526, #62329, #65730 ) ) ;
#77434=CARTESIAN_POINT ( 'NONE',  ( 11.95224097337929337, 7.720691929998547920, -1.091235320809971210 ) ) ;
#77449=EDGE_CURVE ( 'NONE', #52465, #121123, #34241, .T. ) ;
#77470=EDGE_CURVE ( 'NONE', #152468, #174627, #97437, .T. ) ;
#77482=DIRECTION ( 'NONE',  ( -0.000000000000000000, 1.000000000000000000, -0.000000000000000000 ) ) ;
#77487=CARTESIAN_POINT ( 'NONE',  ( 11.97929049433705373, 11.37999999999999901, 0.7046979865771783036 ) ) ;
#77503=VERTEX_POINT ( 'NONE', #161366 ) ;
#77511=CARTESIAN_POINT ( 'NONE',  ( -9.348561386899501002, 3.999985931113709814, -7.001914024221969512 ) ) ;
#77522=CARTESIAN_POINT ( 'NONE',  ( -10.47476534206535170, 5.237283261923990629, -5.169982392003922733 ) ) ;
#77548=ORIENTED_EDGE ( 'NONE', *, *, #110539, .T. ) ;
#77551=CARTESIAN_POINT ( 'NONE',  ( -0.9045775026450960654, 15.44695887967888304, 11.95520906865927380 ) ) ;
#77562=CIRCLE ( 'NONE', #191649, 0.08000000000000020983 ) ;
#77599=ORIENTED_EDGE ( 'NONE', *, *, #90947, .T. ) ;
#77622=CIRCLE ( 'NONE', #63863, 0.07999999999999998779 ) ;
#77635=UNCERTAINTY_MEASURE_WITH_UNIT (LENGTH_MEASURE( 1.000000000000000082E-05 ), #87687, 'distance_accuracy_value', 'NONE');
#77651=ORIENTED_EDGE ( 'NONE', *, *, #34941, .F. ) ;
#77659=CARTESIAN_POINT ( 'NONE',  ( 1.466069532605751007E-15, 14.48154074412737558, 12.00000000000000178 ) ) ;
#77692=CARTESIAN_POINT ( 'NONE',  ( 11.96209379583854293, 11.32792940594236519, 0.9572398070798464609 ) ) ;
#77693=PLANE ( 'NONE',  #18427 ) ;
#77696=CARTESIAN_POINT ( 'NONE',  ( -9.569358774149648639, 4.446947634372959257, 7.167287524840459945 ) ) ;
#77701=( BOUNDED_SURFACE ( )  B_SPLINE_SURFACE ( 3, 2, ( 
 ( #140156, #206180, #190990 ),
 ( #5822, #138006, #57809 ),
 ( #142299, #43720, #58877 ),
 ( #173724, #123970, #72974 ),
 ( #91403, #157463, #9058 ),
 ( #75133, #125033, #42655 ) ),
 .UNSPECIFIED., .F., .F., .T. ) 
 B_SPLINE_SURFACE_WITH_KNOTS ( ( 4, 2, 4 ),
 ( 3, 3 ),
 ( 0.000000000000000000, 0.0003831416164015014384, 0.0007662832328030028768 ),
 ( 0.000000000000000000, 1.000000000000000000 ),
 .UNSPECIFIED. ) 
 GEOMETRIC_REPRESENTATION_ITEM ( )  RATIONAL_B_SPLINE_SURFACE ( (
 ( 1.000000000000000000, 0.7071067811865475727, 1.000000000000000000),
 ( 1.000000000000000000, 0.6829713513656885393, 1.000000000000000000),
 ( 1.000000000000000000, 0.6534833722367636710, 1.000000000000000000),
 ( 1.000000000000000000, 0.6054027484667212633, 1.000000000000000000),
 ( 1.000000000000000000, 0.5875453974411548597, 1.000000000000000000),
 ( 1.000000000000000000, 0.5879095031487528988, 1.000000000000000000) ) ) 
 REPRESENTATION_ITEM ( '' )  SURFACE ( )  );
#77703=CARTESIAN_POINT ( 'NONE',  ( 0.000000000000000000, 14.48154074412737025, -11.92000000000000171 ) ) ;
#77713=VECTOR ( 'NONE', #39211, 1000.000000000000000 ) ;
#77718=B_SPLINE_CURVE_WITH_KNOTS ( 'NONE', 3,
 ( #971, #82242, #50819, #49753, #201306, #148333 ),
 .UNSPECIFIED., .F., .F.,
 ( 4, 2, 4 ),
 ( 0.000000000000000000, 0.0003258677429877278493, 0.0006517354859754556987 ),
 .UNSPECIFIED. ) ;
#77734=CARTESIAN_POINT ( 'NONE',  ( 7.986935577548707421, 15.27020226968796734, -8.898074972344000244 ) ) ;
#77746=EDGE_CURVE ( 'NONE', #29424, #76787, #104483, .T. ) ;
#77754=ORIENTED_EDGE ( 'NONE', *, *, #94349, .F. ) ;
#77786=CARTESIAN_POINT ( 'NONE',  ( 9.709990956404908502, 13.29774486163194958, 8.129890332494706939 ) ) ;
#77787=CARTESIAN_POINT ( 'NONE',  ( -10.33392256004288079, 4.765625372279607141, 5.445010993851796322 ) ) ;
#77792=B_SPLINE_CURVE_WITH_KNOTS ( 'NONE', 3,
 ( #35067, #34013, #84899, #83824, #2550, #70754 ),
 .UNSPECIFIED., .F., .F.,
 ( 4, 2, 4 ),
 ( 0.000000000000000000, 0.0003778774010236168076, 0.0007557548020472336153 ),
 .UNSPECIFIED. ) ;
#77815=CARTESIAN_POINT ( 'NONE',  ( -10.10707714348148301, 4.359868340440408829, -5.857196085253971063 ) ) ;
#77840=CARTESIAN_POINT ( 'NONE',  ( -11.84668730067608600, 10.90000000000000036, -1.400000000000001910 ) ) ;
#77847=CARTESIAN_POINT ( 'NONE',  ( 0.000000000000000000, 15.51887838114830132, 0.000000000000000000 ) ) ;
#77855=CARTESIAN_POINT ( 'NONE',  ( -10.84254087577866521, 4.919568073182916557, 5.035408296252067650 ) ) ;
#77865=FACE_OUTER_BOUND ( 'NONE', #162813, .T. ) ;
#77868=ADVANCED_FACE ( 'NONE', ( #69148 ), #201282, .T. ) ;
#77923=MECHANICAL_DESIGN_GEOMETRIC_PRESENTATION_REPRESENTATION('',(#71085),#88290);
#77925=CARTESIAN_POINT ( 'NONE',  ( -9.367496997601305608, 14.48154074412967596, 7.499999999995371702 ) ) ;
#77951=VERTEX_POINT ( 'NONE', #23616 ) ;
#77974=CARTESIAN_POINT ( 'NONE',  ( 11.48243876534946217, 12.22000000000000064, -3.200000000000001510 ) ) ;
#78017=CARTESIAN_POINT ( 'NONE',  ( 11.49966000274960898, 12.35767154435270498, -3.429881629453144232 ) ) ;
#78028=DIRECTION ( 'NONE',  ( -0.000000000000000000, -1.000000000000000000, -0.000000000000000000 ) ) ;
#78042=DIRECTION ( 'NONE',  ( 0.000000000000000000, 0.000000000000000000, -1.000000000000000000 ) ) ;
#78048=ORIENTED_EDGE ( 'NONE', *, *, #208749, .F. ) ;
#78051=CARTESIAN_POINT ( 'NONE',  ( 10.95308175811721085, 12.29999999999998295, 1.799999999999999600 ) ) ;
#78059=CIRCLE ( 'NONE', #19130, 11.92000000000000171 ) ;
#78079=CARTESIAN_POINT ( 'NONE',  ( -11.97929049433705551, 9.799999999999998934, -0.7046979865771820783 ) ) ;
#78095=CARTESIAN_POINT ( 'NONE',  ( -11.48767021851168124, 13.83004227463830738, -3.470194894594655910 ) ) ;
#78116=( NAMED_UNIT ( * ) PLANE_ANGLE_UNIT ( ) SI_UNIT ( $, .RADIAN. ) );
#78121=ORIENTED_EDGE ( 'NONE', *, *, #81005, .F. ) ;
#78129=EDGE_CURVE ( 'NONE', #55552, #182455, #142698, .T. ) ;
#78130=ORIENTED_EDGE ( 'NONE', *, *, #137433, .T. ) ;
#78135=CARTESIAN_POINT ( 'NONE',  ( 11.48806469435255551, 12.26910227127549646, 3.468902948106700190 ) ) ;
#78159=FILL_AREA_STYLE ('',( #147443 ) ) ;
#78165=DIRECTION ( 'NONE',  ( 0.000000000000000000, 1.000000000000000000, 0.000000000000000000 ) ) ;
#78170=VECTOR ( 'NONE', #179365, 1000.000000000000000 ) ;
#78181=UNCERTAINTY_MEASURE_WITH_UNIT (LENGTH_MEASURE( 1.000000000000000082E-05 ), #23589, 'distance_accuracy_value', 'NONE');
#78183=CARTESIAN_POINT ( 'NONE',  ( -11.33772463945036968, 19.00000000000000000, -3.680000000000002824 ) ) ;
#78193=VERTEX_POINT ( 'NONE', #59331 ) ;
#78222=ORIENTED_EDGE ( 'NONE', *, *, #126323, .F. ) ;
#78244=ORIENTED_EDGE ( 'NONE', *, *, #85559, .F. ) ;
#78291=COLOUR_RGB ( '', 0.40784314, 0.44705882, 0.49803922) ;
#78305=CARTESIAN_POINT ( 'NONE',  ( 11.97929049433705373, 9.719999999999998863, -0.7046979865771834106 ) ) ;
#78314=CARTESIAN_POINT ( 'NONE',  ( 9.980677382359758099, 11.54895643263491145, -6.667707585166605888 ) ) ;
#78325=FILL_AREA_STYLE_COLOUR ( '', #184839 ) ;
#78328=ORIENTED_EDGE ( 'NONE', *, *, #6305, .F. ) ;
#78336=CARTESIAN_POINT ( 'NONE',  ( 8.726851280726220850, 11.84099526508991218, 8.258125689521147450 ) ) ;
#78348=CARTESIAN_POINT ( 'NONE',  ( 0.000000000000000000, 9.719999999999998863, 0.000000000000000000 ) ) ;
#78355=AXIS2_PLACEMENT_3D ( 'NONE', #211494, #13306, #79379 ) ;
#78356=( BOUNDED_CURVE ( )  B_SPLINE_CURVE ( 3, ( #155970, #123558, #205764, #41168 ),
 .UNSPECIFIED., .F., .T. ) 
 B_SPLINE_CURVE_WITH_KNOTS ( ( 4, 4 ),
 ( 4.845169979278624695, 4.852380668139161912 ),
 .UNSPECIFIED. ) 
 CURVE ( )  GEOMETRIC_REPRESENTATION_ITEM ( )  RATIONAL_B_SPLINE_CURVE ( ( 1.000000000000000000, 0.9999956671685397147, 0.9999956671685397147, 1.000000000000000000 ) ) 
 REPRESENTATION_ITEM ( '' )  );
#78366=CARTESIAN_POINT ( 'NONE',  ( -11.95359438121989371, 11.10421899708699733, -1.059536798430483984 ) ) ;
#78383=MECHANICAL_DESIGN_GEOMETRIC_PRESENTATION_REPRESENTATION('',(#47337),#185664);
#78394=CARTESIAN_POINT ( 'NONE',  ( 1.050790385995002740, 15.00000000000000355, 12.64745918785790302 ) ) ;
#78415=EDGE_CURVE ( 'NONE', #14287, #169596, #42502, .T. ) ;
#78437=CARTESIAN_POINT ( 'NONE',  ( 8.779421058653776200, 13.51919467333984493, -7.714288002668382660 ) ) ;
#78440=CARTESIAN_POINT ( 'NONE',  ( 8.110954823418250470, 13.89836686726292037, 9.741300253657557917 ) ) ;
#78473=CARTESIAN_POINT ( 'NONE',  ( -12.76914910123260682, 7.416938840849524262, -2.145643146812736823 ) ) ;
#78479=AXIS2_PLACEMENT_3D ( 'NONE', #138108, #68798, #17914 ) ;
#78492=CARTESIAN_POINT ( 'NONE',  ( -9.608184375605320682, 15.11803084963731258, 7.189074558345553534 ) ) ;
#78499=CARTESIAN_POINT ( 'NONE',  ( 11.83030212645851620, 7.766851926455670352, -1.746998778190154589 ) ) ;
#78534=( GEOMETRIC_REPRESENTATION_CONTEXT ( 3 ) GLOBAL_UNCERTAINTY_ASSIGNED_CONTEXT ( ( #118229 ) ) GLOBAL_UNIT_ASSIGNED_CONTEXT ( ( #53637, #69855, #100254 ) ) REPRESENTATION_CONTEXT ( 'NONE', 'WORKASPACE' ) );
#78548=CARTESIAN_POINT ( 'NONE',  ( -11.88508768177337771, 7.945503028788528432, -1.311673572704820767 ) ) ;
#78549=ADVANCED_FACE ( 'NONE', ( #201283 ), #137396, .T. ) ;
#78556=CARTESIAN_POINT ( 'NONE',  ( -11.95485367524497811, 9.001114148948307303, 0.3044536461800395610 ) ) ;
#78559=FILL_AREA_STYLE ('',( #43954 ) ) ;
#78585=CARTESIAN_POINT ( 'NONE',  ( -11.77618483200234500, 4.711409542047888976, 4.977076041189349098 ) ) ;
#78589=CIRCLE ( 'NONE', #189306, 0.5000000000000008882 ) ;
#78594=ORIENTED_EDGE ( 'NONE', *, *, #24813, .T. ) ;
#78605=CARTESIAN_POINT ( 'NONE',  ( -11.78331023100045627, 12.22000000000000064, -1.800000000000001155 ) ) ;
#78625=CARTESIAN_POINT ( 'NONE',  ( 9.406792723036287995, 4.446947629225665111, 7.380298948578114526 ) ) ;
#78653=CARTESIAN_POINT ( 'NONE',  ( -10.80887392267048241, 4.296486016114100082, -4.677321330754881323 ) ) ;
#78662=CARTESIAN_POINT ( 'NONE',  ( -11.81905481421901705, 12.34264344382733469, -1.592167362352180593 ) ) ;
#78675=FACE_BOUND ( 'NONE', #118382, .T. ) ;
#78682=MECHANICAL_DESIGN_GEOMETRIC_PRESENTATION_REPRESENTATION('',(#106271),#40516);
#78683=EDGE_CURVE ( 'NONE', #84713, #149901, #47165, .T. ) ;
#78721=CYLINDRICAL_SURFACE ( 'NONE', #167099, 0.08000000000000020983 ) ;
#78727=EDGE_CURVE ( 'NONE', #29327, #101924, #85878, .T. ) ;
#78737=EDGE_LOOP ( 'NONE', ( #59741, #211394, #18489, #124124 ) ) ;
#78754=B_SPLINE_CURVE_WITH_KNOTS ( 'NONE', 3,
 ( #31449, #177701, #163584, #94336, #113831, #130088 ),
 .UNSPECIFIED., .F., .F.,
 ( 4, 2, 4 ),
 ( 0.001105973075985389100, 0.001142139074170185750, 0.001178305072354982400 ),
 .UNSPECIFIED. ) ;
#78756=SURFACE_SIDE_STYLE ('',( #12680 ) ) ;
#78760=FILL_AREA_STYLE ('',( #12684 ) ) ;
#78763=AXIS2_PLACEMENT_3D ( 'NONE', #138690, #76858, #191663 ) ;
#78781=CARTESIAN_POINT ( 'NONE',  ( -11.80247861663003484, 11.29999999999997939, 1.695431928471866190 ) ) ;
#78790=CARTESIAN_POINT ( 'NONE',  ( 9.278968692716386357, 13.84997945651597639, -7.537346677959899210 ) ) ;
#78809=EDGE_LOOP ( 'NONE', ( #96308, #119340, #4390, #170228 ) ) ;
#78825=CARTESIAN_POINT ( 'NONE',  ( -11.94105721237523099, 13.52740390989733221, -1.187919463087249827 ) ) ;
#78831=CARTESIAN_POINT ( 'NONE',  ( 7.873842894595653341, 14.32264345063075694, -9.058338245841589753 ) ) ;
#78841=CARTESIAN_POINT ( 'NONE',  ( 9.742269887272128059, 13.15996534559037912, -8.088430353861673083 ) ) ;
#78876=ORIENTED_EDGE ( 'NONE', *, *, #149964, .T. ) ;
#78883=DIRECTION ( 'NONE',  ( 1.000000000000000000, -0.000000000000000000, -0.000000000000000000 ) ) ;
#78896=FACE_OUTER_BOUND ( 'NONE', #162639, .T. ) ;
#78899=( NAMED_UNIT ( * ) PLANE_ANGLE_UNIT ( ) SI_UNIT ( $, .RADIAN. ) );
#78911=AXIS2_PLACEMENT_3D ( 'NONE', #88931, #7640, #126831 ) ;
#78916=ORIENTED_EDGE ( 'NONE', *, *, #27372, .F. ) ;
#78947=MECHANICAL_DESIGN_GEOMETRIC_PRESENTATION_REPRESENTATION('',(#61646),#9688);
#78948=( BOUNDED_SURFACE ( )  B_SPLINE_SURFACE ( 3, 2, ( 
 ( #195212, #164837, #147536 ),
 ( #46848, #213557, #112962 ),
 ( #178974, #65179, #96672 ),
 ( #48969, #131333, #144374 ),
 ( #60939, #162722, #176826 ),
 ( #14294, #197327, #193059 ) ),
 .UNSPECIFIED., .F., .F., .F. ) 
 B_SPLINE_SURFACE_WITH_KNOTS ( ( 4, 2, 4 ),
 ( 3, 3 ),
 ( 0.000000000000000000, 0.0003831416164015018179, 0.0007662832328030036357 ),
 ( 0.000000000000000000, 1.000000000000000000 ),
 .UNSPECIFIED. ) 
 GEOMETRIC_REPRESENTATION_ITEM ( )  RATIONAL_B_SPLINE_SURFACE ( (
 ( 1.000000000000000000, 0.7071067811865475727, 1.000000000000000000),
 ( 1.000000000000000000, 0.6829713513653348222, 1.000000000000000000),
 ( 1.000000000000000000, 0.6534833722372194176, 1.000000000000000000),
 ( 1.000000000000000000, 0.6054027484662655167, 1.000000000000000000),
 ( 1.000000000000000000, 0.5875453974414869274, 1.000000000000000000),
 ( 1.000000000000000000, 0.5879095031487528988, 1.000000000000000000) ) ) 
 REPRESENTATION_ITEM ( '' )  SURFACE ( )  );
#78987=SURFACE_STYLE_USAGE ( .BOTH. , #27030 ) ;
#78989=CYLINDRICAL_SURFACE ( 'NONE', #171146, 10.75000000000000000 ) ;
#78999=CARTESIAN_POINT ( 'NONE',  ( -10.83017591827266557, 4.360326817186668258, 4.636531744782178777 ) ) ;
#79007=AXIS2_PLACEMENT_3D ( 'NONE', #15898, #198907, #148070 ) ;
#79013=ORIENTED_EDGE ( 'NONE', *, *, #173301, .F. ) ;
#79034=B_SPLINE_CURVE_WITH_KNOTS ( 'NONE', 3,
 ( #46399, #15987, #196895, #97287, #34387, #31214, #179593 ),
 .UNSPECIFIED., .F., .F.,
 ( 4, 3, 4 ),
 ( 2.452946696045431814E-07, 0.0004046562657335614943, 0.0006364688305826464486 ),
 .UNSPECIFIED. ) ;
#79057=EDGE_LOOP ( 'NONE', ( #185327, #164167, #97790, #178788 ) ) ;
#79080=CARTESIAN_POINT ( 'NONE',  ( 11.92619526913700057, 10.89999999999998259, 1.328859060402682868 ) ) ;
#79081=DIRECTION ( 'NONE',  ( 0.000000000000000000, 0.000000000000000000, 1.000000000000000000 ) ) ;
#79100=CARTESIAN_POINT ( 'NONE',  ( -11.04536101718726293, 10.90000000000000036, -1.100000000000002087 ) ) ;
#79110=ORIENTED_EDGE ( 'NONE', *, *, #76805, .T. ) ;
#79116=CIRCLE ( 'NONE', #186408, 0.08000000000000015432 ) ;
#79124=VERTEX_POINT ( 'NONE', #208028 ) ;
#79134=EDGE_CURVE ( 'NONE', #48021, #23152, #69745, .T. ) ;
#79146=CARTESIAN_POINT ( 'NONE',  ( -15.75000000000000000, 10.89999999999998259, 3.599999999999999201 ) ) ;
#79163=FILL_AREA_STYLE ('',( #33608 ) ) ;
#79193=EDGE_LOOP ( 'NONE', ( #161979, #196088, #49373, #147330 ) ) ;
#79197=CARTESIAN_POINT ( 'NONE',  ( -9.801034077160730718, 4.485124939227990382, -6.925749731595153946 ) ) ;
#79201=EDGE_CURVE ( 'NONE', #58680, #28791, #28562, .T. ) ;
#79233=CARTESIAN_POINT ( 'NONE',  ( -10.62873463776380234, 9.799999999999982947, 3.199999999999997957 ) ) ;
#79256=EDGE_CURVE ( 'NONE', #72298, #200044, #59790, .T. ) ;
#79258=DIRECTION ( 'NONE',  ( 0.000000000000000000, 0.000000000000000000, 1.000000000000000000 ) ) ;
#79266=CARTESIAN_POINT ( 'NONE',  ( 11.92045683181315141, 9.947240721205149683, -1.382340670101858571 ) ) ;
#79267=EDGE_LOOP ( 'NONE', ( #53420, #131727, #188893, #36911 ) ) ;
#79300=VERTEX_POINT ( 'NONE', #75910 ) ;
#79325=EDGE_CURVE ( 'NONE', #122534, #101488, #170479, .T. ) ;
#79336=CIRCLE ( 'NONE', #189562, 11.67999999982603399 ) ;
#79379=DIRECTION ( 'NONE',  ( 0.000000000000000000, 0.000000000000000000, -1.000000000000000000 ) ) ;
#79400=VERTEX_POINT ( 'NONE', #61795 ) ;
#79409=CARTESIAN_POINT ( 'NONE',  ( 12.04878676029568751, 8.355254920624089365, 5.374760359037731305 ) ) ;
#79423=ORIENTED_EDGE ( 'NONE', *, *, #144259, .F. ) ;
#79431=CARTESIAN_POINT ( 'NONE',  ( 11.33772463945036790, 10.90000000000000036, -3.600000000000002309 ) ) ;
#79432=LINE ( 'NONE', #209404, #111593 ) ;
#79440=AXIS2_PLACEMENT_3D ( 'NONE', #93252, #146271, #159286 ) ;
#79457=EDGE_CURVE ( 'NONE', #164408, #91407, #199406, .T. ) ;
#79462=CARTESIAN_POINT ( 'NONE',  ( -11.77588451118714730, 7.698608310071745287, 2.073293985440898268 ) ) ;
#79465=CARTESIAN_POINT ( 'NONE',  ( 0.6674790882334122877, 15.00000000000000355, 11.66566053519463608 ) ) ;
#79505=CARTESIAN_POINT ( 'NONE',  ( 0.000000000000000000, 3.999999999999996447, 0.000000000000000000 ) ) ;
#79509=CARTESIAN_POINT ( 'NONE',  ( 7.209027064991026634, 14.97176420577651079, -9.190340992810662968 ) ) ;
#79512=CARTESIAN_POINT ( 'NONE',  ( 8.232418323234554691, 14.52480782996326880, 8.289887465044873949 ) ) ;
#79544=CARTESIAN_POINT ( 'NONE',  ( -11.76696981052429614, 4.673730779118272061, -4.995440715239800156 ) ) ;
#79562=ORIENTED_EDGE ( 'NONE', *, *, #9705, .F. ) ;
#79569=CARTESIAN_POINT ( 'NONE',  ( 11.95068985293163344, 7.567001936134044371, 0.4555898092883722827 ) ) ;
#79579=( BOUNDED_SURFACE ( )  B_SPLINE_SURFACE ( 3, 3, ( 
 ( #121030, #137210, #116723, #203232, #52731, #38628, #154515, #37552, #104704, #169684, #167554, #170754, #70020, #150253, #182723, #19155, #135077, #6096, #72164, #138273, #34342, #118865, #201090, #36479, #123181, #206447, #77522, #55944, #92736, #11447 ),
 ( #126363, #105801, #59138, #204287, #93805, #122097, #8249, #43980, #41855, #110099, #40779, #26634, #158781, #192322, #74333, #73237, #140435, #58075, #176110, #141511, #205374, #188061, #139344, #171825, #155582, #159845, #57009, #207519, #109030, #24485 ),
 ( #10378, #25565, #27710, #191255, #124237, #157729, #76454, #9324, #125297, #190197, #42920, #175049, #142562, #107965, #173993, #208568, #39690, #91676, #90597, #23419, #189141, #89530, #60202, #7167, #75398, #106885, #172911, #156656, #84725, #134584 ),
 ( #133518, #200584, #194474, #128506, #35970, #149736, #144707, #1315, #143643, #94866, #28783, #150814, #117291, #209637, #2377, #145775, #183288, #118360, #80734, #100965, #199524, #160920, #51168, #47190, #12514, #61277, #177166, #29858, #68455, #113303 ),
 ( #178243, #78585, #67376, #211776, #179310, #163060, #46117, #193409, #112234, #210718, #63414, #52232, #45053, #34892, #127439, #102048, #111165, #161995, #13585, #79658, #30931, #184347, #167054, #18647, #97007, #19717, #62346, #129566, #14640, #195552 ),
 ( #95939, #168117, #139904, #23978, #152928, #56500, #120510, #137764, #5571, #135626, #171306, #22899, #71650, #121581, #69518, #205934, #203784, #57567, #136694, #122661, #40255, #7726, #104189, #169175, #170238, #154003, #123724, #89014, #86863, #201647 ),
 ( #90080, #37032, #55429, #53295, #189687, #187552, #87930, #39182, #188623, #105268, #41338, #72733, #21822, #155068, #172390, #6656, #138829, #204847, #106366, #156143, #73809, #107447, #173472, #85796, #151876, #3450, #186486, #119427, #4506, #185414 ) ),
 .UNSPECIFIED., .T., .F., .F. ) 
 B_SPLINE_SURFACE_WITH_KNOTS ( ( 4, 3, 4 ),
 ( 4, 2, 2, 2, 2, 2, 2, 2, 2, 2, 2, 2, 2, 2, 4 ),
 ( 0.000000000000000000, 0.5000000000000000000, 1.000000000000000000 ),
 ( 0.3904182756812821231, 0.3921283039710705687, 0.3938383322608589587, 0.3972583888404358499, 0.4040985019995896321, 0.4177787283178971967, 0.4451391809545123257, 0.4999364453639513206, 0.5547656701200603946, 0.5821739285757332460, 0.5958780578035696163, 0.6027301224174878014, 0.6061561547244469494, 0.6078691708779264680, 0.6095821870314059865 ),
 .UNSPECIFIED. ) 
 GEOMETRIC_REPRESENTATION_ITEM ( )  RATIONAL_B_SPLINE_SURFACE ( (
 ( 1.000000000000000000, 1.000000000000000000, 1.000000000000000000, 1.000000000000000000, 1.000000000000000000, 1.000000000000000000, 1.000000000000000000, 1.000000000000000000, 1.000000000000000000, 1.000000000000000000, 1.000000000000000000, 1.000000000000000000, 1.000000000000000000, 1.000000000000000000, 1.000000000000000000, 1.000000000000000000, 1.000000000000000000, 1.000000000000000000, 1.000000000000000000, 1.000000000000000000, 1.000000000000000000, 1.000000000000000000, 1.000000000000000000, 1.000000000000000000, 1.000000000000000000, 1.000000000000000000, 1.000000000000000000, 1.000000000000000000, 1.000000000000000000, 1.000000000000000000),
 ( 0.3333333333333333703, 0.3333333333333333703, 0.3333333333333333703, 0.3333333333333333703, 0.3333333333333333703, 0.3333333333333333703, 0.3333333333333333703, 0.3333333333333333703, 0.3333333333333333703, 0.3333333333333333703, 0.3333333333333333703, 0.3333333333333333703, 0.3333333333333333703, 0.3333333333333333703, 0.3333333333333333703, 0.3333333333333333703, 0.3333333333333333703, 0.3333333333333333703, 0.3333333333333333703, 0.3333333333333333703, 0.3333333333333333703, 0.3333333333333333703, 0.3333333333333333703, 0.3333333333333333703, 0.3333333333333333703, 0.3333333333333333703, 0.3333333333333333703, 0.3333333333333333703, 0.3333333333333333703, 0.3333333333333333703),
 ( 0.3333333333333333703, 0.3333333333333333703, 0.3333333333333333703, 0.3333333333333333703, 0.3333333333333333703, 0.3333333333333333703, 0.3333333333333333703, 0.3333333333333333703, 0.3333333333333333703, 0.3333333333333333703, 0.3333333333333333703, 0.3333333333333333703, 0.3333333333333333703, 0.3333333333333333703, 0.3333333333333333703, 0.3333333333333333703, 0.3333333333333333703, 0.3333333333333333703, 0.3333333333333333703, 0.3333333333333333703, 0.3333333333333333703, 0.3333333333333333703, 0.3333333333333333703, 0.3333333333333333703, 0.3333333333333333703, 0.3333333333333333703, 0.3333333333333333703, 0.3333333333333333703, 0.3333333333333333703, 0.3333333333333333703),
 ( 1.000000000000000000, 1.000000000000000000, 1.000000000000000000, 1.000000000000000000, 1.000000000000000000, 1.000000000000000000, 1.000000000000000000, 1.000000000000000000, 1.000000000000000000, 1.000000000000000000, 1.000000000000000000, 1.000000000000000000, 1.000000000000000000, 1.000000000000000000, 1.000000000000000000, 1.000000000000000000, 1.000000000000000000, 1.000000000000000000, 1.000000000000000000, 1.000000000000000000, 1.000000000000000000, 1.000000000000000000, 1.000000000000000000, 1.000000000000000000, 1.000000000000000000, 1.000000000000000000, 1.000000000000000000, 1.000000000000000000, 1.000000000000000000, 1.000000000000000000),
 ( 0.3333333333333333703, 0.3333333333333333703, 0.3333333333333333703, 0.3333333333333333703, 0.3333333333333333703, 0.3333333333333333703, 0.3333333333333333703, 0.3333333333333333703, 0.3333333333333333703, 0.3333333333333333703, 0.3333333333333333703, 0.3333333333333333703, 0.3333333333333333703, 0.3333333333333333703, 0.3333333333333333703, 0.3333333333333333703, 0.3333333333333333703, 0.3333333333333333703, 0.3333333333333333703, 0.3333333333333333703, 0.3333333333333333703, 0.3333333333333333703, 0.3333333333333333703, 0.3333333333333333703, 0.3333333333333333703, 0.3333333333333333703, 0.3333333333333333703, 0.3333333333333333703, 0.3333333333333333703, 0.3333333333333333703),
 ( 0.3333333333333333703, 0.3333333333333333703, 0.3333333333333333703, 0.3333333333333333703, 0.3333333333333333703, 0.3333333333333333703, 0.3333333333333333703, 0.3333333333333333703, 0.3333333333333333703, 0.3333333333333333703, 0.3333333333333333703, 0.3333333333333333703, 0.3333333333333333703, 0.3333333333333333703, 0.3333333333333333703, 0.3333333333333333703, 0.3333333333333333703, 0.3333333333333333703, 0.3333333333333333703, 0.3333333333333333703, 0.3333333333333333703, 0.3333333333333333703, 0.3333333333333333703, 0.3333333333333333703, 0.3333333333333333703, 0.3333333333333333703, 0.3333333333333333703, 0.3333333333333333703, 0.3333333333333333703, 0.3333333333333333703),
 ( 1.000000000000000000, 1.000000000000000000, 1.000000000000000000, 1.000000000000000000, 1.000000000000000000, 1.000000000000000000, 1.000000000000000000, 1.000000000000000000, 1.000000000000000000, 1.000000000000000000, 1.000000000000000000, 1.000000000000000000, 1.000000000000000000, 1.000000000000000000, 1.000000000000000000, 1.000000000000000000, 1.000000000000000000, 1.000000000000000000, 1.000000000000000000, 1.000000000000000000, 1.000000000000000000, 1.000000000000000000, 1.000000000000000000, 1.000000000000000000, 1.000000000000000000, 1.000000000000000000, 1.000000000000000000, 1.000000000000000000, 1.000000000000000000, 1.000000000000000000) ) ) 
 REPRESENTATION_ITEM ( '' )  SURFACE ( )  );
#79618=CARTESIAN_POINT ( 'NONE',  ( -11.73318219666202999, 7.416709190724854572, 2.527811172656401428 ) ) ;
#79626=CARTESIAN_POINT ( 'NONE',  ( -11.71717583921413208, 8.541564709976100289, -2.387000931153457461 ) ) ;
#79639=ORIENTED_EDGE ( 'NONE', *, *, #33991, .F. ) ;
#79642=CIRCLE ( 'NONE', #159264, 0.07999999999999946043 ) ;
#79658=CARTESIAN_POINT ( 'NONE',  ( -12.06809232949933275, 5.701620653239091396, -4.345812045493805620 ) ) ;
#79661=ORIENTED_EDGE ( 'NONE', *, *, #192419, .T. ) ;
#79662=DIRECTION ( 'NONE',  ( 0.000000000000000000, 1.000000000000000000, 0.000000000000000000 ) ) ;
#79668=CARTESIAN_POINT ( 'NONE',  ( -10.62873463776380056, 9.799999999999998934, -3.200000000000001510 ) ) ;
#79673=ORIENTED_EDGE ( 'NONE', *, *, #90947, .F. ) ;
#79685=DIRECTION ( 'NONE',  ( -0.2684563758389304500, -5.222015543130708508E-15, 0.9632918427306581544 ) ) ;
#79686=( LENGTH_UNIT ( ) NAMED_UNIT ( * ) SI_UNIT ( .MILLI., .METRE. ) );
#79725=CARTESIAN_POINT ( 'NONE',  ( -10.90756946389101323, 4.636105284860334130, -4.485523696119589232 ) ) ;
#79733=( NAMED_UNIT ( * ) PLANE_ANGLE_UNIT ( ) SI_UNIT ( $, .RADIAN. ) );
#79744=CARTESIAN_POINT ( 'NONE',  ( -11.84668730067608422, 13.39999999999998259, 1.399999999999998357 ) ) ;
#79761=DIRECTION ( 'NONE',  ( 0.000000000000000000, -0.000000000000000000, 1.000000000000000000 ) ) ;
#79773=AXIS2_PLACEMENT_3D ( 'NONE', #92236, #191814, #77005 ) ;
#79789=CARTESIAN_POINT ( 'NONE',  ( 11.55950211276791251, 9.719999999999998863, -3.221476510067114329 ) ) ;
#79791=CARTESIAN_POINT ( 'NONE',  ( -11.33772463945036968, 19.00000000000000000, -3.680000000000002824 ) ) ;
#79792=MECHANICAL_DESIGN_GEOMETRIC_PRESENTATION_REPRESENTATION('',(#180141),#200820);
#79823=SURFACE_SIDE_STYLE ('',( #194640 ) ) ;
#79844=CARTESIAN_POINT ( 'NONE',  ( -0.001355188237250771121, 15.43765366524399596, 11.93721149935645265 ) ) ;
#79861=CARTESIAN_POINT ( 'NONE',  ( 9.245229451055090308, 14.18885291725855424, -7.650713753047223342 ) ) ;
#79879=ORIENTED_EDGE ( 'NONE', *, *, #98822, .T. ) ;
#79880=ADVANCED_FACE ( 'NONE', ( #189393 ), #156916, .T. ) ;
#79885=CARTESIAN_POINT ( 'NONE',  ( -11.01135777277261951, 11.00625186781170939, 1.399999999999998579 ) ) ;
#79886=CARTESIAN_POINT ( 'NONE',  ( -10.30104275384242740, 4.689840931292195592, -5.506867539468097483 ) ) ;
#79900=CARTESIAN_POINT ( 'NONE',  ( 7.695629581373169437, 14.38868833749761400, -9.210593468082514335 ) ) ;
#79907=ORIENTED_EDGE ( 'NONE', *, *, #184582, .F. ) ;
#79910=CARTESIAN_POINT ( 'NONE',  ( 9.691970092379245116, 13.38142374607198803, 8.152522038325429321 ) ) ;
#79911=CIRCLE ( 'NONE', #65973, 0.08000000000000020983 ) ;
#79912=CARTESIAN_POINT ( 'NONE',  ( -10.41980074470002648, 5.020554563858687480, 5.279403930596816785 ) ) ;
#79919=ADVANCED_FACE ( 'NONE', ( #6358 ), #34021, .T. ) ;
#79922=ORIENTED_EDGE ( 'NONE', *, *, #61688, .F. ) ;
#79933=EDGE_CURVE ( 'NONE', #53115, #171829, #4403, .T. ) ;
#79939=FACE_OUTER_BOUND ( 'NONE', #153731, .T. ) ;
#79949=ORIENTED_EDGE ( 'NONE', *, *, #153604, .T. ) ;
#79971=( GEOMETRIC_REPRESENTATION_CONTEXT ( 3 ) GLOBAL_UNCERTAINTY_ASSIGNED_CONTEXT ( ( #13177 ) ) GLOBAL_UNIT_ASSIGNED_CONTEXT ( ( #106243, #158156, #24926 ) ) REPRESENTATION_CONTEXT ( 'NONE', 'WORKASPACE' ) );
#79990=VERTEX_POINT ( 'NONE', #112613 ) ;
#80063=CARTESIAN_POINT ( 'NONE',  ( -11.84668730067608422, 10.19999999999999929, -1.320000000000001616 ) ) ;
#80113=CARTESIAN_POINT ( 'NONE',  ( -2.996596126518174419, 14.55175791338114699, 11.58266829935393005 ) ) ;
#80122=CARTESIAN_POINT ( 'NONE',  ( 7.104593929172385636, 14.55347104122142810, 9.619174111504673164 ) ) ;
#80159=VERTEX_POINT ( 'NONE', #212154 ) ;
#80161=EDGE_CURVE ( 'NONE', #118044, #77503, #30236, .T. ) ;
#80166=DIRECTION ( 'NONE',  ( 0.000000000000000000, -0.000000000000000000, 1.000000000000000000 ) ) ;
#80175=B_SPLINE_CURVE_WITH_KNOTS ( 'NONE', 3,
 ( #34761, #118225, #2241, #33704, #181025, #100835 ),
 .UNSPECIFIED., .F., .F.,
 ( 4, 2, 4 ),
 ( 0.000000000000000000, 0.0003205138222656014457, 0.0006410276445312028913 ),
 .UNSPECIFIED. ) ;
#80186=ORIENTED_EDGE ( 'NONE', *, *, #211770, .T. ) ;
#80201=CARTESIAN_POINT ( 'NONE',  ( -11.97181042169641074, 13.88000000000000078, 0.8318531151397159373 ) ) ;
#80214=SURFACE_SIDE_STYLE ('',( #99663 ) ) ;
#80222=ORIENTED_EDGE ( 'NONE', *, *, #149964, .F. ) ;
#80226=EDGE_LOOP ( 'NONE', ( #82825, #46886, #76841, #83326, #27713 ) ) ;
#80281=CARTESIAN_POINT ( 'NONE',  ( 11.91294103507058288, 11.11460089956400843, -1.446263142085487674 ) ) ;
#80294=STYLED_ITEM ( 'NONE', ( #60244 ), #50933 ) ;
#80298=( NAMED_UNIT ( * ) PLANE_ANGLE_UNIT ( ) SI_UNIT ( $, .RADIAN. ) );
#80365=CIRCLE ( 'NONE', #121870, 11.18000000000000149 ) ;
#80382=ORIENTED_EDGE ( 'NONE', *, *, #183135, .F. ) ;
#80409=VERTEX_POINT ( 'NONE', #134164 ) ;
#80411=CARTESIAN_POINT ( 'NONE',  ( 0.000000000000000000, 12.22000000000000064, 0.000000000000000000 ) ) ;
#80417=CARTESIAN_POINT ( 'NONE',  ( 11.97929049433705551, 11.30000000000000249, -0.7046979865771820783 ) ) ;
#80428=EDGE_CURVE ( 'NONE', #91093, #173456, #120090, .T. ) ;
#80459=CARTESIAN_POINT ( 'NONE',  ( -11.89844258446856529, 9.771473106700385713, -1.560502987793169094 ) ) ;
#80465=DIRECTION ( 'NONE',  ( 1.000000000000000000, -0.000000000000000000, -0.000000000000000000 ) ) ;
#80478=CARTESIAN_POINT ( 'NONE',  ( 12.51085889473690749, 7.557192264108227420, 4.121037430627751519 ) ) ;
#80479=ORIENTED_EDGE ( 'NONE', *, *, #12043, .F. ) ;
#80506=CARTESIAN_POINT ( 'NONE',  ( -11.97178994924802353, 11.37999993797205178, -0.8322011300497250685 ) ) ;
#80533=CARTESIAN_POINT ( 'NONE',  ( -3.501245407925418274, 15.99999999999932321, 11.28115623562629466 ) ) ;
#80573=CARTESIAN_POINT ( 'NONE',  ( -11.82065545612590363, 8.157852845329689018, 2.282521414035399321 ) ) ;
#80578=CARTESIAN_POINT ( 'NONE',  ( 10.08935753863141471, 13.93683245669168969, -7.381900748183195304 ) ) ;
#80581=CARTESIAN_POINT ( 'NONE',  ( 7.122954113691880806, 13.97688634340336833, 9.257467215448135889 ) ) ;
#80589=ORIENTED_EDGE ( 'NONE', *, *, #57473, .F. ) ;
#80605=( GEOMETRIC_REPRESENTATION_CONTEXT ( 3 ) GLOBAL_UNCERTAINTY_ASSIGNED_CONTEXT ( ( #28371 ) ) GLOBAL_UNIT_ASSIGNED_CONTEXT ( ( #141855, #191605, #116556 ) ) REPRESENTATION_CONTEXT ( 'NONE', 'WORKASPACE' ) );
#80617=CARTESIAN_POINT ( 'NONE',  ( -11.80100919632472589, 4.809168931535662495, -4.927235675632552159 ) ) ;
#80632=CARTESIAN_POINT ( 'NONE',  ( 0.000000000000000000, 14.48195938056239385, 0.000000000000000000 ) ) ;
#80646=CARTESIAN_POINT ( 'NONE',  ( 11.46937510643195779, 8.378953184613939342, -3.376433863712082761 ) ) ;
#80650=CARTESIAN_POINT ( 'NONE',  ( 11.84668730067608244, 13.40000000000000036, -1.320000000000001616 ) ) ;
#80675=CARTESIAN_POINT ( 'NONE',  ( 11.00592705432737972, 13.61019307346892759, 1.444010445236424856 ) ) ;
#80683=EDGE_CURVE ( 'NONE', #211122, #27064, #93171, .T. ) ;
#80684=CIRCLE ( 'NONE', #7987, 0.08000000000000020983 ) ;
#80693=DIRECTION ( 'NONE',  ( 0.000000000000000000, 0.000000000000000000, -1.000000000000000000 ) ) ;
#80697=CARTESIAN_POINT ( 'NONE',  ( -11.81798298708319273, 7.794783740815080186, -1.819802677367790444 ) ) ;
#80706=CARTESIAN_POINT ( 'NONE',  ( -10.52211599421016786, 5.354012650763439574, -5.769493145238611120 ) ) ;
#80722=CARTESIAN_POINT ( 'NONE',  ( -10.95308175811721085, 9.799999999999998934, -1.800000000000001155 ) ) ;
#80726=CARTESIAN_POINT ( 'NONE',  ( 11.84668730067608600, 10.89999999999998259, 1.319999999999998286 ) ) ;
#80728=EDGE_CURVE ( 'NONE', #127020, #24518, #209355, .T. ) ;
#80734=CARTESIAN_POINT ( 'NONE',  ( -11.88731729969462059, 7.000411858491159656, -4.404230128874679906 ) ) ;
#80742=ORIENTED_EDGE ( 'NONE', *, *, #107910, .T. ) ;
#80753=CARTESIAN_POINT ( 'NONE',  ( -11.92619526913700057, 12.69999999999998153, 1.328859060402682868 ) ) ;
#80755=CARTESIAN_POINT ( 'NONE',  ( 11.04536101718726293, 0.000000000000000000, -1.100000000000002087 ) ) ;
#80764=CARTESIAN_POINT ( 'NONE',  ( -5.975952631313489860, 15.44727933881517323, 10.36472687262296510 ) ) ;
#80777=CARTESIAN_POINT ( 'NONE',  ( 9.405838923370410498, 3.553052382342013704, 7.381490207074219434 ) ) ;
#80808=EDGE_LOOP ( 'NONE', ( #93266, #183080, #194085, #71174 ) ) ;
#80818=STYLED_ITEM ( 'NONE', ( #159412 ), #115007 ) ;
#80824=CARTESIAN_POINT ( 'NONE',  ( -11.92619525870747665, 13.52622296793678380, 1.328859154005173959 ) ) ;
#80881=ORIENTED_EDGE ( 'NONE', *, *, #211067, .T. ) ;
#80885=VERTEX_POINT ( 'NONE', #108102 ) ;
#80898=CARTESIAN_POINT ( 'NONE',  ( -15.75000000000000000, 13.40000000000000036, -1.400000000000001910 ) ) ;
#80900=( LENGTH_UNIT ( ) NAMED_UNIT ( * ) SI_UNIT ( .MILLI., .METRE. ) );
#80903=CARTESIAN_POINT ( 'NONE',  ( 10.62873463776380056, 12.29999999999998295, 3.199999999999997957 ) ) ;
#80908=AXIS2_PLACEMENT_3D ( 'NONE', #48786, #131158, #197149 ) ;
#80926=PRESENTATION_STYLE_ASSIGNMENT (( #165367 ) ) ;
#80935=CARTESIAN_POINT ( 'NONE',  ( 7.506010991098318819, 15.48982135686440031, -9.369134107302478753 ) ) ;
#80959=CARTESIAN_POINT ( 'NONE',  ( -9.970593631352514308, 5.552127128363319564, -5.997086463700067149 ) ) ;
#80961=EDGE_CURVE ( 'NONE', #19959, #101924, #110239, .T. ) ;
#80962=MECHANICAL_DESIGN_GEOMETRIC_PRESENTATION_REPRESENTATION('',(#150089),#112128);
#80969=CARTESIAN_POINT ( 'NONE',  ( -11.35610322553117513, 12.48578371070822790, 3.553412924323499755 ) ) ;
#80986=SURFACE_SIDE_STYLE ('',( #163310 ) ) ;
#80987=CARTESIAN_POINT ( 'NONE',  ( 10.13949827731025088, 13.65534166205038424, -7.300436427310208032 ) ) ;
#80997=CARTESIAN_POINT ( 'NONE',  ( 8.358554193140776079, 14.08791053918336367, -8.548382748741554238 ) ) ;
#80999=EDGE_LOOP ( 'NONE', ( #119413, #28347, #178406, #105509 ) ) ;
#81004=CARTESIAN_POINT ( 'NONE',  ( 0.07968937610752521716, 14.48238360795788893, 11.99973206003776660 ) ) ;
#81005=EDGE_CURVE ( 'NONE', #173182, #99531, #88169, .T. ) ;
#81030=FILL_AREA_STYLE ('',( #194775 ) ) ;
#81044=FACE_OUTER_BOUND ( 'NONE', #64724, .T. ) ;
#81058=DIRECTION ( 'NONE',  ( 0.000000000000000000, 1.000000000000000000, 0.000000000000000000 ) ) ;
#81091=DIRECTION ( 'NONE',  ( 0.000000000000000000, 0.000000000000000000, -1.000000000000000000 ) ) ;
#81107=CARTESIAN_POINT ( 'NONE',  ( 11.78331023100045627, 12.29999999999998295, 1.799999999999999600 ) ) ;
#81120=ADVANCED_FACE ( 'NONE', ( #82982 ), #78721, .T. ) ;
#81137=COLOUR_RGB ( '', 0.40784314, 0.44705882, 0.49803922) ;
#81158=ADVANCED_FACE ( 'NONE', ( #148011 ), #85249, .T. ) ;
#81168=( GEOMETRIC_REPRESENTATION_CONTEXT ( 3 ) GLOBAL_UNCERTAINTY_ASSIGNED_CONTEXT ( ( #145064 ) ) GLOBAL_UNIT_ASSIGNED_CONTEXT ( ( #120361, #87786, #141907 ) ) REPRESENTATION_CONTEXT ( 'NONE', 'WORKASPACE' ) );
#81197=CARTESIAN_POINT ( 'NONE',  ( 8.648791051114949724, 13.73763115593600048, 8.318960809290519620 ) ) ;
#81218=CARTESIAN_POINT ( 'NONE',  ( 11.81907076198591966, 11.25731224596471769, 1.592066415281218505 ) ) ;
#81220=AXIS2_PLACEMENT_3D ( 'NONE', #29081, #32275, #65796 ) ;
#81230=ORIENTED_EDGE ( 'NONE', *, *, #183845, .T. ) ;
#81250=ORIENTED_EDGE ( 'NONE', *, *, #154830, .T. ) ;
#81254=CARTESIAN_POINT ( 'NONE',  ( 9.508009452561562824, 4.000000000000000888, 7.612500000000001599 ) ) ;
#81258=CARTESIAN_POINT ( 'NONE',  ( -15.75000000000000000, 10.90000000000000036, -1.100000000000002087 ) ) ;
#81268=ORIENTED_EDGE ( 'NONE', *, *, #55036, .F. ) ;
#81279=STYLED_ITEM ( 'NONE', ( #98607 ), #189006 ) ;
#81284=CARTESIAN_POINT ( 'NONE',  ( -10.63776469506859534, 5.877592587992107376, 5.457754955663538965 ) ) ;
#81296=ORIENTED_EDGE ( 'NONE', *, *, #11376, .T. ) ;
#81303=CARTESIAN_POINT ( 'NONE',  ( -15.75000000000000000, 10.89999999999998259, 3.199999999999997957 ) ) ;
#81309=ORIENTED_EDGE ( 'NONE', *, *, #195648, .F. ) ;
#81333=MECHANICAL_DESIGN_GEOMETRIC_PRESENTATION_REPRESENTATION('',(#126407),#36316);
#81342=DIRECTION ( 'NONE',  ( 0.000000000000000000, 1.000000000000000000, 0.000000000000000000 ) ) ;
#81351=CARTESIAN_POINT ( 'NONE',  ( -11.97929049433705551, 13.80000000000000071, -0.7046979865771821894 ) ) ;
#81358=ORIENTED_EDGE ( 'NONE', *, *, #206408, .F. ) ;
#81362=DIRECTION ( 'NONE',  ( -0.000000000000000000, -1.000000000000000000, -0.000000000000000000 ) ) ;
#81363=EDGE_CURVE ( 'NONE', #115330, #24518, #63350, .T. ) ;
#81395=CARTESIAN_POINT ( 'NONE',  ( 11.01135777277262306, 11.00624935217894418, -1.400000000000002132 ) ) ;
#81396=ORIENTED_EDGE ( 'NONE', *, *, #11376, .F. ) ;
#81398=UNCERTAINTY_MEASURE_WITH_UNIT (LENGTH_MEASURE( 1.000000000000000082E-05 ), #207681, 'distance_accuracy_value', 'NONE');
#81403=ORIENTED_EDGE ( 'NONE', *, *, #121519, .T. ) ;
#81408=ORIENTED_EDGE ( 'NONE', *, *, #648, .T. ) ;
#81409=VERTEX_POINT ( 'NONE', #28697 ) ;
#81414=CARTESIAN_POINT ( 'NONE',  ( 10.95308175811721085, 12.29999999999998295, 1.799999999999999600 ) ) ;
#81426=ORIENTED_EDGE ( 'NONE', *, *, #47233, .T. ) ;
#81430=( GEOMETRIC_REPRESENTATION_CONTEXT ( 3 ) GLOBAL_UNCERTAINTY_ASSIGNED_CONTEXT ( ( #59816 ) ) GLOBAL_UNIT_ASSIGNED_CONTEXT ( ( #155137, #138897, #122728 ) ) REPRESENTATION_CONTEXT ( 'NONE', 'WORKASPACE' ) );
#81451=ORIENTED_EDGE ( 'NONE', *, *, #110186, .T. ) ;
#81456=CARTESIAN_POINT ( 'NONE',  ( -11.86687934130374522, 13.60951949616558565, 1.056332641424306606 ) ) ;
#81459=LINE ( 'NONE', #95608, #25450 ) ;
#81484=SURFACE_STYLE_FILL_AREA ( #212532 ) ;
#81485=CARTESIAN_POINT ( 'NONE',  ( 11.96535697748089078, 11.25262667064446198, -0.9148528286454237213 ) ) ;
#81513=DIRECTION ( 'NONE',  ( 0.000000000000000000, 0.000000000000000000, 1.000000000000000000 ) ) ;
#81522=DIRECTION ( 'NONE',  ( 0.000000000000000000, 0.000000000000000000, -1.000000000000000000 ) ) ;
#81541=CARTESIAN_POINT ( 'NONE',  ( 9.010018398950542462, 11.11739593148128158, 8.024259704181407216 ) ) ;
#81544=ORIENTED_EDGE ( 'NONE', *, *, #143656, .F. ) ;
#81575=VECTOR ( 'NONE', #109488, 1000.000000000000000 ) ;
#81595=CARTESIAN_POINT ( 'NONE',  ( -11.51301453142883346, 6.867562542198304421, 3.390093443801430073 ) ) ;
#81605=TOROIDAL_SURFACE ( 'NONE', #140407, 11.92000000000000348, 0.08000000000000000167 ) ;
#81633=EDGE_CURVE ( 'NONE', #121309, #23505, #113936, .T. ) ;
#81638=CARTESIAN_POINT ( 'NONE',  ( 9.634427881463707877, 13.63015724552533037, -8.222364378050974310 ) ) ;
#81658=EDGE_CURVE ( 'NONE', #115330, #70402, #77792, .T. ) ;
#81670=CARTESIAN_POINT ( 'NONE',  ( -10.94029418865078362, 4.766281873824294024, -4.419956640179717233 ) ) ;
#81679=ADVANCED_FACE ( 'NONE', ( #21998 ), #175119, .T. ) ;
#81701=COLOUR_RGB ( '', 0.08235294, 0.09019608, 0.10196078) ;
#81716=CARTESIAN_POINT ( 'NONE',  ( 11.81900460097218186, 9.842428651258618544, -1.592493057836596337 ) ) ;
#81739=DIRECTION ( 'NONE',  ( 1.000000000000000000, -0.000000000000000000, -0.000000000000000000 ) ) ;
#81753=CARTESIAN_POINT ( 'NONE',  ( -11.73415479055029209, 7.419463409362142770, -2.523393346103949053 ) ) ;
#81761=CARTESIAN_POINT ( 'NONE',  ( -11.37622529897019952, 7.826419360496526423, -3.683600133736221416 ) ) ;
#81764=FACE_OUTER_BOUND ( 'NONE', #35165, .T. ) ;
#81766=( GEOMETRIC_REPRESENTATION_CONTEXT ( 3 ) GLOBAL_UNCERTAINTY_ASSIGNED_CONTEXT ( ( #181028 ) ) GLOBAL_UNIT_ASSIGNED_CONTEXT ( ( #179827, #112759, #195002 ) ) REPRESENTATION_CONTEXT ( 'NONE', 'WORKASPACE' ) );
#81773=EDGE_LOOP ( 'NONE', ( #157483, #154545, #29394, #157806 ) ) ;
#81775=( GEOMETRIC_REPRESENTATION_CONTEXT ( 3 ) GLOBAL_UNCERTAINTY_ASSIGNED_CONTEXT ( ( #53163 ) ) GLOBAL_UNIT_ASSIGNED_CONTEXT ( ( #207917, #194875, #162395 ) ) REPRESENTATION_CONTEXT ( 'NONE', 'WORKASPACE' ) );
#81862=ORIENTED_EDGE ( 'NONE', *, *, #69515, .T. ) ;
#81869=VECTOR ( 'NONE', #109423, 1000.000000000000000 ) ;
#81896=( LENGTH_UNIT ( ) NAMED_UNIT ( * ) SI_UNIT ( .MILLI., .METRE. ) );
#81922=CARTESIAN_POINT ( 'NONE',  ( 11.41381675112453387, 10.19999999999999929, -3.704697986577184299 ) ) ;
#81935=EDGE_CURVE ( 'NONE', #132208, #142386, #115363, .T. ) ;
#81937=CIRCLE ( 'NONE', #192614, 0.07999999999999946043 ) ;
#81989=CARTESIAN_POINT ( 'NONE',  ( 11.96533679318060095, 9.847539888129947627, -0.9151144679398871551 ) ) ;
#81990=( LENGTH_UNIT ( ) NAMED_UNIT ( * ) SI_UNIT ( .MILLI., .METRE. ) );
#81992=CARTESIAN_POINT ( 'NONE',  ( 11.86145016429273369, 10.09412591486744226, -1.100000000000002087 ) ) ;
#82019=CARTESIAN_POINT ( 'NONE',  ( -10.33433454857960321, 4.766519530047388820, -5.444264161973041638 ) ) ;
#82032=CARTESIAN_POINT ( 'NONE',  ( 8.776573235218648961, 13.27486625357122563, -8.183627694784485485 ) ) ;
#82041=CARTESIAN_POINT ( 'NONE',  ( 9.312415520145556513, 13.13417835526394306, 6.702754826033684665 ) ) ;
#82052=CARTESIAN_POINT ( 'NONE',  ( 6.928203230275523872, 14.53091781611523814, -9.797958971132697314 ) ) ;
#82054=ORIENTED_EDGE ( 'NONE', *, *, #110293, .T. ) ;
#82055=MECHANICAL_DESIGN_GEOMETRIC_PRESENTATION_REPRESENTATION('',(#120187),#137447);
#82060=CARTESIAN_POINT ( 'NONE',  ( 0.03257971700928394970, 14.52926532189213127, 11.98509109043141940 ) ) ;
#82067=PLANE ( 'NONE',  #59764 ) ;
#82068=AXIS2_PLACEMENT_3D ( 'NONE', #121376, #187350, #203578 ) ;
#82099=PLANE ( 'NONE',  #123725 ) ;
#82169=AXIS2_PLACEMENT_3D ( 'NONE', #136132, #167550, #19151 ) ;
#82182=EDGE_CURVE ( 'NONE', #29604, #144257, #131917, .T. ) ;
#82184=CARTESIAN_POINT ( 'NONE',  ( -9.523271316415712562, 15.37774589682084247, 7.301265812912605568 ) ) ;
#82206=CARTESIAN_POINT ( 'NONE',  ( -9.495238110454899072, 14.82843120887656951, -7.231499654889533169 ) ) ;
#82220=EDGE_CURVE ( 'NONE', #73245, #195702, #160571, .T. ) ;
#82242=CARTESIAN_POINT ( 'NONE',  ( 11.33772463945037146, 12.59088423488572062, 3.599999999999998757 ) ) ;
#82248=CARTESIAN_POINT ( 'NONE',  ( 8.435195442881084915, 13.95515841652898281, 8.535564829755013960 ) ) ;
#82270=EDGE_LOOP ( 'NONE', ( #135087, #206688, #93389, #43519 ) ) ;
#82286=CARTESIAN_POINT ( 'NONE',  ( 11.89317557362582711, 9.837241561624077590, -1.599935658896034729 ) ) ;
#82297=CARTESIAN_POINT ( 'NONE',  ( -11.41381675112453387, 12.69999999999998153, 3.704697986577180746 ) ) ;
#82301=ORIENTED_EDGE ( 'NONE', *, *, #83013, .T. ) ;
#82316=SURFACE_STYLE_USAGE ( .BOTH. , #162533 ) ;
#82325=AXIS2_PLACEMENT_3D ( 'NONE', #108560, #173523, #141040 ) ;
#82333=CARTESIAN_POINT ( 'NONE',  ( -11.89630347798379972, 8.889736554344878527, 1.217639561629326517 ) ) ;
#82336=( NAMED_UNIT ( * ) SI_UNIT ( $, .STERADIAN. ) SOLID_ANGLE_UNIT ( ) );
#82393=CARTESIAN_POINT ( 'NONE',  ( 11.41381675112453564, 11.03005666089991799, 3.704697986577179858 ) ) ;
#82401=CIRCLE ( 'NONE', #213806, 11.95586206894151005 ) ;
#82427=ORIENTED_EDGE ( 'NONE', *, *, #108367, .T. ) ;
#82446=CARTESIAN_POINT ( 'NONE',  ( 11.33772463945037146, 10.19999999999998153, 3.599999999999999201 ) ) ;
#82448=CARTESIAN_POINT ( 'NONE',  ( -10.41980074470002648, 5.020554563858687480, 5.279403930596816785 ) ) ;
#82464=CARTESIAN_POINT ( 'NONE',  ( 10.50000000000000178, 10.90000000000000036, -3.600000000000002309 ) ) ;
#82480=CARTESIAN_POINT ( 'NONE',  ( -9.494322902919321905, 15.33478604102567999, -7.339005329679038070 ) ) ;
#82505=CARTESIAN_POINT ( 'NONE',  ( 1.369155121446740960E-15, 18.91999999999999815, -11.18000000000000149 ) ) ;
#82508=CARTESIAN_POINT ( 'NONE',  ( -11.84668729035104384, 12.59481419982588690, -1.400000000000001688 ) ) ;
#82535=SURFACE_STYLE_USAGE ( .BOTH. , #193089 ) ;
#82557=DIRECTION ( 'NONE',  ( -0.9982742078614211811, 0.000000000000000000, -0.05872483221476467591 ) ) ;
#82585=DIRECTION ( 'NONE',  ( 0.000000000000000000, 0.000000000000000000, -1.000000000000000000 ) ) ;
#82587=( LENGTH_UNIT ( ) NAMED_UNIT ( * ) SI_UNIT ( .MILLI., .METRE. ) );
#82598=CARTESIAN_POINT ( 'NONE',  ( 9.224544533040768712, 13.18315223404452574, 9.019998505197962757 ) ) ;
#82618=CARTESIAN_POINT ( 'NONE',  ( 0.000000000000000000, 11.29999999999998117, 0.000000000000000000 ) ) ;
#82633=EDGE_CURVE ( 'NONE', #7968, #45206, #81459, .T. ) ;
#82677=( NAMED_UNIT ( * ) SI_UNIT ( $, .STERADIAN. ) SOLID_ANGLE_UNIT ( ) );
#82697=CARTESIAN_POINT ( 'NONE',  ( 7.019708803244085082, 15.99401525430995186, -9.337312011067078643 ) ) ;
#82708=EDGE_CURVE ( 'NONE', #92493, #96092, #98524, .T. ) ;
#82721=CARTESIAN_POINT ( 'NONE',  ( -10.95308175811721085, 13.79999999999998295, 1.799999999999999600 ) ) ;
#82730=MECHANICAL_DESIGN_GEOMETRIC_PRESENTATION_REPRESENTATION('',(#30811),#138089);
#82737=EDGE_CURVE ( 'NONE', #90728, #175932, #84199, .T. ) ;
#82760=EDGE_LOOP ( 'NONE', ( #107712, #20127, #47101, #41425 ) ) ;
#82762=CARTESIAN_POINT ( 'NONE',  ( 11.33772463945036790, 10.19999999999999929, -3.600000000000000977 ) ) ;
#82769=CARTESIAN_POINT ( 'NONE',  ( 7.874165004059028306, 14.38583653512666416, -8.999470220878452054 ) ) ;
#82774=B_SPLINE_CURVE_WITH_KNOTS ( 'NONE', 3,
 ( #155756, #43095, #76622, #104881, #156832, #7341 ),
 .UNSPECIFIED., .F., .F.,
 ( 4, 2, 4 ),
 ( 0.000000000000000000, 0.0003132070624402877746, 0.0006264141248805755492 ),
 .UNSPECIFIED. ) ;
#82806=( NAMED_UNIT ( * ) SI_UNIT ( $, .STERADIAN. ) SOLID_ANGLE_UNIT ( ) );
#82809=CARTESIAN_POINT ( 'NONE',  ( -11.86145016429273014, 12.69999999999999929, -1.100000000000000533 ) ) ;
#82810=CARTESIAN_POINT ( 'NONE',  ( -11.51166771951771217, 6.864275254849497188, -3.394607536566083272 ) ) ;
#82825=ORIENTED_EDGE ( 'NONE', *, *, #79256, .F. ) ;
#82833=AXIS2_PLACEMENT_3D ( 'NONE', #159438, #60872, #28373 ) ;
#82854=ORIENTED_EDGE ( 'NONE', *, *, #60154, .F. ) ;
#82866=( NAMED_UNIT ( * ) PLANE_ANGLE_UNIT ( ) SI_UNIT ( $, .RADIAN. ) );
#82868=CARTESIAN_POINT ( 'NONE',  ( 11.44779963594995564, 13.40000000000000924, -3.600000000000078693 ) ) ;
#82879=PRODUCT_DEFINITION_CONTEXT ( 'detailed design', #173739, 'design' ) ;
#82908=DIRECTION ( 'NONE',  ( -0.000000000000000000, 0.000000000000000000, -1.000000000000000000 ) ) ;
#82980=CARTESIAN_POINT ( 'NONE',  ( -8.752560982291628378, 15.99999996917861189, -9.356054898117346141 ) ) ;
#82982=FACE_OUTER_BOUND ( 'NONE', #149252, .T. ) ;
#82993=ORIENTED_EDGE ( 'NONE', *, *, #43007, .F. ) ;
#83008=UNCERTAINTY_MEASURE_WITH_UNIT (LENGTH_MEASURE( 1.000000000000000082E-05 ), #206182, 'distance_accuracy_value', 'NONE');
#83013=EDGE_CURVE ( 'NONE', #116397, #60282, #1240, .T. ) ;
#83027=ADVANCED_FACE ( 'NONE', ( #16430 ), #197222, .T. ) ;
#83041=FACE_OUTER_BOUND ( 'NONE', #74747, .T. ) ;
#83076=CARTESIAN_POINT ( 'NONE',  ( -9.812680342707254866, 4.108039100808300148, -6.337802944732694677 ) ) ;
#83077=DIRECTION ( 'NONE',  ( 0.000000000000000000, 0.000000000000000000, 1.000000000000000000 ) ) ;
#83104=CARTESIAN_POINT ( 'NONE',  ( 10.18930308530835660, 13.31154919269470760, 7.183432580020707725 ) ) ;
#83115=CARTESIAN_POINT ( 'NONE',  ( 8.790438134619865451, 13.29428800202395955, -8.101059483297394337 ) ) ;
#83122=CARTESIAN_POINT ( 'NONE',  ( 1.734723475976807094E-15, 15.00041888085534758, 12.17999951260719982 ) ) ;
#83136=EDGE_CURVE ( 'NONE', #23505, #21255, #70414, .T. ) ;
#83158=CARTESIAN_POINT ( 'NONE',  ( 11.78331023100045627, 13.87999999999998302, 1.799999999999999600 ) ) ;
#83218=ORIENTED_EDGE ( 'NONE', *, *, #70698, .T. ) ;
#83222=DIRECTION ( 'NONE',  ( 0.000000000000000000, -1.000000000000000000, 0.000000000000000000 ) ) ;
#83254=CARTESIAN_POINT ( 'NONE',  ( -11.78331023100045627, 12.29999999999998295, 1.799999999999999600 ) ) ;
#83266=CARTESIAN_POINT ( 'NONE',  ( -9.508841981786559927, 15.08576114865397244, -7.212865296072072496 ) ) ;
#83279=CARTESIAN_POINT ( 'NONE',  ( 11.44779963594988814, 10.89999999999998082, 3.600000000000001421 ) ) ;
#83280=AXIS2_PLACEMENT_3D ( 'NONE', #170349, #24092, #90196 ) ;
#83309=CYLINDRICAL_SURFACE ( 'NONE', #190924, 0.08000000000000020983 ) ;
#83326=ORIENTED_EDGE ( 'NONE', *, *, #98945, .T. ) ;
#83342=ORIENTED_EDGE ( 'NONE', *, *, #208712, .F. ) ;
#83347=EDGE_CURVE ( 'NONE', #11477, #93554, #160286, .T. ) ;
#83362=EDGE_LOOP ( 'NONE', ( #96102, #136654, #17650, #64483 ) ) ;
#83366=CARTESIAN_POINT ( 'NONE',  ( -9.812993378609343509, 5.211864641514284635, 6.299721592320037367 ) ) ;
#83387=DIRECTION ( 'NONE',  ( -0.000000000000000000, 1.000000000000000000, -0.000000000000000000 ) ) ;
#83397=ADVANCED_FACE ( 'NONE', ( #154322 ), #194912, .T. ) ;
#83406=ORIENTED_EDGE ( 'NONE', *, *, #6564, .T. ) ;
#83422=VERTEX_POINT ( 'NONE', #89334 ) ;
#83439=ADVANCED_FACE ( 'NONE', ( #139146 ), #129310, .T. ) ;
#83458=CARTESIAN_POINT ( 'NONE',  ( 11.43209210103587914, 11.15596075983914481, 3.649125173352121276 ) ) ;
#83513=SURFACE_STYLE_USAGE ( .BOTH. , #181022 ) ;
#83515=CARTESIAN_POINT ( 'NONE',  ( -9.644676237148278375, 5.067654118421841325, 6.575762993896887565 ) ) ;
#83518=UNCERTAINTY_MEASURE_WITH_UNIT (LENGTH_MEASURE( 1.000000000000000082E-05 ), #149343, 'distance_accuracy_value', 'NONE');
#83519=CARTESIAN_POINT ( 'NONE',  ( -1.386567914617391262, 8.090296256147718523, 10.72428812184712932 ) ) ;
#83529=ORIENTED_EDGE ( 'NONE', *, *, #104333, .F. ) ;
#83548=FACE_OUTER_BOUND ( 'NONE', #186720, .T. ) ;
#83555=CARTESIAN_POINT ( 'NONE',  ( -11.96215121607992415, 9.771664462191758105, 0.9565349792967587916 ) ) ;
#83570=DIRECTION ( 'NONE',  ( 0.000000000000000000, -1.000000000000000000, -9.023263958591317418E-17 ) ) ;
#83573=TRIMMED_CURVE ( 'NONE', #176468, ( PARAMETER_VALUE ( 5.355238923655765149 ), #109946 ), ( PARAMETER_VALUE ( 0.000000000000000000 ), #175955 ), .T., .PARAMETER. ) ;
#83603=CARTESIAN_POINT ( 'NONE',  ( 11.96212011828583677, 11.32812445049936656, -0.9569185076418588176 ) ) ;
#83604=VECTOR ( 'NONE', #164604, 1000.000000000000000 ) ;
#83613=EDGE_LOOP ( 'NONE', ( #128513, #101241, #112215, #14162, #109689, #211247, #160379, #77599 ) ) ;
#83632=CIRCLE ( 'NONE', #104508, 0.08000000000000014044 ) ;
#83650=DIRECTION ( 'NONE',  ( 1.000000000000000000, 0.000000000000000000, -0.000000000000000000 ) ) ;
#83661=CARTESIAN_POINT ( 'NONE',  ( 10.32808049211214652, 11.37156981856230686, -7.280726186550563028 ) ) ;
#83686=( GEOMETRIC_REPRESENTATION_CONTEXT ( 3 ) GLOBAL_UNCERTAINTY_ASSIGNED_CONTEXT ( ( #21125 ) ) GLOBAL_UNIT_ASSIGNED_CONTEXT ( ( #138828, #104188, #6655 ) ) REPRESENTATION_CONTEXT ( 'NONE', 'WORKASPACE' ) );
#83706=DIRECTION ( 'NONE',  ( 0.000000000000000000, 1.000000000000000000, 0.000000000000000000 ) ) ;
#83715=CARTESIAN_POINT ( 'NONE',  ( -10.41980074470002648, 5.020554563858687480, 5.279403930596816785 ) ) ;
#83719=CARTESIAN_POINT ( 'NONE',  ( -11.39017651643713869, 6.534219839500422289, 3.782342671282047153 ) ) ;
#83723=MECHANICAL_DESIGN_GEOMETRIC_PRESENTATION_REPRESENTATION('',(#28391),#52801);
#83764=CARTESIAN_POINT ( 'NONE',  ( 0.000000000000000000, 18.91999999999999815, 0.000000000000000000 ) ) ;
#83778=CIRCLE ( 'NONE', #14658, 11.09999999999999964 ) ;
#83813=CARTESIAN_POINT ( 'NONE',  ( -9.351030441618698674, 15.43943296112659880, 7.441731298566530484 ) ) ;
#83814=VERTEX_POINT ( 'NONE', #14448 ) ;
#83820=CARTESIAN_POINT ( 'NONE',  ( 9.472440634255924863, 13.10139178464343424, -7.368143507540152015 ) ) ;
#83824=CARTESIAN_POINT ( 'NONE',  ( 11.89835103415199313, 13.82893085832465552, -1.561208891256347986 ) ) ;
#83828=CARTESIAN_POINT ( 'NONE',  ( 8.370495502396751775, 14.07684108737213080, -8.536638310158815912 ) ) ;
#83835=CARTESIAN_POINT ( 'NONE',  ( 11.80235830595198543, 12.30000000000000071, -1.696088231482801856 ) ) ;
#83855=EDGE_CURVE ( 'NONE', #173182, #171829, #27514, .T. ) ;
#83871=FACE_OUTER_BOUND ( 'NONE', #39026, .T. ) ;
#83881=CARTESIAN_POINT ( 'NONE',  ( -10.50060100873255031, 5.377693802073524765, 5.808388628131299747 ) ) ;
#83884=( NAMED_UNIT ( * ) PLANE_ANGLE_UNIT ( ) SI_UNIT ( $, .RADIAN. ) );
#83898=( NAMED_UNIT ( * ) PLANE_ANGLE_UNIT ( ) SI_UNIT ( $, .RADIAN. ) );
#83914=VERTEX_POINT ( 'NONE', #194285 ) ;
#83956=VERTEX_POINT ( 'NONE', #209444 ) ;
#83959=( BOUNDED_SURFACE ( )  B_SPLINE_SURFACE ( 3, 2, ( 
 ( #126919, #172392, #142047 ),
 ( #27185, #122663, #189689 ),
 ( #192877, #174542, #93291 ),
 ( #73812, #188626, #139906 ),
 ( #107449, #44532, #108515 ),
 ( #156146, #26118, #92229 ) ),
 .UNSPECIFIED., .F., .F., .T. ) 
 B_SPLINE_SURFACE_WITH_KNOTS ( ( 4, 2, 4 ),
 ( 3, 3 ),
 ( 0.000000000000000000, 0.0003831327362561326704, 0.0007662654725122653408 ),
 ( 0.000000000000000000, 1.000000000000000000 ),
 .UNSPECIFIED. ) 
 GEOMETRIC_REPRESENTATION_ITEM ( )  RATIONAL_B_SPLINE_SURFACE ( (
 ( 1.000000000000000000, 0.5879095031487664436, 1.000000000000000000),
 ( 1.000000000000000000, 0.5873691247585943742, 1.000000000000000000),
 ( 1.000000000000000000, 0.6054349545487748285, 1.000000000000000000),
 ( 1.000000000000000000, 0.6533334602776329492, 1.000000000000000000),
 ( 1.000000000000000000, 0.6828746263143679052, 1.000000000000000000),
 ( 1.000000000000000000, 0.7071067811865475727, 1.000000000000000000) ) ) 
 REPRESENTATION_ITEM ( '' )  SURFACE ( )  );
#84021=UNCERTAINTY_MEASURE_WITH_UNIT (LENGTH_MEASURE( 1.000000000000000082E-05 ), #70164, 'distance_accuracy_value', 'NONE');
#84048=EDGE_CURVE ( 'NONE', #14213, #73245, #42279, .T. ) ;
#84050=CARTESIAN_POINT ( 'NONE',  ( 0.6674790882333445641, 16.00000000000000711, -11.66566053519551005 ) ) ;
#84052=CARTESIAN_POINT ( 'NONE',  ( -10.12897898315521061, 6.154003805053667620, 5.673299828594959848 ) ) ;
#84062=DIRECTION ( 'NONE',  ( 0.2150645590070887347, -0.8781765503997437383, 0.4272624273056235267 ) ) ;
#84063=ORIENTED_EDGE ( 'NONE', *, *, #27652, .F. ) ;
#84082=VERTEX_POINT ( 'NONE', #163938 ) ;
#84084=DIRECTION ( 'NONE',  ( 1.000000000000000000, -0.000000000000000000, -0.000000000000000000 ) ) ;
#84087=CARTESIAN_POINT ( 'NONE',  ( 0.000000000000000000, 0.08000000000000020983, 0.000000000000000000 ) ) ;
#84096=DIRECTION ( 'NONE',  ( -0.000000000000000000, -1.000000000000000000, -0.000000000000000000 ) ) ;
#84119=EDGE_CURVE ( 'NONE', #97605, #201490, #97231, .T. ) ;
#84125=CARTESIAN_POINT ( 'NONE',  ( 11.94980361723080264, 10.09761943414563312, -1.099999926404445771 ) ) ;
#84143=COLOUR_RGB ( '', 0.72549020, 0.75294118, 0.79215686) ;
#84148=VERTEX_POINT ( 'NONE', #201724 ) ;
#84154=CARTESIAN_POINT ( 'NONE',  ( -9.420111044277531320, 2.999985932080179829, -6.906458289183190047 ) ) ;
#84165=SURFACE_STYLE_USAGE ( .BOTH. , #186997 ) ;
#84171=CARTESIAN_POINT ( 'NONE',  ( 11.39809020714891830, 7.521243758227223353, 3.778010186578677931 ) ) ;
#84183=CARTESIAN_POINT ( 'NONE',  ( 9.269816152938050280, 13.50982561720567254, -6.801071679830670291 ) ) ;
#84192=CARTESIAN_POINT ( 'NONE',  ( -11.86686399458719343, 12.49071270224662200, 1.056461745586970480 ) ) ;
#84195=ORIENTED_EDGE ( 'NONE', *, *, #123168, .F. ) ;
#84198=DIRECTION ( 'NONE',  ( 1.224643483124941457E-16, 0.002327115863041261980, 0.9999972922622142324 ) ) ;
#84199=CIRCLE ( 'NONE', #60091, 0.07999999999999940492 ) ;
#84208=FILL_AREA_STYLE_COLOUR ( '', #149765 ) ;
#84242=CARTESIAN_POINT ( 'NONE',  ( 11.07790593930098311, 11.29999999999999893, -0.7000000000000009548 ) ) ;
#84284=UNCERTAINTY_MEASURE_WITH_UNIT (LENGTH_MEASURE( 1.000000000000000082E-05 ), #8436, 'distance_accuracy_value', 'NONE');
#84300=( GEOMETRIC_REPRESENTATION_CONTEXT ( 3 ) GLOBAL_UNCERTAINTY_ASSIGNED_CONTEXT ( ( #155432 ) ) GLOBAL_UNIT_ASSIGNED_CONTEXT ( ( #174971, #160837, #107887 ) ) REPRESENTATION_CONTEXT ( 'NONE', 'WORKASPACE' ) );
#84317=CARTESIAN_POINT ( 'NONE',  ( -10.51588623913388254, 11.11317498266430803, -3.554197739806004286 ) ) ;
#84325=EDGE_CURVE ( 'NONE', #182472, #208480, #149001, .T. ) ;
#84334=CARTESIAN_POINT ( 'NONE',  ( -11.97929049433705373, 9.719999999999998863, -0.7046979865771834106 ) ) ;
#84347=CARTESIAN_POINT ( 'NONE',  ( -0.08053691275167716712, 19.00000000000000000, 11.99972973886014316 ) ) ;
#84390=CARTESIAN_POINT ( 'NONE',  ( 8.786015989428143769, 13.41256886957122951, 8.173703117781000671 ) ) ;
#84443=CARTESIAN_POINT ( 'NONE',  ( 9.397848989302721279, 13.71838071990982577, 7.462089927986413684 ) ) ;
#84444=CARTESIAN_POINT ( 'NONE',  ( -11.01135777277262129, 13.39999999999998259, 1.399999999999998579 ) ) ;
#84445=CARTESIAN_POINT ( 'NONE',  ( -10.36733242867369142, 5.031604590660524678, 7.295138277318285347 ) ) ;
#84468=CARTESIAN_POINT ( 'NONE',  ( -11.04724700974751350, 7.053076968211740017, -4.573939983942181264 ) ) ;
#84521=PLANE ( 'NONE',  #82068 ) ;
#84560=FILL_AREA_STYLE ('',( #34733 ) ) ;
#84641=DIRECTION ( 'NONE',  ( 0.000000000000000000, 9.023263958591318651E-17, -1.000000000000000000 ) ) ;
#84647=TOROIDAL_SURFACE ( 'NONE', #153763, 11.92000000000000171, 0.08000000000000000167 ) ;
#84649=CARTESIAN_POINT ( 'NONE',  ( -10.50059885609813115, 5.377696206510352184, -5.808392519734754345 ) ) ;
#84673=AXIS2_PLACEMENT_3D ( 'NONE', #1895, #71168, #152451 ) ;
#84675=CARTESIAN_POINT ( 'NONE',  ( -4.363689859051672393, 15.44735444335154639, -11.13992621954916906 ) ) ;
#84686=CARTESIAN_POINT ( 'NONE',  ( 0.000000000000000000, 11.37999999999998302, 0.000000000000000000 ) ) ;
#84711=ORIENTED_EDGE ( 'NONE', *, *, #87773, .F. ) ;
#84713=VERTEX_POINT ( 'NONE', #162612 ) ;
#84725=CARTESIAN_POINT ( 'NONE',  ( -10.84554942614793127, 5.653270432668692891, -6.476099931950408006 ) ) ;
#84738=CARTESIAN_POINT ( 'NONE',  ( 12.54948750854022954, 7.400697955233512815, 0.9574523190714994136 ) ) ;
#84746=CARTESIAN_POINT ( 'NONE',  ( 11.01135777277262306, 10.09374813218825473, 1.399999999999998579 ) ) ;
#84750=ORIENTED_EDGE ( 'NONE', *, *, #82708, .T. ) ;
#84751=CARTESIAN_POINT ( 'NONE',  ( 11.01135777277262306, 0.000000000000000000, -1.400000000000001910 ) ) ;
#84764=EDGE_CURVE ( 'NONE', #144610, #197667, #135270, .T. ) ;
#84789=CARTESIAN_POINT ( 'NONE',  ( -10.33433454857960321, 4.766519530047388820, -5.444264161973041638 ) ) ;
#84790=DIRECTION ( 'NONE',  ( -0.000000000000000000, -1.000000000000000000, -0.000000000000000000 ) ) ;
#84794=CARTESIAN_POINT ( 'NONE',  ( -12.00015887837301420, 8.029270226016196332, -0.2577645811446898638 ) ) ;
#84838=CARTESIAN_POINT ( 'NONE',  ( 9.192976028328162741, 13.26461296551308600, -9.042127702714923387 ) ) ;
#84855=CARTESIAN_POINT ( 'NONE',  ( -9.671688505580934958, 4.446957226446405009, -7.030662469568692785 ) ) ;
#84867=CARTESIAN_POINT ( 'NONE',  ( -10.78237064342727791, 6.270194388237658956, -4.501389708959286473 ) ) ;
#84892=FILL_AREA_STYLE ('',( #38281 ) ) ;
#84899=CARTESIAN_POINT ( 'NONE',  ( 11.92046840572485777, 13.65252124794270472, -1.382231356234943753 ) ) ;
#84903=CARTESIAN_POINT ( 'NONE',  ( 8.131124540793322808, 14.25330072365142620, -8.765600733912146225 ) ) ;
#84908=CARTESIAN_POINT ( 'NONE',  ( 11.78331023100045627, 9.799999999999982947, 1.799999999999999600 ) ) ;
#84924=LINE ( 'NONE', #182412, #207151 ) ;
#84934=CARTESIAN_POINT ( 'NONE',  ( -6.730704588151846579, 14.55213479732962512, -9.891043484334160141 ) ) ;
#84941=DIRECTION ( 'NONE',  ( 1.000000000000000000, -0.000000000000000000, -0.000000000000000000 ) ) ;
#84953=CARTESIAN_POINT ( 'NONE',  ( -11.15559248640632006, 7.313804510108741219, 4.428430090804268637 ) ) ;
#84970=CARTESIAN_POINT ( 'NONE',  ( 11.33772463945037146, 13.39999999999998259, 3.599999999999999201 ) ) ;
#84999=CARTESIAN_POINT ( 'NONE',  ( -10.42545925421531372, 5.088249681016463022, 5.944232428158755077 ) ) ;
#85004=CIRCLE ( 'NONE', #157703, 11.05000000000000426 ) ;
#85010=DIRECTION ( 'NONE',  ( -0.000000000000000000, 1.000000000000000000, -0.000000000000000000 ) ) ;
#85012=ADVANCED_FACE ( 'NONE', ( #178870 ), #64401, .T. ) ;
#85068=FILL_AREA_STYLE ('',( #200922 ) ) ;
#85069=EDGE_CURVE ( 'NONE', #146971, #188369, #183627, .T. ) ;
#85116=CARTESIAN_POINT ( 'NONE',  ( 0.3263184169964285508, 14.00000000000028955, -11.67999999558625213 ) ) ;
#85118=CARTESIAN_POINT ( 'NONE',  ( -10.99878419127389684, 6.872217442641685103, 3.961452310287494338 ) ) ;
#85120=VERTEX_POINT ( 'NONE', #32596 ) ;
#85125=CIRCLE ( 'NONE', #106056, 0.08000000000000020983 ) ;
#85126=CARTESIAN_POINT ( 'NONE',  ( -1.333449616921166481, 8.249651149236388648, -11.01993490927447716 ) ) ;
#85161=SURFACE_SIDE_STYLE ('',( #152302 ) ) ;
#85163=MECHANICAL_DESIGN_GEOMETRIC_PRESENTATION_REPRESENTATION('',(#178555),#81766);
#85213=ORIENTED_EDGE ( 'NONE', *, *, #206026, .T. ) ;
#85219=CARTESIAN_POINT ( 'NONE',  ( -10.67060214796032724, 5.239869845146935212, -6.813287888368859235 ) ) ;
#85228=FACE_OUTER_BOUND ( 'NONE', #190345, .T. ) ;
#85233=( GEOMETRIC_REPRESENTATION_CONTEXT ( 3 ) GLOBAL_UNCERTAINTY_ASSIGNED_CONTEXT ( ( #149029 ) ) GLOBAL_UNIT_ASSIGNED_CONTEXT ( ( #134807, #83884, #50333 ) ) REPRESENTATION_CONTEXT ( 'NONE', 'WORKASPACE' ) );
#85235=CARTESIAN_POINT ( 'NONE',  ( 11.92009470520713066, 6.690327200924609308, -0.9868518554555439914 ) ) ;
#85246=CARTESIAN_POINT ( 'NONE',  ( 9.266593812803435526, 13.58595580518854362, 6.819388300972848427 ) ) ;
#85249=( BOUNDED_SURFACE ( )  B_SPLINE_SURFACE ( 3, 3, ( 
 ( #131793, #197798, #33177, #99258, #38510, #202031, #51570, #198849, #67766, #133917, #136018, #85118, #69908, #3834, #103513, #151204, #184733, #53691, #199924, #22219, #37436, #104588, #120906, #117695, #170633, #101368, #52622, #119823, #150140, #1712 ),
 ( #21153, #183687, #169572, #35293, #167446, #19040, #2776, #84052, #34234, #185803, #87259, #68846, #634, #132845, #168504, #153323, #4898, #88332, #134966, #200974, #118750, #36359, #102436, #100307, #186878, #54757, #20104, #86191, #70976, #152260 ),
 ( #137086, #203112, #66698, #50496, #116617, #182612, #166373, #17965, #27591, #5974, #42808, #175998, #155460, #125180, #9208, #92627, #76342, #60089, #108916, #26519, #173875, #208457, #205250, #191142, #174938, #142449, #172793, #23300, #24365, #8133 ),
 ( #158670, #154396, #72046, #10267, #126250, #105674, #74219, #204166, #192209, #124123, #156543, #140314, #43871, #190085, #109987, #141395, #56892, #138158, #7043, #73119, #75280, #90477, #207405, #157612, #55821, #206332, #41737, #59024, #139220, #121978 ),
 ( #189021, #123067, #187942, #106765, #171701, #57957, #39572, #107846, #40663, #25448, #89411, #91555, #48141, #160803, #210607, #46003, #78473, #177053, #127323, #64365, #146710, #194360, #93689, #11330, #47069, #80617, #130511, #115308, #128393, #79544 ),
 ( #114254, #212726, #44938, #196498, #211658, #112122, #159731, #180250, #65396, #97953, #63296, #179190, #113186, #95822, #195439, #31874, #12394, #161881, #181298, #77408, #164007, #143525, #94755, #15583, #162942, #81670, #147756, #213774, #131542, #197544 ),
 ( #145662, #30814, #178125, #96893, #111046, #209521, #13468, #29740, #144592, #49189, #62235, #129456, #14523, #28670, #61161, #193294, #100057, #3585, #67518, #84867, #167194, #201791, #17706, #53431, #68592, #37184, #185555, #32925, #54506, #119568 ) ),
 .UNSPECIFIED., .T., .F., .F. ) 
 B_SPLINE_SURFACE_WITH_KNOTS ( ( 4, 3, 4 ),
 ( 4, 2, 2, 2, 2, 2, 2, 2, 2, 2, 2, 2, 2, 2, 4 ),
 ( 0.000000000000000000, 0.5000000000000000000, 1.000000000000000000 ),
 ( 0.3904182756812821231, 0.3921283039710705687, 0.3938383322608589587, 0.3972583888404358499, 0.4040985019995896321, 0.4177787283178971967, 0.4451391809545123257, 0.4999364453639513206, 0.5547656701200603946, 0.5821739285757332460, 0.5958780578035696163, 0.6027301224174878014, 0.6061561547244469494, 0.6078691708779264680, 0.6095821870314059865 ),
 .UNSPECIFIED. ) 
 GEOMETRIC_REPRESENTATION_ITEM ( )  RATIONAL_B_SPLINE_SURFACE ( (
 ( 1.000000000000000000, 1.000000000000000000, 1.000000000000000000, 1.000000000000000000, 1.000000000000000000, 1.000000000000000000, 1.000000000000000000, 1.000000000000000000, 1.000000000000000000, 1.000000000000000000, 1.000000000000000000, 1.000000000000000000, 1.000000000000000000, 1.000000000000000000, 1.000000000000000000, 1.000000000000000000, 1.000000000000000000, 1.000000000000000000, 1.000000000000000000, 1.000000000000000000, 1.000000000000000000, 1.000000000000000000, 1.000000000000000000, 1.000000000000000000, 1.000000000000000000, 1.000000000000000000, 1.000000000000000000, 1.000000000000000000, 1.000000000000000000, 1.000000000000000000),
 ( 0.3333333333333333703, 0.3333333333333333703, 0.3333333333333333703, 0.3333333333333333703, 0.3333333333333333703, 0.3333333333333333703, 0.3333333333333333703, 0.3333333333333333703, 0.3333333333333333703, 0.3333333333333333703, 0.3333333333333333703, 0.3333333333333333703, 0.3333333333333333703, 0.3333333333333333703, 0.3333333333333333703, 0.3333333333333333703, 0.3333333333333333703, 0.3333333333333333703, 0.3333333333333333703, 0.3333333333333333703, 0.3333333333333333703, 0.3333333333333333703, 0.3333333333333333703, 0.3333333333333333703, 0.3333333333333333703, 0.3333333333333333703, 0.3333333333333333703, 0.3333333333333333703, 0.3333333333333333703, 0.3333333333333333703),
 ( 0.3333333333333333703, 0.3333333333333333703, 0.3333333333333333703, 0.3333333333333333703, 0.3333333333333333703, 0.3333333333333333703, 0.3333333333333333703, 0.3333333333333333703, 0.3333333333333333703, 0.3333333333333333703, 0.3333333333333333703, 0.3333333333333333703, 0.3333333333333333703, 0.3333333333333333703, 0.3333333333333333703, 0.3333333333333333703, 0.3333333333333333703, 0.3333333333333333703, 0.3333333333333333703, 0.3333333333333333703, 0.3333333333333333703, 0.3333333333333333703, 0.3333333333333333703, 0.3333333333333333703, 0.3333333333333333703, 0.3333333333333333703, 0.3333333333333333703, 0.3333333333333333703, 0.3333333333333333703, 0.3333333333333333703),
 ( 1.000000000000000000, 1.000000000000000000, 1.000000000000000000, 1.000000000000000000, 1.000000000000000000, 1.000000000000000000, 1.000000000000000000, 1.000000000000000000, 1.000000000000000000, 1.000000000000000000, 1.000000000000000000, 1.000000000000000000, 1.000000000000000000, 1.000000000000000000, 1.000000000000000000, 1.000000000000000000, 1.000000000000000000, 1.000000000000000000, 1.000000000000000000, 1.000000000000000000, 1.000000000000000000, 1.000000000000000000, 1.000000000000000000, 1.000000000000000000, 1.000000000000000000, 1.000000000000000000, 1.000000000000000000, 1.000000000000000000, 1.000000000000000000, 1.000000000000000000),
 ( 0.3333333333333333703, 0.3333333333333333703, 0.3333333333333333703, 0.3333333333333333703, 0.3333333333333333703, 0.3333333333333333703, 0.3333333333333333703, 0.3333333333333333703, 0.3333333333333333703, 0.3333333333333333703, 0.3333333333333333703, 0.3333333333333333703, 0.3333333333333333703, 0.3333333333333333703, 0.3333333333333333703, 0.3333333333333333703, 0.3333333333333333703, 0.3333333333333333703, 0.3333333333333333703, 0.3333333333333333703, 0.3333333333333333703, 0.3333333333333333703, 0.3333333333333333703, 0.3333333333333333703, 0.3333333333333333703, 0.3333333333333333703, 0.3333333333333333703, 0.3333333333333333703, 0.3333333333333333703, 0.3333333333333333703),
 ( 0.3333333333333333703, 0.3333333333333333703, 0.3333333333333333703, 0.3333333333333333703, 0.3333333333333333703, 0.3333333333333333703, 0.3333333333333333703, 0.3333333333333333703, 0.3333333333333333703, 0.3333333333333333703, 0.3333333333333333703, 0.3333333333333333703, 0.3333333333333333703, 0.3333333333333333703, 0.3333333333333333703, 0.3333333333333333703, 0.3333333333333333703, 0.3333333333333333703, 0.3333333333333333703, 0.3333333333333333703, 0.3333333333333333703, 0.3333333333333333703, 0.3333333333333333703, 0.3333333333333333703, 0.3333333333333333703, 0.3333333333333333703, 0.3333333333333333703, 0.3333333333333333703, 0.3333333333333333703, 0.3333333333333333703),
 ( 1.000000000000000000, 1.000000000000000000, 1.000000000000000000, 1.000000000000000000, 1.000000000000000000, 1.000000000000000000, 1.000000000000000000, 1.000000000000000000, 1.000000000000000000, 1.000000000000000000, 1.000000000000000000, 1.000000000000000000, 1.000000000000000000, 1.000000000000000000, 1.000000000000000000, 1.000000000000000000, 1.000000000000000000, 1.000000000000000000, 1.000000000000000000, 1.000000000000000000, 1.000000000000000000, 1.000000000000000000, 1.000000000000000000, 1.000000000000000000, 1.000000000000000000, 1.000000000000000000, 1.000000000000000000, 1.000000000000000000, 1.000000000000000000, 1.000000000000000000) ) ) 
 REPRESENTATION_ITEM ( '' )  SURFACE ( )  );
#85258=CARTESIAN_POINT ( 'NONE',  ( 8.126472743488658779, 14.19519224714456840, -8.830242308825365427 ) ) ;
#85275=( NAMED_UNIT ( * ) PLANE_ANGLE_UNIT ( ) SI_UNIT ( $, .RADIAN. ) );
#85317=ORIENTED_EDGE ( 'NONE', *, *, #23681, .F. ) ;
#85373=CARTESIAN_POINT ( 'NONE',  ( 0.000000000000000000, 7.000000000000000000, 0.000000000000000000 ) ) ;
#85376=CARTESIAN_POINT ( 'NONE',  ( 11.49978884755350172, 12.35729178837194375, 3.429452816445248242 ) ) ;
#85405=ORIENTED_EDGE ( 'NONE', *, *, #193355, .F. ) ;
#85428=( GEOMETRIC_REPRESENTATION_CONTEXT ( 3 ) GLOBAL_UNCERTAINTY_ASSIGNED_CONTEXT ( ( #102698 ) ) GLOBAL_UNIT_ASSIGNED_CONTEXT ( ( #111481, #147129, #12821 ) ) REPRESENTATION_CONTEXT ( 'NONE', 'WORKASPACE' ) );
#85431=CARTESIAN_POINT ( 'NONE',  ( 11.44786932348564079, 13.79999999999998295, 3.303370173849796032 ) ) ;
#85474=EDGE_CURVE ( 'NONE', #50054, #46947, #71762, .T. ) ;
#85519=CARTESIAN_POINT ( 'NONE',  ( -11.55950211276791251, 11.37999999999998302, 3.221476510067112109 ) ) ;
#85559=EDGE_CURVE ( 'NONE', #211752, #129544, #180105, .T. ) ;
#85562=CARTESIAN_POINT ( 'NONE',  ( 0.000000000000000000, 15.00000000000000000, -11.68000000000000149 ) ) ;
#85583=EDGE_CURVE ( 'NONE', #140333, #6177, #104027, .T. ) ;
#85593=CARTESIAN_POINT ( 'NONE',  ( -11.45842088241054135, 12.50693529122955283, -3.566211699757781073 ) ) ;
#85596=ORIENTED_EDGE ( 'NONE', *, *, #59134, .T. ) ;
#85606=FACE_OUTER_BOUND ( 'NONE', #202048, .T. ) ;
#85618=CARTESIAN_POINT ( 'NONE',  ( 11.78331023100045627, 9.799999999999998934, -1.800000000000001155 ) ) ;
#85627=FACE_OUTER_BOUND ( 'NONE', #61029, .T. ) ;
#85642=AXIS2_PLACEMENT_3D ( 'NONE', #212174, #192724, #44378 ) ;
#85655=CARTESIAN_POINT ( 'NONE',  ( -9.812993378609343509, 5.211864641514284635, 6.299721592320037367 ) ) ;
#85658=UNCERTAINTY_MEASURE_WITH_UNIT (LENGTH_MEASURE( 1.000000000000000082E-05 ), #35766, 'distance_accuracy_value', 'NONE');
#85659=DIRECTION ( 'NONE',  ( 0.000000000000000000, 0.000000000000000000, 1.000000000000000000 ) ) ;
#85689=FILL_AREA_STYLE ('',( #139804 ) ) ;
#85708=DIRECTION ( 'NONE',  ( 0.000000000000000000, 0.000000000000000000, -1.000000000000000000 ) ) ;
#85710=FACE_OUTER_BOUND ( 'NONE', #79193, .T. ) ;
#85742=CARTESIAN_POINT ( 'NONE',  ( 11.94105721839855505, 11.02698343341124243, -1.187919402540330127 ) ) ;
#85745=VECTOR ( 'NONE', #211089, 1000.000000000000000 ) ;
#85774=CARTESIAN_POINT ( 'NONE',  ( -11.33772463945036968, 12.59088423488573660, -3.600000000000000977 ) ) ;
#85776=CARTESIAN_POINT ( 'NONE',  ( -1.734723475976807094E-15, 4.518467169708414666, -11.92000000000000171 ) ) ;
#85782=ORIENTED_EDGE ( 'NONE', *, *, #157408, .F. ) ;
#85796=CARTESIAN_POINT ( 'NONE',  ( -10.52284260640670688, 5.420240069097000735, -5.071998063130033430 ) ) ;
#85819=COLOUR_RGB ( '', 0.66274510, 0.83137255, 0.94901961) ;
#85821=CARTESIAN_POINT ( 'NONE',  ( 11.97929049433705551, 12.30000000000000071, -0.7046979865771820783 ) ) ;
#85827=LINE ( 'NONE', #135657, #77713 ) ;
#85860=LINE ( 'NONE', #18707, #5613 ) ;
#85864=CARTESIAN_POINT ( 'NONE',  ( -11.01510031751075758, 5.354170659035768942, -4.767690450682862568 ) ) ;
#85874=CIRCLE ( 'NONE', #61759, 0.07999999999999998779 ) ;
#85878=B_SPLINE_CURVE_WITH_KNOTS ( 'NONE', 3,
 ( #156064, #170164, #87860, #71581, #73737, #139834 ),
 .UNSPECIFIED., .F., .F.,
 ( 4, 2, 4 ),
 ( 0.000000000000000000, 0.0003258677429877279035, 0.0006517354859754558071 ),
 .UNSPECIFIED. ) ;
#85880=ORIENTED_EDGE ( 'NONE', *, *, #2314, .F. ) ;
#85910=CARTESIAN_POINT ( 'NONE',  ( 7.209650745910531455, 13.96317866693702925, -9.185143276789457190 ) ) ;
#85928=CARTESIAN_POINT ( 'NONE',  ( 11.97929049433705373, 13.88000000000000078, -0.7046979865771834106 ) ) ;
#85931=( BOUNDED_SURFACE ( )  B_SPLINE_SURFACE ( 3, 3, ( 
 ( #75665, #141772, #59407, #37830, #103908, #71368, #78841, #176368, #192588, #97257, #46369, #43189, #160109, #175311, #13835, #112488, #93002, #162248, #27975, #163311, #113560, #212029, #208838, #62594, #147076, #94069, #109302, #44243, #110364, #63672, #213097, #11712, #146018, #126625, #29048, #194730, #178498, #77786, #125563, #79910, #14892, #31184 ),
 ( #143907, #80987, #209900, #129826, #144961, #61538, #195808, #191524, #127704, #76715, #60468, #193664, #47444, #12766, #177430, #45307, #26898, #30108, #159046, #111426, #210966, #128757, #96199, #179563, #10639, #142831, #95131, #161180, #35425, #1840, #51702, #198972, #130870, #197919, #83104, #32237, #102573, #152393, #20236, #86321, #49546, #118883 ),
 ( #167573, #33294, #181667, #200053, #84183, #64727, #115672, #17027, #182742, #98309, #149184, #50617, #166503, #151335, #67899, #34360, #99378, #760, #165431, #131910, #66827, #132970, #116742, #48503, #100433, #15958, #117825, #18095, #150271, #65764, #2904, #36495, #134043, #82041, #148135, #183815, #135095, #101503, #19172, #85246, #114622, #68976 ),
 ( #201108, #52749, #184869, #168633, #164373, #196865, #180613, #214136, #192067, #158529, #208321, #141254, #70039, #140169, #25313, #185935, #44803, #94620, #176913, #28529, #206191, #61024, #175860, #9070, #109846, #189949, #123981, #142311, #26378, #3971, #57819, #173735, #125046, #37570, #91414, #207262, #108776, #93546, #156400, #107709, #10126, #76201 ),
 ( #191001, #59952, #126107, #43732, #27448, #7988, #159590, #119960, #143381, #136155, #74077, #106625, #127185, #58892, #157475, #42668, #11189, #77269, #209380, #193153, #174802, #110907, #202172, #53830, #172654, #24229, #92491, #41598, #75144, #90331, #81541, #78336, #195302, #210462, #49055, #147623, #128259, #197414, #211525, #132468, #148684, #32796 ),
 ( #212595, #115176, #63160, #13335, #111988, #181171, #213642, #252, #129325, #66324, #62100, #98870, #14386, #161743, #96758, #164922, #179056, #95689, #46932, #64233, #162809, #182226, #160663, #177990, #80478, #16515, #79409, #113050, #198471, #33849, #48006, #146577, #114124, #130376, #194221, #45866, #50116, #145526, #180116, #29603, #30675, #82598 ),
 ( #196366, #31741, #97814, #163878, #116236, #15453, #12259, #65268, #144458, #131414, #100977, #99930, #83661, #168127, #187565, #154016, #5582, #149751, #152942, #2390, #135638, #84738, #167066, #184359, #165992, #86875, #70591, #68468, #67390, #151888, #54382, #134595, #18658, #51179, #120520, #4518, #71662, #150827, #103130, #69531, #200596, #52243 ) ),
 .UNSPECIFIED., .T., .F., .T. ) 
 B_SPLINE_SURFACE_WITH_KNOTS ( ( 4, 3, 4 ),
 ( 4, 2, 2, 2, 2, 2, 2, 2, 2, 2, 2, 2, 2, 2, 2, 2, 2, 2, 2, 2, 4 ),
 ( 0.000000000000000000, 0.5000000000000000000, 1.000000000000000000 ),
 ( 0.2451329569378435380, 0.2471230096987881431, 0.2491130624597327203, 0.2530931679816219027, 0.2610533790254002673, 0.2769738011129569966, 0.3088146452880705106, 0.3724963336382974832, 0.4043793557688165619, 0.4362623778993356405, 0.5000489545690223192, 0.5638291548596064962, 0.5957026119297792466, 0.6275760689999518860, 0.6912196958168144167, 0.7230415092252455711, 0.7389524159294611483, 0.7469078692815689369, 0.7508855959576228312, 0.7528744592956497783, 0.7548633226336768365 ),
 .UNSPECIFIED. ) 
 GEOMETRIC_REPRESENTATION_ITEM ( )  RATIONAL_B_SPLINE_SURFACE ( (
 ( 1.000000000000000000, 1.000000000000000000, 1.000000000000000000, 1.000000000000000000, 1.000000000000000000, 1.000000000000000000, 1.000000000000000000, 1.000000000000000000, 1.000000000000000000, 1.000000000000000000, 1.000000000000000000, 1.000000000000000000, 1.000000000000000000, 1.000000000000000000, 1.000000000000000000, 1.000000000000000000, 1.000000000000000000, 1.000000000000000000, 1.000000000000000000, 1.000000000000000000, 1.000000000000000000, 1.000000000000000000, 1.000000000000000000, 1.000000000000000000, 1.000000000000000000, 1.000000000000000000, 1.000000000000000000, 1.000000000000000000, 1.000000000000000000, 1.000000000000000000, 1.000000000000000000, 1.000000000000000000, 1.000000000000000000, 1.000000000000000000, 1.000000000000000000, 1.000000000000000000, 1.000000000000000000, 1.000000000000000000, 1.000000000000000000, 1.000000000000000000, 1.000000000000000000, 1.000000000000000000),
 ( 0.3333333333333333703, 0.3333333333333333703, 0.3333333333333333703, 0.3333333333333333703, 0.3333333333333333703, 0.3333333333333333703, 0.3333333333333333703, 0.3333333333333333703, 0.3333333333333333703, 0.3333333333333333703, 0.3333333333333333703, 0.3333333333333333703, 0.3333333333333333703, 0.3333333333333333703, 0.3333333333333333703, 0.3333333333333333703, 0.3333333333333333703, 0.3333333333333333703, 0.3333333333333333703, 0.3333333333333333703, 0.3333333333333333703, 0.3333333333333333703, 0.3333333333333333703, 0.3333333333333333703, 0.3333333333333333703, 0.3333333333333333703, 0.3333333333333333703, 0.3333333333333333703, 0.3333333333333333703, 0.3333333333333333703, 0.3333333333333333703, 0.3333333333333333703, 0.3333333333333333703, 0.3333333333333333703, 0.3333333333333333703, 0.3333333333333333703, 0.3333333333333333703, 0.3333333333333333703, 0.3333333333333333703, 0.3333333333333333703, 0.3333333333333333703, 0.3333333333333333703),
 ( 0.3333333333333333703, 0.3333333333333333703, 0.3333333333333333703, 0.3333333333333333703, 0.3333333333333333703, 0.3333333333333333703, 0.3333333333333333703, 0.3333333333333333703, 0.3333333333333333703, 0.3333333333333333703, 0.3333333333333333703, 0.3333333333333333703, 0.3333333333333333703, 0.3333333333333333703, 0.3333333333333333703, 0.3333333333333333703, 0.3333333333333333703, 0.3333333333333333703, 0.3333333333333333703, 0.3333333333333333703, 0.3333333333333333703, 0.3333333333333333703, 0.3333333333333333703, 0.3333333333333333703, 0.3333333333333333703, 0.3333333333333333703, 0.3333333333333333703, 0.3333333333333333703, 0.3333333333333333703, 0.3333333333333333703, 0.3333333333333333703, 0.3333333333333333703, 0.3333333333333333703, 0.3333333333333333703, 0.3333333333333333703, 0.3333333333333333703, 0.3333333333333333703, 0.3333333333333333703, 0.3333333333333333703, 0.3333333333333333703, 0.3333333333333333703, 0.3333333333333333703),
 ( 1.000000000000000000, 1.000000000000000000, 1.000000000000000000, 1.000000000000000000, 1.000000000000000000, 1.000000000000000000, 1.000000000000000000, 1.000000000000000000, 1.000000000000000000, 1.000000000000000000, 1.000000000000000000, 1.000000000000000000, 1.000000000000000000, 1.000000000000000000, 1.000000000000000000, 1.000000000000000000, 1.000000000000000000, 1.000000000000000000, 1.000000000000000000, 1.000000000000000000, 1.000000000000000000, 1.000000000000000000, 1.000000000000000000, 1.000000000000000000, 1.000000000000000000, 1.000000000000000000, 1.000000000000000000, 1.000000000000000000, 1.000000000000000000, 1.000000000000000000, 1.000000000000000000, 1.000000000000000000, 1.000000000000000000, 1.000000000000000000, 1.000000000000000000, 1.000000000000000000, 1.000000000000000000, 1.000000000000000000, 1.000000000000000000, 1.000000000000000000, 1.000000000000000000, 1.000000000000000000),
 ( 0.3333333333333333703, 0.3333333333333333703, 0.3333333333333333703, 0.3333333333333333703, 0.3333333333333333703, 0.3333333333333333703, 0.3333333333333333703, 0.3333333333333333703, 0.3333333333333333703, 0.3333333333333333703, 0.3333333333333333703, 0.3333333333333333703, 0.3333333333333333703, 0.3333333333333333703, 0.3333333333333333703, 0.3333333333333333703, 0.3333333333333333703, 0.3333333333333333703, 0.3333333333333333703, 0.3333333333333333703, 0.3333333333333333703, 0.3333333333333333703, 0.3333333333333333703, 0.3333333333333333703, 0.3333333333333333703, 0.3333333333333333703, 0.3333333333333333703, 0.3333333333333333703, 0.3333333333333333703, 0.3333333333333333703, 0.3333333333333333703, 0.3333333333333333703, 0.3333333333333333703, 0.3333333333333333703, 0.3333333333333333703, 0.3333333333333333703, 0.3333333333333333703, 0.3333333333333333703, 0.3333333333333333703, 0.3333333333333333703, 0.3333333333333333703, 0.3333333333333333703),
 ( 0.3333333333333333703, 0.3333333333333333703, 0.3333333333333333703, 0.3333333333333333703, 0.3333333333333333703, 0.3333333333333333703, 0.3333333333333333703, 0.3333333333333333703, 0.3333333333333333703, 0.3333333333333333703, 0.3333333333333333703, 0.3333333333333333703, 0.3333333333333333703, 0.3333333333333333703, 0.3333333333333333703, 0.3333333333333333703, 0.3333333333333333703, 0.3333333333333333703, 0.3333333333333333703, 0.3333333333333333703, 0.3333333333333333703, 0.3333333333333333703, 0.3333333333333333703, 0.3333333333333333703, 0.3333333333333333703, 0.3333333333333333703, 0.3333333333333333703, 0.3333333333333333703, 0.3333333333333333703, 0.3333333333333333703, 0.3333333333333333703, 0.3333333333333333703, 0.3333333333333333703, 0.3333333333333333703, 0.3333333333333333703, 0.3333333333333333703, 0.3333333333333333703, 0.3333333333333333703, 0.3333333333333333703, 0.3333333333333333703, 0.3333333333333333703, 0.3333333333333333703),
 ( 1.000000000000000000, 1.000000000000000000, 1.000000000000000000, 1.000000000000000000, 1.000000000000000000, 1.000000000000000000, 1.000000000000000000, 1.000000000000000000, 1.000000000000000000, 1.000000000000000000, 1.000000000000000000, 1.000000000000000000, 1.000000000000000000, 1.000000000000000000, 1.000000000000000000, 1.000000000000000000, 1.000000000000000000, 1.000000000000000000, 1.000000000000000000, 1.000000000000000000, 1.000000000000000000, 1.000000000000000000, 1.000000000000000000, 1.000000000000000000, 1.000000000000000000, 1.000000000000000000, 1.000000000000000000, 1.000000000000000000, 1.000000000000000000, 1.000000000000000000, 1.000000000000000000, 1.000000000000000000, 1.000000000000000000, 1.000000000000000000, 1.000000000000000000, 1.000000000000000000, 1.000000000000000000, 1.000000000000000000, 1.000000000000000000, 1.000000000000000000, 1.000000000000000000, 1.000000000000000000) ) ) 
 REPRESENTATION_ITEM ( '' )  SURFACE ( )  );
#85959=CARTESIAN_POINT ( 'NONE',  ( 1.734723475976807094E-15, 15.00041888085534758, 12.17999951260719982 ) ) ;
#85960=CARTESIAN_POINT ( 'NONE',  ( -9.386399775572158433, 15.51845911145272083, 7.476390437876971440 ) ) ;
#85975=FACE_OUTER_BOUND ( 'NONE', #46093, .T. ) ;
#85980=CARTESIAN_POINT ( 'NONE',  ( 11.86239285000045918, 12.22000000000000064, -1.812080536912753059 ) ) ;
#85985=TOROIDAL_SURFACE ( 'NONE', #200065, 12.18000000000000149, 0.5000000000000008882 ) ;
#86025=CARTESIAN_POINT ( 'NONE',  ( -11.04592006821611427, 7.049318325634454041, 4.577072995540873102 ) ) ;
#86039=AXIS2_PLACEMENT_3D ( 'NONE', #102513, #22295, #120987 ) ;
#86040=CARTESIAN_POINT ( 'NONE',  ( -11.94105721237522921, 10.07259215598210567, -1.187919463087249605 ) ) ;
#86081=CARTESIAN_POINT ( 'NONE',  ( -9.348561386512724170, 4.000007913748541810, -7.001914023932275910 ) ) ;
#86095=ADVANCED_FACE ( 'NONE', ( #42256 ), #23833, .F. ) ;
#86120=DIRECTION ( 'NONE',  ( -0.000000000000000000, -1.000000000000000000, -0.000000000000000000 ) ) ;
#86143=FILL_AREA_STYLE_COLOUR ( '', #19403 ) ;
#86164=UNCERTAINTY_MEASURE_WITH_UNIT (LENGTH_MEASURE( 1.000000000000000082E-05 ), #137126, 'distance_accuracy_value', 'NONE');
#86189=CARTESIAN_POINT ( 'NONE',  ( -9.117697077653634352, 15.00000000001154987, -7.299999999986293453 ) ) ;
#86191=CARTESIAN_POINT ( 'NONE',  ( -9.997720234198379075, 5.662301760159435204, -5.943093865039206669 ) ) ;
#86199=DIRECTION ( 'NONE',  ( 0.8594130494132222742, -0.03761243564701257508, -0.5098965730253202100 ) ) ;
#86206=ORIENTED_EDGE ( 'NONE', *, *, #128408, .T. ) ;
#86230=FACE_BOUND ( 'NONE', #123787, .T. ) ;
#86239=ADVANCED_FACE ( 'NONE', ( #195957 ), #78989, .F. ) ;
#86242=MECHANICAL_DESIGN_GEOMETRIC_PRESENTATION_REPRESENTATION('',(#158924),#24073);
#86257=ORIENTED_EDGE ( 'NONE', *, *, #80161, .F. ) ;
#86267=DIRECTION ( 'NONE',  ( -0.000000000000000000, 1.000000000000000000, -0.000000000000000000 ) ) ;
#86291=CARTESIAN_POINT ( 'NONE',  ( -11.97181073603049839, 11.37999999999999901, -0.8318477717169578955 ) ) ;
#86294=CARTESIAN_POINT ( 'NONE',  ( -10.20559888102932256, 5.000029895416906456, -7.525687786258633771 ) ) ;
#86309=CARTESIAN_POINT ( 'NONE',  ( 10.37552651436754836, 9.126834862229522116, 6.082233718396662603 ) ) ;
#86313=ORIENTED_EDGE ( 'NONE', *, *, #203350, .F. ) ;
#86321=CARTESIAN_POINT ( 'NONE',  ( 10.14216661378989848, 13.64382096325071458, 7.299002950830796088 ) ) ;
#86334=CARTESIAN_POINT ( 'NONE',  ( -0.9037479196795165093, 15.51845925029282114, -11.99999999996284750 ) ) ;
#86376=VECTOR ( 'NONE', #99325, 1000.000000000000000 ) ;
#86396=CYLINDRICAL_SURFACE ( 'NONE', #191345, 0.07999999999999998779 ) ;
#86454=B_SPLINE_CURVE_WITH_KNOTS ( 'NONE', 3,
 ( #41298, #107406, #142008, #177680, #125808, #190702 ),
 .UNSPECIFIED., .F., .F.,
 ( 4, 2, 4 ),
 ( 0.000000000000000000, 0.0003844267940947831432, 0.0007688535881895662864 ),
 .UNSPECIFIED. ) ;
#86484=CARTESIAN_POINT ( 'NONE',  ( -10.52942622947605145, 3.950194995956630262, -5.760434021238635793 ) ) ;
#86500=CARTESIAN_POINT ( 'NONE',  ( 11.41381675112453387, 13.39999999999998259, 3.704697986577180302 ) ) ;
#86539=DIRECTION ( 'NONE',  ( 0.000000000000000000, 1.000000000000000000, 0.000000000000000000 ) ) ;
#86565=CARTESIAN_POINT ( 'NONE',  ( 11.01135777277262306, 13.39999999999998259, 1.399999999999998579 ) ) ;
#86581=CARTESIAN_POINT ( 'NONE',  ( -10.39320420135713263, 4.932286138528427344, 5.331284845095887626 ) ) ;
#86612=EDGE_LOOP ( 'NONE', ( #69232, #31671, #36432, #206982 ) ) ;
#86646=CARTESIAN_POINT ( 'NONE',  ( -11.86687215968023601, 11.10942212305781851, 1.056395335932115209 ) ) ;
#86649=ORIENTED_EDGE ( 'NONE', *, *, #88601, .T. ) ;
#86659=CARTESIAN_POINT ( 'NONE',  ( -11.78331023100045627, 13.79999999999999893, -1.800000000000001155 ) ) ;
#86663=DIRECTION ( 'NONE',  ( 0.000000000000000000, 0.000000000000000000, 1.000000000000000000 ) ) ;
#86694=ADVANCED_FACE ( 'NONE', ( #198671 ), #164081, .F. ) ;
#86724=CARTESIAN_POINT ( 'NONE',  ( -10.14895191633106819, 4.000000000000000888, 7.601392964450660372 ) ) ;
#86725=EDGE_LOOP ( 'NONE', ( #154569, #100035, #41332, #132631, #132417, #125052, #153336, #48162 ) ) ;
#86734=AXIS2_PLACEMENT_3D ( 'NONE', #63443, #194501, #144736 ) ;
#86738=VERTEX_POINT ( 'NONE', #35112 ) ;
#86756=CARTESIAN_POINT ( 'NONE',  ( -6.777498110814238252, 15.51954974125004760, 9.912810906811193590 ) ) ;
#86763=EDGE_LOOP ( 'NONE', ( #94330, #97182, #79423, #99705 ) ) ;
#86778=CARTESIAN_POINT ( 'NONE',  ( -10.53033573153658153, 3.951415937214838525, -5.758770635485034539 ) ) ;
#86784=DIRECTION ( 'NONE',  ( 0.8003905296791066215, 0.000000000000000000, -0.5994789404140892231 ) ) ;
#86792=STYLED_ITEM ( 'NONE', ( #137643 ), #70312 ) ;
#86796=MECHANICAL_DESIGN_GEOMETRIC_PRESENTATION_REPRESENTATION('',(#180192),#52166);
#86810=CARTESIAN_POINT ( 'NONE',  ( -5.969155412111654790, 15.44727373956653693, -10.36857180707296244 ) ) ;
#86826=FACE_BOUND ( 'NONE', #55845, .T. ) ;
#86832=SURFACE_STYLE_FILL_AREA ( #5540 ) ;
#86850=VERTEX_POINT ( 'NONE', #153147 ) ;
#86852=ORIENTED_EDGE ( 'NONE', *, *, #147049, .T. ) ;
#86863=CARTESIAN_POINT ( 'NONE',  ( -10.91675076000969113, 4.673595418013491987, -4.467283485442433921 ) ) ;
#86868=CARTESIAN_POINT ( 'NONE',  ( 11.89942855770814312, 12.30000000000000071, -0.7000000000000009548 ) ) ;
#86875=CARTESIAN_POINT ( 'NONE',  ( 11.72719273365024506, 8.694648967210921953, 4.374500150831954315 ) ) ;
#86889=TOROIDAL_SURFACE ( 'NONE', #111078, 12.17999999982603576, 0.5000000000000008882 ) ;
#86891=CARTESIAN_POINT ( 'NONE',  ( -15.75000000000000000, 10.19999999999999929, 1.099999999999996758 ) ) ;
#86931=CARTESIAN_POINT ( 'NONE',  ( 11.35605497252127449, 9.985818540483530015, 3.553547709190206572 ) ) ;
#86952=EDGE_CURVE ( 'NONE', #131029, #141526, #70797, .T. ) ;
#86974=CARTESIAN_POINT ( 'NONE',  ( 9.599742726594369557, 13.73983281947659840, -8.263962686181493211 ) ) ;
#87004=CARTESIAN_POINT ( 'NONE',  ( 9.100780844468317810, 14.29763700255456449, -7.752528009982434298 ) ) ;
#87022=CARTESIAN_POINT ( 'NONE',  ( 0.000000000000000000, 14.55305236562705318, 0.000000000000000000 ) ) ;
#87023=CARTESIAN_POINT ( 'NONE',  ( -9.333041836230234978, 15.44694763438833540, 7.472413793097425483 ) ) ;
#87027=PLANE ( 'NONE',  #210080 ) ;
#87033=CARTESIAN_POINT ( 'NONE',  ( 11.86145016429273191, 10.90000000000000036, -1.100000000000002087 ) ) ;
#87036=AXIS2_PLACEMENT_3D ( 'NONE', #89263, #172643, #71898 ) ;
#87079=CARTESIAN_POINT ( 'NONE',  ( -11.86145016429273191, 11.00587876334730453, 1.099999999999996758 ) ) ;
#87080=CARTESIAN_POINT ( 'NONE',  ( -10.89183333199790304, 4.909323612238608803, -5.036858318171157478 ) ) ;
#87089=CARTESIAN_POINT ( 'NONE',  ( -11.40611951520848955, 7.885036337628656078, 3.737597762133503920 ) ) ;
#87093=CIRCLE ( 'NONE', #173713, 0.08000000000000019595 ) ;
#87095=ORIENTED_EDGE ( 'NONE', *, *, #98624, .F. ) ;
#87104=DIRECTION ( 'NONE',  ( 0.000000000000000000, -1.000000000000000000, 0.000000000000000000 ) ) ;
#87105=DIRECTION ( 'NONE',  ( 0.000000000000000000, 0.000000000000000000, -1.000000000000000000 ) ) ;
#87143=CARTESIAN_POINT ( 'NONE',  ( -11.81293272228161229, 8.718537709414365011, -2.131821593364598755 ) ) ;
#87144=LINE ( 'NONE', #90363, #158278 ) ;
#87149=TOROIDAL_SURFACE ( 'NONE', #128691, 12.18000000000000149, 0.5000000000000008882 ) ;
#87182=( BOUNDED_SURFACE ( )  B_SPLINE_SURFACE ( 3, 2, ( 
 ( #91876, #111364, #194667 ),
 ( #193605, #174192, #192525 ),
 ( #44179, #157932, #173114 ),
 ( #144902, #94007, #90798 ),
 ( #8448, #127640, #11650 ),
 ( #177369, #75597, #24695 ) ),
 .UNSPECIFIED., .F., .F., .F. ) 
 B_SPLINE_SURFACE_WITH_KNOTS ( ( 4, 2, 4 ),
 ( 3, 3 ),
 ( -4.336808689942017736E-19, 0.0003831416164015013842, 0.0007662832328030032020 ),
 ( 0.000000000000000000, 1.000000000000000000 ),
 .UNSPECIFIED. ) 
 GEOMETRIC_REPRESENTATION_ITEM ( )  RATIONAL_B_SPLINE_SURFACE ( (
 ( 1.000000000000000000, 0.7071067811865475727, 1.000000000000000000),
 ( 1.000000000000000000, 0.6829713513657061918, 1.000000000000000000),
 ( 1.000000000000000000, 0.6534833722367423547, 1.000000000000000000),
 ( 1.000000000000000000, 0.6054027484667425796, 1.000000000000000000),
 ( 1.000000000000000000, 0.5875453974411385394, 1.000000000000000000),
 ( 1.000000000000000000, 0.5879095031487528988, 1.000000000000000000) ) ) 
 REPRESENTATION_ITEM ( '' )  SURFACE ( )  );
#87184=DIRECTION ( 'NONE',  ( 0.000000000000000000, 0.000000000000000000, 1.000000000000000000 ) ) ;
#87204=PLANE ( 'NONE',  #182270 ) ;
#87207=( NAMED_UNIT ( * ) PLANE_ANGLE_UNIT ( ) SI_UNIT ( $, .RADIAN. ) );
#87215=CARTESIAN_POINT ( 'NONE',  ( 6.928203230275525648, 15.00000000000000000, -9.797958971132702644 ) ) ;
#87259=CARTESIAN_POINT ( 'NONE',  ( -10.37105062950515943, 6.927298630606520291, 5.133691221222295376 ) ) ;
#87267=FACE_OUTER_BOUND ( 'NONE', #136710, .T. ) ;
#87324=EDGE_CURVE ( 'NONE', #16328, #131029, #174472, .T. ) ;
#87347=MECHANICAL_DESIGN_GEOMETRIC_PRESENTATION_REPRESENTATION('',(#104674),#142739);
#87367=CARTESIAN_POINT ( 'NONE',  ( -10.44369633504468631, 5.112959841837462882, -5.232137017608346596 ) ) ;
#87377=FACE_OUTER_BOUND ( 'NONE', #163109, .T. ) ;
#87384=CARTESIAN_POINT ( 'NONE',  ( 11.70591049654802696, 7.005752292624462640, -2.417405326248005082 ) ) ;
#87410=CARTESIAN_POINT ( 'NONE',  ( -8.171050030069373804, 15.51987628351127313, -8.834037170385874660 ) ) ;
#87411=ORIENTED_EDGE ( 'NONE', *, *, #57852, .F. ) ;
#87412=ORIENTED_EDGE ( 'NONE', *, *, #208952, .T. ) ;
#87438=DIRECTION ( 'NONE',  ( -0.000000000000000000, 0.000000000000000000, -1.000000000000000000 ) ) ;
#87450=VECTOR ( 'NONE', #70067, 1000.000000000000000 ) ;
#87452=CARTESIAN_POINT ( 'NONE',  ( 11.86145016429272836, 10.90000000000000036, 1.179999999999997051 ) ) ;
#87472=AXIS2_PLACEMENT_3D ( 'NONE', #169091, #32698, #4427 ) ;
#87473=DIRECTION ( 'NONE',  ( 0.000000000000000000, 1.000000000000000000, 0.000000000000000000 ) ) ;
#87489=AXIS2_PLACEMENT_3D ( 'NONE', #213813, #36144, #118540 ) ;
#87500=B_SPLINE_CURVE_WITH_KNOTS ( 'NONE', 3,
 ( #141933, #46540, #207946, #92104, #96369, #75826 ),
 .UNSPECIFIED., .F., .F.,
 ( 4, 2, 4 ),
 ( 0.000000000000000000, 0.0003844267940947825469, 0.0007688535881895650938 ),
 .UNSPECIFIED. ) ;
#87555=CYLINDRICAL_SURFACE ( 'NONE', #147805, 0.3999999999999997446 ) ;
#87568=( LENGTH_UNIT ( ) NAMED_UNIT ( * ) SI_UNIT ( .MILLI., .METRE. ) );
#87570=DIRECTION ( 'NONE',  ( 0.000000000000000000, 0.000000000000000000, -1.000000000000000000 ) ) ;
#87595=EDGE_CURVE ( 'NONE', #90065, #53890, #58213, .T. ) ;
#87634=AXIS2_PLACEMENT_3D ( 'NONE', #56315, #158097, #173281 ) ;
#87647=CARTESIAN_POINT ( 'NONE',  ( 11.80235830595197655, 13.79999999999998295, 1.696088231482818065 ) ) ;
#87653=PLANE ( 'NONE',  #58462 ) ;
#87687=( LENGTH_UNIT ( ) NAMED_UNIT ( * ) SI_UNIT ( .MILLI., .METRE. ) );
#87699=FILL_AREA_STYLE ('',( #170006 ) ) ;
#87700=CARTESIAN_POINT ( 'NONE',  ( -11.89942855770814134, 11.29999999999999893, 0.6999999999999992895 ) ) ;
#87757=DIRECTION ( 'NONE',  ( 0.000000000000000000, -0.000000000000000000, 1.000000000000000000 ) ) ;
#87771=ORIENTED_EDGE ( 'NONE', *, *, #172633, .T. ) ;
#87773=EDGE_CURVE ( 'NONE', #120419, #183827, #159103, .T. ) ;
#87786=( NAMED_UNIT ( * ) PLANE_ANGLE_UNIT ( ) SI_UNIT ( $, .RADIAN. ) );
#87792=CARTESIAN_POINT ( 'NONE',  ( -10.43059486372414568, 5.377696206510353072, -5.769669902936525929 ) ) ;
#87795=CARTESIAN_POINT ( 'NONE',  ( -9.510677803526956353, 3.006766436585398772, 6.782528980676592489 ) ) ;
#87819=CARTESIAN_POINT ( 'NONE',  ( -0.008622056139523381901, 15.44694768828586540, 11.95585894197802013 ) ) ;
#87828=CARTESIAN_POINT ( 'NONE',  ( -9.608184375698545665, 14.88196915126796327, -7.189074558220958089 ) ) ;
#87836=CARTESIAN_POINT ( 'NONE',  ( -11.94105721237523099, 10.19999999999999929, 1.187919463087248273 ) ) ;
#87848=CARTESIAN_POINT ( 'NONE',  ( -10.30143037061213285, 3.720351604917702115, -6.155881949090546534 ) ) ;
#87860=CARTESIAN_POINT ( 'NONE',  ( 11.35605497252127272, 13.61418145951645542, -3.553547709190210124 ) ) ;
#87865=CARTESIAN_POINT ( 'NONE',  ( 9.367496997597598352, 4.518459255872631530, 7.500000000000000000 ) ) ;
#87889=ADVANCED_FACE ( 'NONE', ( #85228 ), #168615, .F. ) ;
#87912=CARTESIAN_POINT ( 'NONE',  ( -1.499999999999946709, 7.750000000000000000, 15.75000000000000711 ) ) ;
#87915=ORIENTED_EDGE ( 'NONE', *, *, #108416, .T. ) ;
#87929=CYLINDRICAL_SURFACE ( 'NONE', #24772, 0.3999999999999997446 ) ;
#87930=CARTESIAN_POINT ( 'NONE',  ( -10.52284959769361805, 5.420271152154175986, 5.071911021504272199 ) ) ;
#87946=VERTEX_POINT ( 'NONE', #103632 ) ;
#87951=CARTESIAN_POINT ( 'NONE',  ( -10.62873463776380056, 13.79999999999998295, 3.199999999999997957 ) ) ;
#87967=EDGE_CURVE ( 'NONE', #15788, #84713, #140256, .T. ) ;
#87984=FACE_OUTER_BOUND ( 'NONE', #164895, .T. ) ;
#87988=AXIS2_PLACEMENT_3D ( 'NONE', #80726, #64473, #111158 ) ;
#87990=ADVANCED_FACE ( 'NONE', ( #87377 ), #79579, .T. ) ;
#87997=SURFACE_SIDE_STYLE ('',( #184410 ) ) ;
#88024=DIRECTION ( 'NONE',  ( -0.9982742078614211811, 0.000000000000000000, -0.05872483221476467591 ) ) ;
#88061=CARTESIAN_POINT ( 'NONE',  ( 10.50000000000000178, 12.59159113040219857, -3.600000000000000977 ) ) ;
#88084=B_SPLINE_CURVE_WITH_KNOTS ( 'NONE', 3,
 ( #197868, #98262, #184810, #182685, #81992, #130824 ),
 .UNSPECIFIED., .F., .F.,
 ( 4, 2, 4 ),
 ( 0.000000000000000000, 0.0003155923098472861849, 0.0006311846196945723698 ),
 .UNSPECIFIED. ) ;
#88095=CARTESIAN_POINT ( 'NONE',  ( 9.276214967470513884, 13.85813420416141639, 7.540790294154477991 ) ) ;
#88104=DIRECTION ( 'NONE',  ( -0.000000000000000000, -1.000000000000000000, -0.000000000000000000 ) ) ;
#88113=DIRECTION ( 'NONE',  ( 0.000000000000000000, 0.000000000000000000, 1.000000000000000000 ) ) ;
#88116=ORIENTED_EDGE ( 'NONE', *, *, #13918, .T. ) ;
#88143=EDGE_CURVE ( 'NONE', #19657, #125687, #208203, .T. ) ;
#88144=LINE ( 'NONE', #55636, #28262 ) ;
#88162=DIRECTION ( 'NONE',  ( 7.993605777301127091E-15, 0.000000000000000000, -1.000000000000000000 ) ) ;
#88169=B_SPLINE_CURVE_WITH_KNOTS ( 'NONE', 3,
 ( #177308, #146960, #212975, #195689, #97142, #28923 ),
 .UNSPECIFIED., .F., .F.,
 ( 4, 2, 4 ),
 ( 0.001259240562161249421, 0.001573673787268791650, 0.001888107012376333878 ),
 .UNSPECIFIED. ) ;
#88207=DIRECTION ( 'NONE',  ( 1.000000000000000000, -0.000000000000000000, -0.000000000000000000 ) ) ;
#88217=CARTESIAN_POINT ( 'NONE',  ( -11.75716154505269984, 8.610272713044158976, -2.418301517245814658 ) ) ;
#88274=( GEOMETRIC_REPRESENTATION_CONTEXT ( 3 ) GLOBAL_UNCERTAINTY_ASSIGNED_CONTEXT ( ( #205743 ) ) GLOBAL_UNIT_ASSIGNED_CONTEXT ( ( #183504, #146783, #82806 ) ) REPRESENTATION_CONTEXT ( 'NONE', 'WORKASPACE' ) );
#88279=( NAMED_UNIT ( * ) PLANE_ANGLE_UNIT ( ) SI_UNIT ( $, .RADIAN. ) );
#88282=CARTESIAN_POINT ( 'NONE',  ( -11.01135777277261951, 13.50500854530268668, -1.400000000000001465 ) ) ;
#88290=( GEOMETRIC_REPRESENTATION_CONTEXT ( 3 ) GLOBAL_UNCERTAINTY_ASSIGNED_CONTEXT ( ( #187420 ) ) GLOBAL_UNIT_ASSIGNED_CONTEXT ( ( #37613, #200092, #169743 ) ) REPRESENTATION_CONTEXT ( 'NONE', 'WORKASPACE' ) );
#88293=( LENGTH_UNIT ( ) NAMED_UNIT ( * ) SI_UNIT ( .MILLI., .METRE. ) );
#88300=CARTESIAN_POINT ( 'NONE',  ( 9.598595877357185557, 13.73909624707286703, 8.266025096903813818 ) ) ;
#88332=CARTESIAN_POINT ( 'NONE',  ( -10.78552488895401318, 8.017604977416297629, -4.042330561003328881 ) ) ;
#88343=EDGE_LOOP ( 'NONE', ( #96611, #212600, #106632, #111696, #202836, #72194, #132243, #174640 ) ) ;
#88361=ORIENTED_EDGE ( 'NONE', *, *, #141283, .T. ) ;
#88372=( NAMED_UNIT ( * ) PLANE_ANGLE_UNIT ( ) SI_UNIT ( $, .RADIAN. ) );
#88388=CARTESIAN_POINT ( 'NONE',  ( 11.89942855770813956, 9.719999999999998863, 0.6999999999999992895 ) ) ;
#88445=CARTESIAN_POINT ( 'NONE',  ( -11.38600250725030172, 3.712543481068769857, -5.706073308245968256 ) ) ;
#88455=( NAMED_UNIT ( * ) SI_UNIT ( $, .STERADIAN. ) SOLID_ANGLE_UNIT ( ) );
#88461=CARTESIAN_POINT ( 'NONE',  ( 11.84810327283921261, 6.845834857362776305, 1.964380509715618617 ) ) ;
#88466=EDGE_LOOP ( 'NONE', ( #67113, #185577, #60749, #138654 ) ) ;
#88471=EDGE_LOOP ( 'NONE', ( #131813, #37446, #18724, #78876, #40193, #194449, #142303, #58502 ) ) ;
#88480=CARTESIAN_POINT ( 'NONE',  ( 0.000000000000000000, 0.08000000000000020983, 11.09999999999999964 ) ) ;
#88527=CARTESIAN_POINT ( 'NONE',  ( 11.86145016429273014, 13.50587876334730453, -1.100000000000000089 ) ) ;
#88531=CARTESIAN_POINT ( 'NONE',  ( -9.928285507789787800, 5.423409019249701757, -6.081825614513333811 ) ) ;
#88544=DIRECTION ( 'NONE',  ( 0.000000000000000000, 0.000000000000000000, -1.000000000000000000 ) ) ;
#88585=VECTOR ( 'NONE', #24684, 1000.000000000000000 ) ;
#88601=EDGE_CURVE ( 'NONE', #137788, #45474, #96493, .T. ) ;
#88614=CARTESIAN_POINT ( 'NONE',  ( -11.89942855770814134, 13.79999999999999893, -0.7000000000000009548 ) ) ;
#88622=FILL_AREA_STYLE ('',( #74496 ) ) ;
#88623=( NAMED_UNIT ( * ) SI_UNIT ( $, .STERADIAN. ) SOLID_ANGLE_UNIT ( ) );
#88631=CYLINDRICAL_SURFACE ( 'NONE', #71689, 0.07999999999999998779 ) ;
#88646=CARTESIAN_POINT ( 'NONE',  ( 7.220996296834734096, 15.51845925587262798, -9.590923008284281792 ) ) ;
#88652=CARTESIAN_POINT ( 'NONE',  ( 11.41108574530292863, 13.75836855377623635, 3.405883542057587476 ) ) ;
#88668=( BOUNDED_SURFACE ( )  B_SPLINE_SURFACE ( 3, 2, ( 
 ( #3251, #117094, #164719 ),
 ( #118166, #183094, #184152 ),
 ( #49907, #150619, #182014 ),
 ( #19516, #85593, #35775 ),
 ( #33645, #152730, #70383 ),
 ( #69319, #16308, #165791 ) ),
 .UNSPECIFIED., .F., .F., .F. ) 
 B_SPLINE_SURFACE_WITH_KNOTS ( ( 4, 2, 4 ),
 ( 3, 3 ),
 ( -4.065758146820641628E-19, 0.0003831416164015016010, 0.0007662832328030036357 ),
 ( 0.000000000000000000, 1.000000000000000000 ),
 .UNSPECIFIED. ) 
 GEOMETRIC_REPRESENTATION_ITEM ( )  RATIONAL_B_SPLINE_SURFACE ( (
 ( 1.000000000000000000, 0.7071067811865475727, 1.000000000000000000),
 ( 1.000000000000000000, 0.6829713513656306967, 1.000000000000000000),
 ( 1.000000000000000000, 0.6534833722368420528, 1.000000000000000000),
 ( 1.000000000000000000, 0.6054027484666428816, 1.000000000000000000),
 ( 1.000000000000000000, 0.5875453974412017111, 1.000000000000000000),
 ( 1.000000000000000000, 0.5879095031487528988, 1.000000000000000000) ) ) 
 REPRESENTATION_ITEM ( '' )  SURFACE ( )  );
#88694=EDGE_CURVE ( 'NONE', #131029, #48008, #115961, .T. ) ;
#88715=CARTESIAN_POINT ( 'NONE',  ( -11.91826848676304884, 10.09166292761251071, 1.400000051402189971 ) ) ;
#88730=CARTESIAN_POINT ( 'NONE',  ( 0.005207752244010266374, 14.55743561439478739, 11.94812378735272240 ) ) ;
#88731=FILL_AREA_STYLE_COLOUR ( '', #127669 ) ;
#88732=CARTESIAN_POINT ( 'NONE',  ( -9.470186914265017464, 4.005096909781187264, 6.837150237413082365 ) ) ;
#88746=CARTESIAN_POINT ( 'NONE',  ( -1.499999999999961364, 8.500000000000000000, 10.64483442802188762 ) ) ;
#88769=CARTESIAN_POINT ( 'NONE',  ( 10.50000000000000178, 10.19999999999999929, -3.600000000000000977 ) ) ;
#88778=ORIENTED_EDGE ( 'NONE', *, *, #64050, .F. ) ;
#88787=CARTESIAN_POINT ( 'NONE',  ( -11.86145016429273014, 10.90000000000000036, 1.179999999999997051 ) ) ;
#88801=ORIENTED_EDGE ( 'NONE', *, *, #11908, .T. ) ;
#88822=AXIS2_PLACEMENT_3D ( 'NONE', #14359, #63133, #175831 ) ;
#88831=CARTESIAN_POINT ( 'NONE',  ( -0.8448260811288544891, 15.46906395968185244, 12.00404981830694240 ) ) ;
#88844=CARTESIAN_POINT ( 'NONE',  ( 11.92619526913699879, 10.90000000000000036, -1.328859060402686199 ) ) ;
#88845=CARTESIAN_POINT ( 'NONE',  ( 9.905435134813219022, 11.51422724318055835, -6.695335200864244385 ) ) ;
#88850=CARTESIAN_POINT ( 'NONE',  ( 11.92619526913699879, 12.69999999999998153, 1.328859060402684644 ) ) ;
#88851=CIRCLE ( 'NONE', #92276, 0.07999999999999943268 ) ;
#88868=FILL_AREA_STYLE ('',( #22750 ) ) ;
#88879=CARTESIAN_POINT ( 'NONE',  ( -10.71692179555930302, 5.308633586712264041, 6.728550107195007790 ) ) ;
#88919=AXIS2_PLACEMENT_3D ( 'NONE', #205200, #188966, #92577 ) ;
#88931=CARTESIAN_POINT ( 'NONE',  ( 11.89942855770813956, 12.22000000000000064, -0.7000000000000009548 ) ) ;
#88932=DIRECTION ( 'NONE',  ( -0.7806247497998004548, 0.000000000000000000, 0.6249999999999992228 ) ) ;
#88937=CARTESIAN_POINT ( 'NONE',  ( -11.92619526913699879, 10.19999999999998153, 1.328859060402684644 ) ) ;
#88963=CARTESIAN_POINT ( 'NONE',  ( -15.75000000000000000, 12.30000000000000071, -3.200000000000001510 ) ) ;
#88970=CARTESIAN_POINT ( 'NONE',  ( -11.97929049433705373, 13.88000000000000078, -0.7046979865771834106 ) ) ;
#88979=TOROIDAL_SURFACE ( 'NONE', #123692, 11.92000000000000171, 0.08000000000000000167 ) ;
#88994=DIRECTION ( 'NONE',  ( -1.000000000000000000, 0.000000000000000000, 0.000000000000000000 ) ) ;
#88996=CARTESIAN_POINT ( 'NONE',  ( -11.84668730067608600, 12.69999999999999929, -1.400000000000001910 ) ) ;
#88999=EDGE_LOOP ( 'NONE', ( #208004, #12948, #48055, #11541 ) ) ;
#89006=EDGE_CURVE ( 'NONE', #118697, #172216, #5355, .T. ) ;
#89014=CARTESIAN_POINT ( 'NONE',  ( -10.92050379694822837, 4.688480456342538183, -4.459762147120462039 ) ) ;
#89015=STYLED_ITEM ( 'NONE', ( #61594 ), #198182 ) ;
#89028=CARTESIAN_POINT ( 'NONE',  ( 11.97929049433705551, 12.29999999999999716, 0.7046979865771803020 ) ) ;
#89033=DIRECTION ( 'NONE',  ( -0.9632918427306580433, 0.000000000000000000, -0.2684563758389303945 ) ) ;
#89037=CARTESIAN_POINT ( 'NONE',  ( 11.01135777277262306, 10.19999999999998153, 1.399999999999998579 ) ) ;
#89043=DIRECTION ( 'NONE',  ( 1.000000000000000000, -0.000000000000000000, -0.000000000000000000 ) ) ;
#89047=( GEOMETRIC_REPRESENTATION_CONTEXT ( 3 ) GLOBAL_UNCERTAINTY_ASSIGNED_CONTEXT ( ( #14236 ) ) GLOBAL_UNIT_ASSIGNED_CONTEXT ( ( #133148, #183987, #166685 ) ) REPRESENTATION_CONTEXT ( 'NONE', 'WORKASPACE' ) );
#89049=LINE ( 'NONE', #155106, #56995 ) ;
#89080=FILL_AREA_STYLE ('',( #188691 ) ) ;
#89104=ORIENTED_EDGE ( 'NONE', *, *, #201250, .F. ) ;
#89126=CARTESIAN_POINT ( 'NONE',  ( 8.721781227551465676, 14.89250699912923537, 8.248177467968419663 ) ) ;
#89127=ORIENTED_EDGE ( 'NONE', *, *, #158166, .F. ) ;
#89152=AXIS2_PLACEMENT_3D ( 'NONE', #184667, #86120, #203041 ) ;
#89179=DIRECTION ( 'NONE',  ( 0.000000000000000000, 1.000000000000000000, 0.000000000000000000 ) ) ;
#89187=CARTESIAN_POINT ( 'NONE',  ( -10.45911050446410506, 5.175404930453152197, 5.201426885097844455 ) ) ;
#89192=CARTESIAN_POINT ( 'NONE',  ( -9.333041836229170940, 14.55305236563267535, -7.472413793097618218 ) ) ;
#89237=CARTESIAN_POINT ( 'NONE',  ( -11.88234649872613602, 12.34339217083249096, 0.9090484974825225883 ) ) ;
#89263=CARTESIAN_POINT ( 'NONE',  ( 0.000000000000000000, 13.79999999999998295, 0.000000000000000000 ) ) ;
#89278=ORIENTED_EDGE ( 'NONE', *, *, #3774, .T. ) ;
#89279=CARTESIAN_POINT ( 'NONE',  ( -1.797304815382257948, 14.48004927659174257, -11.89862588508291275 ) ) ;
#89298=( LENGTH_UNIT ( ) NAMED_UNIT ( * ) SI_UNIT ( .MILLI., .METRE. ) );
#89308=AXIS2_PLACEMENT_3D ( 'NONE', #118942, #54947, #185991 ) ;
#89315=CARTESIAN_POINT ( 'NONE',  ( 11.92619526913699879, 12.57218333338757077, -1.328859060402686199 ) ) ;
#89334=CARTESIAN_POINT ( 'NONE',  ( -10.44369633504468631, 5.112959841837461994, -5.232137017608345708 ) ) ;
#89349=CIRCLE ( 'NONE', #210390, 0.08000000000000040412 ) ;
#89362=( NAMED_UNIT ( * ) PLANE_ANGLE_UNIT ( ) SI_UNIT ( $, .RADIAN. ) );
#89374=CARTESIAN_POINT ( 'NONE',  ( 8.523031442321446605, 14.76712986476217715, -9.394111251778250349 ) ) ;
#89376=CARTESIAN_POINT ( 'NONE',  ( 9.180878539475957112, 14.08084533201349586, 6.958356306020501592 ) ) ;
#89411=CARTESIAN_POINT ( 'NONE',  ( -12.06798728936711385, 5.701251286509326555, 4.345411722927631004 ) ) ;
#89451=CARTESIAN_POINT ( 'NONE',  ( -15.75000000000000000, 10.90000000000000036, -1.800000000000001155 ) ) ;
#89467=VECTOR ( 'NONE', #71050, 1000.000000000000000 ) ;
#89503=AXIS2_PLACEMENT_3D ( 'NONE', #128671, #127611, #114530 ) ;
#89530=CARTESIAN_POINT ( 'NONE',  ( -11.03376256896084584, 6.348997720274319079, -6.086949085616508270 ) ) ;
#89536=CARTESIAN_POINT ( 'NONE',  ( 8.998985659026871531, 12.36178301847608196, 7.871464661039776267 ) ) ;
#89538=ORIENTED_EDGE ( 'NONE', *, *, #137200, .F. ) ;
#89552=EDGE_CURVE ( 'NONE', #187716, #169055, #19036, .T. ) ;
#89574=CARTESIAN_POINT ( 'NONE',  ( 9.367496997597598352, 3.530917816115240804, 7.500000000000001776 ) ) ;
#89600=( LENGTH_UNIT ( ) NAMED_UNIT ( * ) SI_UNIT ( .MILLI., .METRE. ) );
#89605=CARTESIAN_POINT ( 'NONE',  ( -11.29167836119662738, 5.103960725615834804, -5.764738477843053488 ) ) ;
#89653=MECHANICAL_DESIGN_GEOMETRIC_PRESENTATION_REPRESENTATION('',(#162299),#65481);
#89670=EDGE_CURVE ( 'NONE', #152119, #139854, #112366, .T. ) ;
#89672=DIRECTION ( 'NONE',  ( 1.000000000000000000, -0.000000000000000000, -0.000000000000000000 ) ) ;
#89674=EDGE_CURVE ( 'NONE', #109578, #16927, #98810, .T. ) ;
#89706=( NAMED_UNIT ( * ) PLANE_ANGLE_UNIT ( ) SI_UNIT ( $, .RADIAN. ) );
#89710=( BOUNDED_SURFACE ( )  B_SPLINE_SURFACE ( 3, 2, ( 
 ( #104418, #156373, #140139 ),
 ( #92461, #171536, #41567 ),
 ( #158500, #22052, #157446 ),
 ( #10099, #72959, #76173 ),
 ( #142279, #208289, #59922 ),
 ( #187779, #105504, #56729 ) ),
 .UNSPECIFIED., .F., .F., .F. ) 
 B_SPLINE_SURFACE_WITH_KNOTS ( ( 4, 2, 4 ),
 ( 3, 3 ),
 ( 0.000000000000000000, 0.0003831327362561331041, 0.0007662654725122662082 ),
 ( 0.000000000000000000, 1.000000000000000000 ),
 .UNSPECIFIED. ) 
 GEOMETRIC_REPRESENTATION_ITEM ( )  RATIONAL_B_SPLINE_SURFACE ( (
 ( 1.000000000000000000, 0.5879095031487548972, 1.000000000000000000),
 ( 1.000000000000000000, 0.5873691247577044194, 1.000000000000000000),
 ( 1.000000000000000000, 0.6054349545499626561, 1.000000000000000000),
 ( 1.000000000000000000, 0.6533334602764224730, 1.000000000000000000),
 ( 1.000000000000000000, 0.6828746263152811746, 1.000000000000000000),
 ( 1.000000000000000000, 0.7071067811865475727, 1.000000000000000000) ) ) 
 REPRESENTATION_ITEM ( '' )  SURFACE ( )  );
#89725=CARTESIAN_POINT ( 'NONE',  ( 8.625358771641339573, 15.01266977653634349, -8.344411790353040814 ) ) ;
#89727=FACE_OUTER_BOUND ( 'NONE', #40135, .T. ) ;
#89749=CARTESIAN_POINT ( 'NONE',  ( 6.882015208740349443, 15.51887838114830132, 9.732639244658489730 ) ) ;
#89762=EDGE_CURVE ( 'NONE', #186645, #62746, #71080, .T. ) ;
#89771=DIRECTION ( 'NONE',  ( -0.7806247497998005658, 0.000000000000000000, -0.6249999999999988898 ) ) ;
#89784=DIRECTION ( 'NONE',  ( 0.000000000000000000, 1.804652791718263484E-16, -1.000000000000000000 ) ) ;
#89809=CARTESIAN_POINT ( 'NONE',  ( -11.97302537858639759, 13.79875989808050107, 0.8111997896468257085 ) ) ;
#89811=CARTESIAN_POINT ( 'NONE',  ( -11.60067993250125262, 4.148157162114866736, 5.314938114050354656 ) ) ;
#89844=CARTESIAN_POINT ( 'NONE',  ( 11.88168509644349058, 11.37999999999998302, 1.685788023084328513 ) ) ;
#89847=( LENGTH_UNIT ( ) NAMED_UNIT ( * ) SI_UNIT ( .MILLI., .METRE. ) );
#89852=EDGE_LOOP ( 'NONE', ( #103379, #136560, #45580, #179973 ) ) ;
#89871=( LENGTH_UNIT ( ) NAMED_UNIT ( * ) SI_UNIT ( .MILLI., .METRE. ) );
#89873=FACE_OUTER_BOUND ( 'NONE', #137185, .T. ) ;
#89884=ORIENTED_EDGE ( 'NONE', *, *, #89762, .F. ) ;
#89902=CARTESIAN_POINT ( 'NONE',  ( -6.739446930247193990, 15.46990418895350849, 9.939002560225588923 ) ) ;
#89916=DIRECTION ( 'NONE',  ( -0.000000000000000000, -1.000000000000000000, -0.000000000000000000 ) ) ;
#89927=ORIENTED_EDGE ( 'NONE', *, *, #95972, .F. ) ;
#89940=SURFACE_STYLE_FILL_AREA ( #172246 ) ;
#89948=CARTESIAN_POINT ( 'NONE',  ( -0.07968937631781032593, 15.51803367805782052, 11.99973206003984139 ) ) ;
#89949=CARTESIAN_POINT ( 'NONE',  ( -11.23957921816311512, 4.929848952671569862, 5.866464787178605533 ) ) ;
#89997=CARTESIAN_POINT ( 'NONE',  ( -8.148229011229679131, 14.52979931989257523, 8.855646333722853925 ) ) ;
#90000=CARTESIAN_POINT ( 'NONE',  ( -11.48243876534946040, 9.799999999999998934, -3.200000000000001510 ) ) ;
#90002=CARTESIAN_POINT ( 'NONE',  ( -11.84668730067608422, 10.89999999999998259, 1.399999999999998357 ) ) ;
#90028=CARTESIAN_POINT ( 'NONE',  ( 11.87815913191726480, 11.30307820631413307, 1.708869976696563597 ) ) ;
#90049=EDGE_CURVE ( 'NONE', #44585, #20115, #91603, .T. ) ;
#90065=VERTEX_POINT ( 'NONE', #122132 ) ;
#90066=ORIENTED_EDGE ( 'NONE', *, *, #211523, .F. ) ;
#90073=CARTESIAN_POINT ( 'NONE',  ( 11.01135777277262484, 13.50498644914894086, -1.400000000000001243 ) ) ;
#90080=CARTESIAN_POINT ( 'NONE',  ( -10.44369227015510404, 5.112964020592957404, 5.232143560358708534 ) ) ;
#90081=EDGE_CURVE ( 'NONE', #66250, #105059, #209157, .T. ) ;
#90083=CARTESIAN_POINT ( 'NONE',  ( 9.644012019580303630, 13.59213021077435535, 8.211487644058824031 ) ) ;
#90085=CARTESIAN_POINT ( 'NONE',  ( -9.305047017617200211, 15.51845925588232333, -7.449999999995526423 ) ) ;
#90093=CARTESIAN_POINT ( 'NONE',  ( -9.508009452559559094, 15.00000000000599343, 7.612499999990692601 ) ) ;
#90102=CARTESIAN_POINT ( 'NONE',  ( -11.45846087878769559, 13.59311600781440887, -3.566076377698187194 ) ) ;
#90138=ORIENTED_EDGE ( 'NONE', *, *, #17565, .F. ) ;
#90145=CYLINDRICAL_SURFACE ( 'NONE', #119520, 0.3999999999999993006 ) ;
#90149=CARTESIAN_POINT ( 'NONE',  ( 11.01135777277262306, 10.19999999999998153, 1.399999999999998579 ) ) ;
#90156=CARTESIAN_POINT ( 'NONE',  ( 11.78331023100045627, 12.22000000000000064, -1.800000000000001155 ) ) ;
#90169=DIRECTION ( 'NONE',  ( 0.000000000000000000, 0.000000000000000000, -1.000000000000000000 ) ) ;
#90174=AXIS2_PLACEMENT_3D ( 'NONE', #127244, #195357, #209440 ) ;
#90193=CARTESIAN_POINT ( 'NONE',  ( 9.181860203497647532, 14.16078059704854653, 7.658820650071877623 ) ) ;
#90196=DIRECTION ( 'NONE',  ( 0.000000000000000000, -7.228014483236694583E-17, 1.000000000000000000 ) ) ;
#90247=CARTESIAN_POINT ( 'NONE',  ( -10.45142682343936791, 5.144546645612242841, 5.216777551074719632 ) ) ;
#90251=CARTESIAN_POINT ( 'NONE',  ( -4.797639982484825261, 14.48151998951723662, -11.00824919581360817 ) ) ;
#90311=DIRECTION ( 'NONE',  ( -0.9982742078614211811, 0.000000000000000000, -0.05872483221476467591 ) ) ;
#90331=CARTESIAN_POINT ( 'NONE',  ( 9.227664502431396798, 10.66305660167662595, 7.832549530788790015 ) ) ;
#90350=PRODUCT_DEFINITION_FORMATION_WITH_SPECIFIED_SOURCE ( 'ANY', '', #59182, .NOT_KNOWN. ) ;
#90355=VECTOR ( 'NONE', #1999, 1000.000000000000000 ) ;
#90363=CARTESIAN_POINT ( 'NONE',  ( -11.01135777277262129, 0.000000000000000000, -1.400000000000001910 ) ) ;
#90387=DIRECTION ( 'NONE',  ( -7.993605777301127091E-15, 0.000000000000000000, 1.000000000000000000 ) ) ;
#90390=CARTESIAN_POINT ( 'NONE',  ( 0.3554123170485725680, 15.00000000000058265, 12.67999999502907649 ) ) ;
#90434=DIRECTION ( 'NONE',  ( -0.000000000000000000, 1.000000000000000000, 1.804652791718263484E-16 ) ) ;
#90441=CARTESIAN_POINT ( 'NONE',  ( 7.017272423055321617, 15.99342652349251104, 9.336217528587633652 ) ) ;
#90449=UNCERTAINTY_MEASURE_WITH_UNIT (LENGTH_MEASURE( 1.000000000000000082E-05 ), #102775, 'distance_accuracy_value', 'NONE');
#90477=CARTESIAN_POINT ( 'NONE',  ( -11.47191357686926771, 5.776505007901941546, -5.393588192467421827 ) ) ;
#90494=CARTESIAN_POINT ( 'NONE',  ( -10.45361012356095465, 5.194925941179032058, 5.800590495124775536 ) ) ;
#90498=ORIENTED_EDGE ( 'NONE', *, *, #36673, .T. ) ;
#90515=FACE_BOUND ( 'NONE', #154877, .T. ) ;
#90516=( LENGTH_UNIT ( ) NAMED_UNIT ( * ) SI_UNIT ( .MILLI., .METRE. ) );
#90517=CARTESIAN_POINT ( 'NONE',  ( 1.369155121446740960E-15, 0.08000000000000020983, -11.18000000000000149 ) ) ;
#90518=MECHANICAL_DESIGN_GEOMETRIC_PRESENTATION_REPRESENTATION('',(#14408),#163185);
#90542=FILL_AREA_STYLE_COLOUR ( '', #182740 ) ;
#90551=( BOUNDED_SURFACE ( )  B_SPLINE_SURFACE ( 3, 2, ( 
 ( #106640, #125062, #138034 ),
 ( #189965, #25330, #204047 ),
 ( #58908, #208339, #9086 ),
 ( #41614, #107726, #8003 ),
 ( #55697, #75160, #74094 ),
 ( #93564, #6922, #72999 ),
 ( #42686, #141270, #108793 ),
 ( #156416, #43749, #26395 ),
 ( #92508, #121853, #40537 ),
 ( #187824, #172668, #158545 ) ),
 .UNSPECIFIED., .F., .F., .T. ) 
 B_SPLINE_SURFACE_WITH_KNOTS ( ( 4, 2, 2, 2, 4 ),
 ( 3, 3 ),
 ( -6.776263578034402713E-19, 0.0004030251014121639832, 0.0008060502028243286170, 0.001209075304236493197, 0.001612100405648657885 ),
 ( 0.000000000000000000, 1.000000000000000000 ),
 .UNSPECIFIED. ) 
 GEOMETRIC_REPRESENTATION_ITEM ( )  RATIONAL_B_SPLINE_SURFACE ( (
 ( 1.000000000000000000, 0.8509629433967621503, 1.000000000000000000),
 ( 1.000000000000000000, 0.8510310118808769309, 1.000000000000000000),
 ( 1.000000000000000000, 0.8495812529563572246, 1.000000000000000000),
 ( 1.000000000000000000, 0.8465918360525789277, 1.000000000000000000),
 ( 1.000000000000000000, 0.8452340365386274978, 1.000000000000000000),
 ( 1.000000000000000000, 0.8452309425927184705, 1.000000000000000000),
 ( 1.000000000000000000, 0.8465710739603070634, 1.000000000000000000),
 ( 1.000000000000000000, 0.8495952187152705504, 1.000000000000000000),
 ( 1.000000000000000000, 0.8510135196387130785, 1.000000000000000000),
 ( 1.000000000000000000, 0.8509629433966219292, 1.000000000000000000) ) ) 
 REPRESENTATION_ITEM ( '' )  SURFACE ( )  );
#90591=ORIENTED_EDGE ( 'NONE', *, *, #25088, .F. ) ;
#90597=CARTESIAN_POINT ( 'NONE',  ( -11.50790213655337979, 7.746734403679841563, -4.957264960544601529 ) ) ;
#90603=CARTESIAN_POINT ( 'NONE',  ( 8.126867821905964462, 14.19425889842085375, 8.829897715376826994 ) ) ;
#90625=CARTESIAN_POINT ( 'NONE',  ( -11.41381675112453387, 10.89999999999998259, 3.704697986577180746 ) ) ;
#90666=( NAMED_UNIT ( * ) SI_UNIT ( $, .STERADIAN. ) SOLID_ANGLE_UNIT ( ) );
#90671=CARTESIAN_POINT ( 'NONE',  ( -10.96415609372974131, 4.387140345944800401, -6.371816014364277692 ) ) ;
#90679=ORIENTED_EDGE ( 'NONE', *, *, #213686, .F. ) ;
#90720=CIRCLE ( 'NONE', #66381, 11.09999999999999964 ) ;
#90728=VERTEX_POINT ( 'NONE', #20997 ) ;
#90767=VERTEX_POINT ( 'NONE', #192042 ) ;
#90771=CARTESIAN_POINT ( 'NONE',  ( -11.94105721237523277, 19.00000000000000000, 1.187919463087248273 ) ) ;
#90780=EDGE_LOOP ( 'NONE', ( #61181, #42085, #92063, #74776 ) ) ;
#90786=CARTESIAN_POINT ( 'NONE',  ( 6.743451144134843922, 15.00000000000000000, -9.536680065235831449 ) ) ;
#90787=CARTESIAN_POINT ( 'NONE',  ( 7.504827820433121133, 15.48994999688346574, -9.370061686304214987 ) ) ;
#90798=CARTESIAN_POINT ( 'NONE',  ( 11.43190902327452108, 9.944778717421318248, 3.649704988378163595 ) ) ;
#90851=CARTESIAN_POINT ( 'NONE',  ( -11.33772463945037323, 10.09097530385347774, 3.599999999999998312 ) ) ;
#90852=CARTESIAN_POINT ( 'NONE',  ( -11.84668730067608600, 10.19999999999998153, 1.399999999999998357 ) ) ;
#90862=DIRECTION ( 'NONE',  ( -0.000000000000000000, -1.000000000000000000, -0.000000000000000000 ) ) ;
#90867=CARTESIAN_POINT ( 'NONE',  ( -11.94105721839851952, 13.52698343341134191, 1.187919402540718927 ) ) ;
#90868=AXIS2_PLACEMENT_3D ( 'NONE', #113586, #13860, #149209 ) ;
#90869=CARTESIAN_POINT ( 'NONE',  ( -10.57368757801325820, 3.061359382655743033, 7.009609602318408683 ) ) ;
#90884=CIRCLE ( 'NONE', #160126, 0.08000000000000020983 ) ;
#90897=CARTESIAN_POINT ( 'NONE',  ( -5.991201117307169532, 15.51884043567246962, -10.40697266434820634 ) ) ;
#90899=MECHANICAL_DESIGN_GEOMETRIC_PRESENTATION_REPRESENTATION('',(#73555),#94468);
#90908=LINE ( 'NONE', #140747, #15596 ) ;
#90913=ORIENTED_EDGE ( 'NONE', *, *, #175999, .F. ) ;
#90921=CARTESIAN_POINT ( 'NONE',  ( -3.529886618686457478, 14.55202822082756065, 11.43118357259692708 ) ) ;
#90932=DIRECTION ( 'NONE',  ( 1.000000000000000000, -0.000000000000000000, -0.000000000000000000 ) ) ;
#90947=EDGE_CURVE ( 'NONE', #204424, #80409, #101935, .T. ) ;
#90964=CARTESIAN_POINT ( 'NONE',  ( -6.714337407434930682, 15.44785316226682603, 9.902284344783144121 ) ) ;
#90973=DIRECTION ( 'NONE',  ( 0.000000000000000000, 0.000000000000000000, -1.000000000000000000 ) ) ;
#90978=DIRECTION ( 'NONE',  ( 0.000000000000000000, 0.000000000000000000, 1.000000000000000000 ) ) ;
#91013=CARTESIAN_POINT ( 'NONE',  ( -0.01853512708398871028, 15.45720132225713961, 11.97163374478179243 ) ) ;
#91014=CARTESIAN_POINT ( 'NONE',  ( -9.968679514594425584, 5.546356146656833630, 6.001058933476985935 ) ) ;
#91025=CIRCLE ( 'NONE', #21695, 0.5000000000000004441 ) ;
#91030=CARTESIAN_POINT ( 'NONE',  ( 11.86239285000045740, 13.88000000000000078, -1.812080536912752837 ) ) ;
#91044=DIRECTION ( 'NONE',  ( 0.000000000000000000, 0.000000000000000000, 1.000000000000000000 ) ) ;
#91055=CARTESIAN_POINT ( 'NONE',  ( 11.94105721237523277, 13.40000000000000036, 1.187919463087245386 ) ) ;
#91065=CARTESIAN_POINT ( 'NONE',  ( -5.941061940081919346, 14.53065791113160365, 10.43603815422727443 ) ) ;
#91070=CARTESIAN_POINT ( 'NONE',  ( -11.78331023100045449, 11.29999999999998117, 1.799999999999999600 ) ) ;
#91077=SURFACE_SIDE_STYLE ('',( #143046 ) ) ;
#91093=VERTEX_POINT ( 'NONE', #143356 ) ;
#91131=CARTESIAN_POINT ( 'NONE',  ( 11.52888687719590521, 9.805768748949638791, -3.331331986263459388 ) ) ;
#91133=ORIENTED_EDGE ( 'NONE', *, *, #130231, .F. ) ;
#91134=CARTESIAN_POINT ( 'NONE',  ( -11.89839339040395316, 13.82877468403921561, -1.560885614203537219 ) ) ;
#91153=CARTESIAN_POINT ( 'NONE',  ( -10.56580427165518721, 4.154138811340903459, -5.596901375327959727 ) ) ;
#91161=CARTESIAN_POINT ( 'NONE',  ( 11.86145016429272836, 12.69999999999999929, -1.100000000000000311 ) ) ;
#91176=CARTESIAN_POINT ( 'NONE',  ( -11.41108574530281494, 13.75836855377625589, -3.405883542057589253 ) ) ;
#91194=STYLED_ITEM ( 'NONE', ( #21876 ), #114086 ) ;
#91204=DIRECTION ( 'NONE',  ( 0.000000000000000000, 0.000000000000000000, -1.000000000000000000 ) ) ;
#91252=ORIENTED_EDGE ( 'NONE', *, *, #16807, .F. ) ;
#91263=CARTESIAN_POINT ( 'NONE',  ( 7.471411487236919058, 15.41976068137822153, 9.339997063786253051 ) ) ;
#91267=FILL_AREA_STYLE_COLOUR ( '', #92808 ) ;
#91276=EDGE_LOOP ( 'NONE', ( #177257, #51126, #125280, #117349 ) ) ;
#91282=CARTESIAN_POINT ( 'NONE',  ( 0.7124089920921555796, 14.00000000000000711, -12.66466791154696381 ) ) ;
#91304=ADVANCED_FACE ( 'NONE', ( #139595 ), #184877, .T. ) ;
#91312=CARTESIAN_POINT ( 'NONE',  ( -9.719212163200577237, 3.553054704878167325, 6.967211938571212571 ) ) ;
#91322=ORIENTED_EDGE ( 'NONE', *, *, #210558, .F. ) ;
#91325=DIRECTION ( 'NONE',  ( -1.000000000000000000, 0.000000000000000000, 0.000000000000000000 ) ) ;
#91326=CARTESIAN_POINT ( 'NONE',  ( -10.57232049882948388, 5.599334429189661400, -4.968988939937085014 ) ) ;
#91337=CARTESIAN_POINT ( 'NONE',  ( 0.000000000000000000, 15.51887838114830132, 0.000000000000000000 ) ) ;
#91338=ORIENTED_EDGE ( 'NONE', *, *, #62182, .F. ) ;
#91377=CARTESIAN_POINT ( 'NONE',  ( -11.95359438121989548, 12.49578100291300586, 1.059536798430472437 ) ) ;
#91403=CARTESIAN_POINT ( 'NONE',  ( -11.33772465723237666, 13.50868300734826377, 3.600000000000073364 ) ) ;
#91407=VERTEX_POINT ( 'NONE', #174232 ) ;
#91414=CARTESIAN_POINT ( 'NONE',  ( 8.892465212752345138, 12.91714147110841893, 7.587471063468475663 ) ) ;
#91417=ORIENTED_EDGE ( 'NONE', *, *, #52471, .F. ) ;
#91442=DIRECTION ( 'NONE',  ( 0.000000000000000000, 1.000000000000000000, 0.000000000000000000 ) ) ;
#91470=CARTESIAN_POINT ( 'NONE',  ( -7.247736482492992849, 15.00000000000182077, 10.57961706324680584 ) ) ;
#91493=DIRECTION ( 'NONE',  ( 1.000000000000000000, -0.000000000000000000, -0.000000000000000000 ) ) ;
#91514=DIRECTION ( 'NONE',  ( 0.000000000000000000, -1.000000000000000000, 0.000000000000000000 ) ) ;
#91521=CARTESIAN_POINT ( 'NONE',  ( 7.840529994971273453, 15.85037637632706264, 8.677903555585629647 ) ) ;
#91545=FACE_OUTER_BOUND ( 'NONE', #78737, .T. ) ;
#91555=CARTESIAN_POINT ( 'NONE',  ( -12.26626736352559455, 6.252815285820443769, 3.851661612215340647 ) ) ;
#91572=DIRECTION ( 'NONE',  ( 0.000000000000000000, 0.000000000000000000, 1.000000000000000000 ) ) ;
#91578=ORIENTED_EDGE ( 'NONE', *, *, #195389, .T. ) ;
#91585=CARTESIAN_POINT ( 'NONE',  ( 10.40106502431298452, 10.48805886172130997, 5.993424745873436876 ) ) ;
#91597=CARTESIAN_POINT ( 'NONE',  ( 11.07131503167114772, 13.79999999999999716, 0.8043049353970801452 ) ) ;
#91603=B_SPLINE_CURVE_WITH_KNOTS ( 'NONE', 3,
 ( #200069, #21308, #153480, #136170, #185957, #134061 ),
 .UNSPECIFIED., .F., .F.,
 ( 4, 2, 4 ),
 ( 0.001279092382393099943, 0.001599469101539996744, 0.001919845820686893545 ),
 .UNSPECIFIED. ) ;
#91659=EDGE_CURVE ( 'NONE', #144349, #72818, #990, .T. ) ;
#91676=CARTESIAN_POINT ( 'NONE',  ( -11.68462027884434917, 8.171766027648200037, -4.455682980299036089 ) ) ;
#91710=VECTOR ( 'NONE', #54580, 1000.000000000000000 ) ;
#91748=CARTESIAN_POINT ( 'NONE',  ( -10.71748749772954135, 5.309591131546671505, -6.727448623506740333 ) ) ;
#91763=ORIENTED_EDGE ( 'NONE', *, *, #57540, .T. ) ;
#91784=AXIS2_PLACEMENT_3D ( 'NONE', #144130, #174471, #61764 ) ;
#91785=EDGE_CURVE ( 'NONE', #130487, #115079, #5203, .T. ) ;
#91814=COLOUR_RGB ( '', 0.40784314, 0.44705882, 0.49803922) ;
#91827=CARTESIAN_POINT ( 'NONE',  ( 11.84668729035180590, 10.09481419982586736, 1.399999999999998357 ) ) ;
#91840=VERTEX_POINT ( 'NONE', #115645 ) ;
#91847=CARTESIAN_POINT ( 'NONE',  ( 8.889064146099206809, 12.82244507866851180, 7.992677692963079394 ) ) ;
#91853=CARTESIAN_POINT ( 'NONE',  ( -8.159939477482263115, 15.51961010445367961, 8.809817911661959045 ) ) ;
#91856=EDGE_LOOP ( 'NONE', ( #31967, #9404, #188573, #99127 ) ) ;
#91876=CARTESIAN_POINT ( 'NONE',  ( 11.48243876534946217, 9.799999999999982947, 3.199999999999997957 ) ) ;
#91879=CIRCLE ( 'NONE', #46887, 11.09999999999999964 ) ;
#91882=CARTESIAN_POINT ( 'NONE',  ( 11.48243876534946217, 12.30000000000000071, -3.200000000000001510 ) ) ;
#91908=ORIENTED_EDGE ( 'NONE', *, *, #161956, .T. ) ;
#91935=CARTESIAN_POINT ( 'NONE',  ( 11.86239285000045918, 13.79999999999998295, 1.812080536912751283 ) ) ;
#91940=CARTESIAN_POINT ( 'NONE',  ( -10.49071307728992153, 3.038037579769635066, 7.129592439487457689 ) ) ;
#91945=CARTESIAN_POINT ( 'NONE',  ( -11.84103413958613160, 11.11004478473142676, -1.443924719788764799 ) ) ;
#91965=DIRECTION ( 'NONE',  ( 1.509903313490213211E-14, 0.000000000000000000, -1.000000000000000000 ) ) ;
#91975=ORIENTED_EDGE ( 'NONE', *, *, #141380, .T. ) ;
#92001=DIRECTION ( 'NONE',  ( 0.8003905296791061774, 0.000000000000000000, -0.5994789404140897782 ) ) ;
#92005=FILL_AREA_STYLE ('',( #159111 ) ) ;
#92006=AXIS2_PLACEMENT_3D ( 'NONE', #1081, #199287, #202478 ) ;
#92010=CARTESIAN_POINT ( 'NONE',  ( -10.46082884891970366, 3.933599711960402256, 5.880821593625136678 ) ) ;
#92040=CARTESIAN_POINT ( 'NONE',  ( 0.05568659246542585761, 15.51846069310708387, 11.99987079111352983 ) ) ;
#92052=CARTESIAN_POINT ( 'NONE',  ( 1.464677571780234644E-15, 0.000000000000000000, -11.92000000000000171 ) ) ;
#92063=ORIENTED_EDGE ( 'NONE', *, *, #130801, .F. ) ;
#92102=LINE ( 'NONE', #138710, #142181 ) ;
#92104=CARTESIAN_POINT ( 'NONE',  ( -11.48788097203293823, 9.769569456023079468, 3.469500700354829714 ) ) ;
#92137=CARTESIAN_POINT ( 'NONE',  ( -4.705920246013195474, 14.55298554035344694, 10.99996989179731877 ) ) ;
#92162=EDGE_CURVE ( 'NONE', #177822, #161745, #109054, .T. ) ;
#92170=MECHANICAL_DESIGN_GEOMETRIC_PRESENTATION_REPRESENTATION('',(#188910),#36763);
#92174=FACE_OUTER_BOUND ( 'NONE', #187669, .T. ) ;
#92187=ORIENTED_EDGE ( 'NONE', *, *, #131977, .T. ) ;
#92188=( GEOMETRIC_REPRESENTATION_CONTEXT ( 3 ) GLOBAL_UNCERTAINTY_ASSIGNED_CONTEXT ( ( #122528 ) ) GLOBAL_UNIT_ASSIGNED_CONTEXT ( ( #55190, #121337, #21578 ) ) REPRESENTATION_CONTEXT ( 'NONE', 'WORKASPACE' ) );
#92207=ORIENTED_EDGE ( 'NONE', *, *, #33178, .T. ) ;
#92210=CARTESIAN_POINT ( 'NONE',  ( 10.56511880488638333, 13.75886523581518439, -3.405056808716383276 ) ) ;
#92229=CARTESIAN_POINT ( 'NONE',  ( -11.55950211276791428, 9.719999999999982876, 3.221476510067112109 ) ) ;
#92230=CARTESIAN_POINT ( 'NONE',  ( -11.48243876534946217, 9.719999999999982876, 3.199999999999997957 ) ) ;
#92236=CARTESIAN_POINT ( 'NONE',  ( 11.78331023100045627, 9.719999999999998863, -1.800000000000001155 ) ) ;
#92241=EDGE_CURVE ( 'NONE', #118348, #49028, #188443, .T. ) ;
#92276=AXIS2_PLACEMENT_3D ( 'NONE', #26760, #7290, #190318 ) ;
#92277=VECTOR ( 'NONE', #156944, 1000.000000000000000 ) ;
#92315=COLOUR_RGB ( '', 0.40784314, 0.44705882, 0.49803922) ;
#92321=ORIENTED_EDGE ( 'NONE', *, *, #93834, .T. ) ;
#92326=CIRCLE ( 'NONE', #202962, 0.07999999999999998779 ) ;
#92341=( GEOMETRIC_REPRESENTATION_CONTEXT ( 3 ) GLOBAL_UNCERTAINTY_ASSIGNED_CONTEXT ( ( #167980 ) ) GLOBAL_UNIT_ASSIGNED_CONTEXT ( ( #193242, #192157, #10216 ) ) REPRESENTATION_CONTEXT ( 'NONE', 'WORKASPACE' ) );
#92342=CARTESIAN_POINT ( 'NONE',  ( 7.862692832760656891, 15.31533744430288024, 9.008167824251760436 ) ) ;
#92365=EDGE_LOOP ( 'NONE', ( #44520, #171909, #207534, #161527 ) ) ;
#92401=CARTESIAN_POINT ( 'NONE',  ( -11.14501278000869355, 7.223412960316487386, -3.546411330735405265 ) ) ;
#92434=ORIENTED_EDGE ( 'NONE', *, *, #13181, .T. ) ;
#92444=CARTESIAN_POINT ( 'NONE',  ( 11.01135777277262306, 0.000000000000000000, -1.400000000000001910 ) ) ;
#92461=CARTESIAN_POINT ( 'NONE',  ( -11.33772467203841394, 11.00732847981850426, -3.600000000000000977 ) ) ;
#92465=CIRCLE ( 'NONE', #113374, 12.00000000000000178 ) ;
#92473=CARTESIAN_POINT ( 'NONE',  ( 11.15287142971249246, 9.124439414695240558, 4.432553360691933619 ) ) ;
#92491=CARTESIAN_POINT ( 'NONE',  ( 11.22826844164464433, 7.784147190670918093, 5.449213193111969389 ) ) ;
#92493=VERTEX_POINT ( 'NONE', #43411 ) ;
#92505=B_SPLINE_CURVE_WITH_KNOTS ( 'NONE', 3,
 ( #196276, #91597, #114034, #207441, #9246, #157649 ),
 .UNSPECIFIED., .F., .F.,
 ( 4, 2, 4 ),
 ( 0.0006258038130483377197, 0.0009388807108837884767, 0.001251957608719239234 ),
 .UNSPECIFIED. ) ;
#92506=CARTESIAN_POINT ( 'NONE',  ( -6.748402506350539731, 15.51952511195976214, -9.932705294953846575 ) ) ;
#92508=CARTESIAN_POINT ( 'NONE',  ( 9.406792723036451420, 4.446947629225756593, -7.380298948578194462 ) ) ;
#92510=DIRECTION ( 'NONE',  ( 1.000000000000000000, -0.000000000000000000, 1.224646799147353207E-16 ) ) ;
#92518=DIRECTION ( 'NONE',  ( 0.000000000000000000, 0.000000000000000000, 1.000000000000000000 ) ) ;
#92520=CARTESIAN_POINT ( 'NONE',  ( -15.75000000000000000, 12.30000000000000071, -1.800000000000001155 ) ) ;
#92549=CARTESIAN_POINT ( 'NONE',  ( -3.796053574492201044, 16.00000000000182254, 12.24940615670304211 ) ) ;
#92554=DIRECTION ( 'NONE',  ( 0.000000000000000000, 0.000000000000000000, -1.000000000000000000 ) ) ;
#92569=SURFACE_SIDE_STYLE ('',( #108854 ) ) ;
#92577=DIRECTION ( 'NONE',  ( 0.000000000000000000, -0.000000000000000000, 1.000000000000000000 ) ) ;
#92589=CARTESIAN_POINT ( 'NONE',  ( -10.47657863273387058, 4.460721775326359939, 5.863621068794715896 ) ) ;
#92595=CARTESIAN_POINT ( 'NONE',  ( 10.03397232106342862, 14.16760128048179723, 7.472996930959428852 ) ) ;
#92612=DIRECTION ( 'NONE',  ( 0.000000000000000000, 0.000000000000000000, -1.000000000000000000 ) ) ;
#92627=CARTESIAN_POINT ( 'NONE',  ( -12.36958382383909871, 9.653479897959526213, -1.396270995789667513 ) ) ;
#92628=CIRCLE ( 'NONE', #64903, 11.92000000000000171 ) ;
#92651=ORIENTED_EDGE ( 'NONE', *, *, #39389, .F. ) ;
#92652=CARTESIAN_POINT ( 'NONE',  ( 11.52487297331679095, 8.447199575603240973, 3.365429268895913761 ) ) ;
#92662=CARTESIAN_POINT ( 'NONE',  ( -11.89197369110779867, 13.80000000000000249, 0.8056055387119849254 ) ) ;
#92679=CARTESIAN_POINT ( 'NONE',  ( 11.07790593930098311, 9.799999999999998934, 0.6999999999999992895 ) ) ;
#92686=ADVANCED_FACE ( 'NONE', ( #92174 ), #75763, .T. ) ;
#92694=SURFACE_STYLE_USAGE ( .BOTH. , #141469 ) ;
#92697=CARTESIAN_POINT ( 'NONE',  ( -11.01453822196416077, 5.351648037286913073, 4.768917646641087416 ) ) ;
#92736=CARTESIAN_POINT ( 'NONE',  ( -10.45142907045522129, 5.144535043903895932, -5.216774619840575333 ) ) ;
#92742=ADVANCED_FACE ( 'NONE', ( #213328 ), #9346, .T. ) ;
#92759=CIRCLE ( 'NONE', #213763, 11.95586206894156689 ) ;
#92801=CARTESIAN_POINT ( 'NONE',  ( -15.75000000000000000, 13.39999999999998259, 3.599999999999999201 ) ) ;
#92803=( GEOMETRIC_REPRESENTATION_CONTEXT ( 3 ) GLOBAL_UNCERTAINTY_ASSIGNED_CONTEXT ( ( #99231 ) ) GLOBAL_UNIT_ASSIGNED_CONTEXT ( ( #194148, #40723, #145458 ) ) REPRESENTATION_CONTEXT ( 'NONE', 'WORKASPACE' ) );
#92805=CARTESIAN_POINT ( 'NONE',  ( -11.41381675112453387, 13.40000000000000036, -3.704697986577184299 ) ) ;
#92808=COLOUR_RGB ( '', 0.31764706, 0.68627451, 0.89019608) ;
#92811=CARTESIAN_POINT ( 'NONE',  ( -10.19200560444942560, 4.477620260464512114, -5.707107691925500603 ) ) ;
#92831=CARTESIAN_POINT ( 'NONE',  ( -15.75000000000000000, 10.19999999999999929, -3.600000000000000977 ) ) ;
#92889=EDGE_LOOP ( 'NONE', ( #127570, #17141 ) ) ;
#92902=LINE ( 'NONE', #206614, #68439 ) ;
#92909=CARTESIAN_POINT ( 'NONE',  ( 11.95103256899996502, 6.645237973884175808, 0.4970601757468578463 ) ) ;
#92912=CARTESIAN_POINT ( 'NONE',  ( -10.28373532799257539, 4.806408141292263458, 6.104877701959067871 ) ) ;
#92916=CARTESIAN_POINT ( 'NONE',  ( -7.829692872007384175, 15.51984681892806073, 9.104471052007852450 ) ) ;
#92949=CARTESIAN_POINT ( 'NONE',  ( 9.397879144821100539, 13.53129603721547980, -7.462055881301290050 ) ) ;
#92999=ORIENTED_EDGE ( 'NONE', *, *, #20907, .T. ) ;
#93002=CARTESIAN_POINT ( 'NONE',  ( 11.73212044392280262, 8.686627382477217552, -4.360314433000339385 ) ) ;
#93003=CARTESIAN_POINT ( 'NONE',  ( -11.73082749631449140, 4.534045925630191931, 5.066687987500840151 ) ) ;
#93007=AXIS2_PLACEMENT_3D ( 'NONE', #129632, #26703, #11519 ) ;
#93072=CARTESIAN_POINT ( 'NONE',  ( -10.65376315971086640, 4.226338639847933898, 5.523257262081396668 ) ) ;
#93101=DIRECTION ( 'NONE',  ( 0.000000000000000000, 0.000000000000000000, -1.000000000000000000 ) ) ;
#93110=CARTESIAN_POINT ( 'NONE',  ( 0.000000000000000000, 15.44694763437329676, -11.95586206896577153 ) ) ;
#93114=CARTESIAN_POINT ( 'NONE',  ( -0.08053691275167716712, 15.51846456562902965, 11.99972973886013961 ) ) ;
#93121=EDGE_CURVE ( 'NONE', #79124, #79300, #185034, .T. ) ;
#93151=VERTEX_POINT ( 'NONE', #33821 ) ;
#93171=B_SPLINE_CURVE_WITH_KNOTS ( 'NONE', 3,
 ( #182870, #18224, #53952, #101629, #186065, #103777, #201236, #150393, #51826, #68025, #52877, #119013, #123315, #126501, #40918, #174131, #107024, #205517, #176247, #60341, #189279, #41995, #157870, #105948, #27849, #25704, #93947, #173049, #158922, #76593, #44118, #140575, #57149, #206588 ),
 .UNSPECIFIED., .F., .F.,
 ( 4, 2, 2, 2, 2, 2, 2, 2, 2, 2, 2, 2, 2, 2, 2, 2, 4 ),
 ( 1.734723475976807094E-18, 0.001499835624873080290, 0.002999671249746158844, 0.004499506874619237616, 0.005999342499492315954, 0.007499178124365395159, 0.008999013749238471763, 0.009748931561675010932, 0.01049884937411154663, 0.01199868499898462497, 0.01349852062385770504, 0.01499835624873078165, 0.01649819187360385825, 0.01799802749847694006, 0.02099769874822308285, 0.02249753437309615772, 0.02399736999796922565 ),
 .UNSPECIFIED. ) ;
#93174=ADVANCED_FACE ( 'NONE', ( #118342 ), #212718, .F. ) ;
#93181=ORIENTED_EDGE ( 'NONE', *, *, #151057, .T. ) ;
#93214=CARTESIAN_POINT ( 'NONE',  ( -1.423205080756925867, 7.980384757729337863, -10.65537363484301636 ) ) ;
#93235=AXIS2_PLACEMENT_3D ( 'NONE', #174503, #110613, #43429 ) ;
#93248=LINE ( 'NONE', #143081, #23811 ) ;
#93252=CARTESIAN_POINT ( 'NONE',  ( 0.000000000000000000, 0.000000000000000000, 0.000000000000000000 ) ) ;
#93262=ADVANCED_FACE ( 'NONE', ( #136677 ), #185397, .F. ) ;
#93266=ORIENTED_EDGE ( 'NONE', *, *, #84325, .T. ) ;
#93269=DIRECTION ( 'NONE',  ( 0.000000000000000000, 0.000000000000000000, -1.000000000000000000 ) ) ;
#93288=CARTESIAN_POINT ( 'NONE',  ( -11.96217875511318240, 13.82854366578976979, 0.9561995067075053090 ) ) ;
#93289=CARTESIAN_POINT ( 'NONE',  ( -10.72841194583914515, 4.501991598509155423, -5.277862265383093998 ) ) ;
#93291=CARTESIAN_POINT ( 'NONE',  ( -11.43195036480940452, 9.944755037147515964, 3.649565797774462883 ) ) ;
#93354=CARTESIAN_POINT ( 'NONE',  ( -9.748756651352278979, 4.000007913748506283, -7.301653494139321410 ) ) ;
#93364=CARTESIAN_POINT ( 'NONE',  ( 11.92051736251532823, 11.15180243792678638, -1.381800029228912763 ) ) ;
#93375=ORIENTED_EDGE ( 'NONE', *, *, #193499, .F. ) ;
#93389=ORIENTED_EDGE ( 'NONE', *, *, #167734, .T. ) ;
#93398=ADVANCED_FACE ( 'NONE', ( #149717 ), #23221, .T. ) ;
#93399=CARTESIAN_POINT ( 'NONE',  ( 7.904908961251512878, 15.38485759653958240, 9.030111759985443243 ) ) ;
#93400=DIRECTION ( 'NONE',  ( -0.000000000000000000, -1.000000000000000000, -0.000000000000000000 ) ) ;
#93403=CARTESIAN_POINT ( 'NONE',  ( -11.89942855770814134, 12.30000000000000071, -0.7000000000000009548 ) ) ;
#93406=CARTESIAN_POINT ( 'NONE',  ( 11.96217875511317885, 12.27145633421023518, 0.9561995067075056420 ) ) ;
#93416=VERTEX_POINT ( 'NONE', #75926 ) ;
#93436=VECTOR ( 'NONE', #114152, 1000.000000000000000 ) ;
#93441=VERTEX_POINT ( 'NONE', #158262 ) ;
#93455=CARTESIAN_POINT ( 'NONE',  ( 11.52888687719656957, 11.29423125104975512, 3.331331986263658784 ) ) ;
#93460=EDGE_LOOP ( 'NONE', ( #4636, #90679, #140184, #200702 ) ) ;
#93464=CARTESIAN_POINT ( 'NONE',  ( 11.84668730067608600, 13.39999999999998259, 1.319999999999998286 ) ) ;
#93465=CARTESIAN_POINT ( 'NONE',  ( -6.755832238374201992, 14.48046842839597836, -9.927744211455593160 ) ) ;
#93474=MECHANICAL_DESIGN_GEOMETRIC_PRESENTATION_REPRESENTATION('',(#114243),#72718);
#93489=CARTESIAN_POINT ( 'NONE',  ( -11.41381675112453387, 13.40000000000000036, -3.704697986577184299 ) ) ;
#93527=( NAMED_UNIT ( * ) PLANE_ANGLE_UNIT ( ) SI_UNIT ( $, .RADIAN. ) );
#93530=LINE ( 'NONE', #111966, #72969 ) ;
#93537=( NAMED_UNIT ( * ) SI_UNIT ( $, .STERADIAN. ) SOLID_ANGLE_UNIT ( ) );
#93546=CARTESIAN_POINT ( 'NONE',  ( 8.831606621645018862, 13.23576961196815205, 7.655963609598713582 ) ) ;
#93552=ORIENTED_EDGE ( 'NONE', *, *, #70698, .F. ) ;
#93554=VERTEX_POINT ( 'NONE', #88996 ) ;
#93564=CARTESIAN_POINT ( 'NONE',  ( 9.601932014265541326, 4.115787152683093808, -7.121345992675182757 ) ) ;
#93578=AXIS2_PLACEMENT_3D ( 'NONE', #114393, #39461, #54644 ) ;
#93582=CARTESIAN_POINT ( 'NONE',  ( -11.88234649872613602, 11.25660782916751579, -0.9090484974825174813 ) ) ;
#93584=EDGE_CURVE ( 'NONE', #109578, #22427, #154139, .T. ) ;
#93606=CARTESIAN_POINT ( 'NONE',  ( -11.33171338088452451, 6.586873243287150181, 3.814917260415342959 ) ) ;
#93635=DIRECTION ( 'NONE',  ( 0.000000000000000000, 0.000000000000000000, 1.000000000000000000 ) ) ;
#93636=CARTESIAN_POINT ( 'NONE',  ( -15.75000000000000000, 12.30000000000000071, -1.800000000000001155 ) ) ;
#93637=FILL_AREA_STYLE ('',( #205203 ) ) ;
#93647=CARTESIAN_POINT ( 'NONE',  ( -9.858348327010764578, 3.999999999999995559, 6.855072103023518437 ) ) ;
#93651=CARTESIAN_POINT ( 'NONE',  ( 7.826754997383993384, 14.96923099944252478, -9.976823565866945742 ) ) ;
#93654=CARTESIAN_POINT ( 'NONE',  ( 9.023309422432060245, 13.48888919738144665, 9.153259163867227599 ) ) ;
#93689=CARTESIAN_POINT ( 'NONE',  ( -11.87992086682929660, 5.100687730227392969, -4.764507118098673111 ) ) ;
#93697=EDGE_CURVE ( 'NONE', #50054, #7711, #107210, .T. ) ;
#93715=CARTESIAN_POINT ( 'NONE',  ( 12.00021129026602651, 7.586573191464381694, -0.2104672827513448807 ) ) ;
#93719=B_SPLINE_CURVE_WITH_KNOTS ( 'NONE', 3,
 ( #78051, #127977, #29310, #209096, #59669, #60731 ),
 .UNSPECIFIED., .F., .F.,
 ( 4, 2, 4 ),
 ( 0.000000000000000000, 0.0003141588434155108628, 0.0006283176868310217256 ),
 .UNSPECIFIED. ) ;
#93734=( GEOMETRIC_REPRESENTATION_CONTEXT ( 3 ) GLOBAL_UNCERTAINTY_ASSIGNED_CONTEXT ( ( #185024 ) ) GLOBAL_UNIT_ASSIGNED_CONTEXT ( ( #81896, #116584, #198819 ) ) REPRESENTATION_CONTEXT ( 'NONE', 'WORKASPACE' ) );
#93783=CIRCLE ( 'NONE', #145600, 11.09999999999999964 ) ;
#93805=CARTESIAN_POINT ( 'NONE',  ( -10.02511099414689077, 5.770000865873268658, 5.887978427067937837 ) ) ;
#93809=FILL_AREA_STYLE_COLOUR ( '', #121852 ) ;
#93834=EDGE_CURVE ( 'NONE', #66250, #94599, #78754, .T. ) ;
#93836=CARTESIAN_POINT ( 'NONE',  ( -8.121044095224613457, 15.44793984265997189, 8.785326000989064354 ) ) ;
#93857=ORIENTED_EDGE ( 'NONE', *, *, #162091, .F. ) ;
#93881=CARTESIAN_POINT ( 'NONE',  ( -10.68988767858338917, 3.994679225574373493, -4.900161361628223133 ) ) ;
#93886=ORIENTED_EDGE ( 'NONE', *, *, #54909, .F. ) ;
#93908=EDGE_CURVE ( 'NONE', #112981, #26907, #12187, .T. ) ;
#93941=CIRCLE ( 'NONE', #28195, 11.67999951260719804 ) ;
#93945=DIRECTION ( 'NONE',  ( 0.000000000000000000, 0.000000000000000000, -1.000000000000000000 ) ) ;
#93947=CARTESIAN_POINT ( 'NONE',  ( 10.91746247397144209, 8.226910605520304287, 4.997041797683915654 ) ) ;
#93959=CARTESIAN_POINT ( 'NONE',  ( 11.87828357750012565, 9.796897472595873069, 1.708055325888905962 ) ) ;
#93978=CARTESIAN_POINT ( 'NONE',  ( 8.812339285468201666, 13.17645074827856710, 8.077252134077332002 ) ) ;
#93981=FACE_OUTER_BOUND ( 'NONE', #31572, .T. ) ;
#93985=CARTESIAN_POINT ( 'NONE',  ( -9.367496997602099640, 14.48154074412328995, -7.499999999994433786 ) ) ;
#93997=CARTESIAN_POINT ( 'NONE',  ( 2.195822763121351960E-15, 15.42895922032036715, 11.92238959702059731 ) ) ;
#93998=COLOUR_RGB ( '', 0.31764706, 0.68627451, 0.89019608) ;
#94007=CARTESIAN_POINT ( 'NONE',  ( 11.45842088241066392, 10.00693529122952086, 3.566211699757795284 ) ) ;
#94018=CARTESIAN_POINT ( 'NONE',  ( 8.715232613915466331, 14.87911529561621649, -8.250190486245246646 ) ) ;
#94060=CARTESIAN_POINT ( 'NONE',  ( 8.776224899084628106, 13.27471476138783224, 8.184001253707569035 ) ) ;
#94068=DIRECTION ( 'NONE',  ( -0.000000000000000000, -1.000000000000000000, -0.000000000000000000 ) ) ;
#94069=CARTESIAN_POINT ( 'NONE',  ( 11.72719273365024506, 8.694648967210921953, 4.374500150831954315 ) ) ;
#94121=EDGE_LOOP ( 'NONE', ( #205909, #167533, #192075, #86257 ) ) ;
#94122=STYLED_ITEM ( 'NONE', ( #107970 ), #27695 ) ;
#94129=CARTESIAN_POINT ( 'NONE',  ( -11.04536101718726293, 13.40000000000000036, 1.099999999999996758 ) ) ;
#94134=CARTESIAN_POINT ( 'NONE',  ( 9.406473631745788211, 4.446947634372973468, 7.380697509896862130 ) ) ;
#94218=CARTESIAN_POINT ( 'NONE',  ( -10.39320420135713263, 4.932286138528427344, 5.331284845095887626 ) ) ;
#94222=ADVANCED_FACE ( 'NONE', ( #201369 ), #39713, .T. ) ;
#94223=UNCERTAINTY_MEASURE_WITH_UNIT (LENGTH_MEASURE( 1.000000000000000082E-05 ), #192647, 'distance_accuracy_value', 'NONE');
#94245=ORIENTED_EDGE ( 'NONE', *, *, #153873, .F. ) ;
#94282=AXIS2_PLACEMENT_3D ( 'NONE', #27452, #14120, #197155 ) ;
#94304=CYLINDRICAL_SURFACE ( 'NONE', #37236, 12.00000000000000178 ) ;
#94318=FILL_AREA_STYLE ('',( #28225 ) ) ;
#94330=ORIENTED_EDGE ( 'NONE', *, *, #76833, .T. ) ;
#94336=CARTESIAN_POINT ( 'NONE',  ( -9.345711740228745512, 14.55696679586869458, 7.452166123624950345 ) ) ;
#94338=ORIENTED_EDGE ( 'NONE', *, *, #94666, .T. ) ;
#94349=EDGE_CURVE ( 'NONE', #7772, #79400, #61039, .T. ) ;
#94370=( BOUNDED_SURFACE ( )  B_SPLINE_SURFACE ( 3, 3, ( 
 ( #4811, #24284, #90390, #25370, #70893, #91470, #9126, #75202 ),
 ( #141313, #44860, #193213, #128316, #63213, #12313, #146629, #13389 ),
 ( #176972, #127243, #58946, #110964, #143442, #60012, #142371, #158588 ),
 ( #28589, #79465, #129377, #94677, #125103, #191061, #112044, #10188 ),
 ( #126165, #42726, #159654, #194279, #80533, #108834, #160719, #29661 ),
 ( #174860, #179110, #26439, #62158, #92549, #192129, #45924, #145582 ),
 ( #78394, #209439, #144514, #210522, #178045, #30732, #109907, #96815 ) ),
 .UNSPECIFIED., .T., .F., .F. ) 
 B_SPLINE_SURFACE_WITH_KNOTS ( ( 4, 3, 4 ),
 ( 4, 2, 2, 4 ),
 ( 0.000000000000000000, 0.5000000000000000000, 1.000000000000000000 ),
 ( 0.000000000000000000, 0.08643212109064293824, 0.5432160605453214552, 1.000000000000000000 ),
 .UNSPECIFIED. ) 
 GEOMETRIC_REPRESENTATION_ITEM ( )  RATIONAL_B_SPLINE_SURFACE ( (
 ( 1.000000000000000000, 1.000000000000000000, 1.000000000000000000, 1.000000000000000000, 1.000000000000000000, 1.000000000000000000, 1.000000000000000000, 1.000000000000000000),
 ( 0.3333333333333333703, 0.3333333333333333703, 0.3333333333333333703, 0.3333333333333333703, 0.3333333333333333703, 0.3333333333333333703, 0.3333333333333333703, 0.3333333333333333703),
 ( 0.3333333333333333703, 0.3333333333333333703, 0.3333333333333333703, 0.3333333333333333703, 0.3333333333333333703, 0.3333333333333333703, 0.3333333333333333703, 0.3333333333333333703),
 ( 1.000000000000000000, 1.000000000000000000, 1.000000000000000000, 1.000000000000000000, 1.000000000000000000, 1.000000000000000000, 1.000000000000000000, 1.000000000000000000),
 ( 0.3333333333333333703, 0.3333333333333333703, 0.3333333333333333703, 0.3333333333333333703, 0.3333333333333333703, 0.3333333333333333703, 0.3333333333333333703, 0.3333333333333333703),
 ( 0.3333333333333333703, 0.3333333333333333703, 0.3333333333333333703, 0.3333333333333333703, 0.3333333333333333703, 0.3333333333333333703, 0.3333333333333333703, 0.3333333333333333703),
 ( 1.000000000000000000, 1.000000000000000000, 1.000000000000000000, 1.000000000000000000, 1.000000000000000000, 1.000000000000000000, 1.000000000000000000, 1.000000000000000000) ) ) 
 REPRESENTATION_ITEM ( '' )  SURFACE ( )  );
#94402=PLANE ( 'NONE',  #82325 ) ;
#94410=CARTESIAN_POINT ( 'NONE',  ( -11.48806469435255373, 13.83089772872446943, 3.468902948106700634 ) ) ;
#94431=CARTESIAN_POINT ( 'NONE',  ( 11.92619525870751573, 11.02622296793679979, -1.328859154004804699 ) ) ;
#94434=CARTESIAN_POINT ( 'NONE',  ( -11.52888687719587146, 12.30576874894960682, 3.331331986263616152 ) ) ;
#94446=CARTESIAN_POINT ( 'NONE',  ( -15.75000000000000000, 10.19999999999999929, -0.7000000000000009548 ) ) ;
#94453=VECTOR ( 'NONE', #108821, 1000.000000000000000 ) ;
#94468=( GEOMETRIC_REPRESENTATION_CONTEXT ( 3 ) GLOBAL_UNCERTAINTY_ASSIGNED_CONTEXT ( ( #109455 ) ) GLOBAL_UNIT_ASSIGNED_CONTEXT ( ( #90516, #122019, #203157 ) ) REPRESENTATION_CONTEXT ( 'NONE', 'WORKASPACE' ) );
#94482=VECTOR ( 'NONE', #190863, 1000.000000000000000 ) ;
#94483=CARTESIAN_POINT ( 'NONE',  ( -7.247736482492767252, 15.00000000000521538, -10.57961706324489626 ) ) ;
#94597=CARTESIAN_POINT ( 'NONE',  ( -11.07790593930098311, 11.29999999999999893, -0.7000000000000009548 ) ) ;
#94599=VERTEX_POINT ( 'NONE', #194236 ) ;
#94600=EDGE_CURVE ( 'NONE', #167139, #84713, #30691, .T. ) ;
#94620=CARTESIAN_POINT ( 'NONE',  ( 11.19153690645859456, 7.659836902099854683, -3.616912593835723388 ) ) ;
#94657=EDGE_CURVE ( 'NONE', #162756, #123444, #78059, .T. ) ;
#94666=EDGE_CURVE ( 'NONE', #108640, #8935, #188610, .T. ) ;
#94674=CARTESIAN_POINT ( 'NONE',  ( -11.77709913112472684, 7.702278142422434470, -2.066753809368463646 ) ) ;
#94677=CARTESIAN_POINT ( 'NONE',  ( -1.724555757182492988, 14.99999999999692157, 11.68000002332616383 ) ) ;
#94684=STYLED_ITEM ( 'NONE', ( #100968 ), #69155 ) ;
#94694=VERTEX_POINT ( 'NONE', #49022 ) ;
#94716=CARTESIAN_POINT ( 'NONE',  ( 1.469576158976824342E-15, 3.999999999999998224, -12.00000000000000355 ) ) ;
#94720=CARTESIAN_POINT ( 'NONE',  ( 6.871661793415180242, 16.00000000000000000, -9.446021445709373410 ) ) ;
#94723=CARTESIAN_POINT ( 'NONE',  ( 8.310125652063469204, 13.22383526519563368, 8.544412637909269748 ) ) ;
#94729=ORIENTED_EDGE ( 'NONE', *, *, #61508, .F. ) ;
#94744=CARTESIAN_POINT ( 'NONE',  ( -9.949568243101348131, 5.483630524090502334, 6.039417671888569039 ) ) ;
#94755=CARTESIAN_POINT ( 'NONE',  ( -11.01578653029999266, 5.045029590669321884, -4.264301349201883085 ) ) ;
#94772=CARTESIAN_POINT ( 'NONE',  ( -9.351007409505983858, 14.56055123930838668, 7.441777623061154756 ) ) ;
#94779=CARTESIAN_POINT ( 'NONE',  ( 11.95152720720105322, 7.668029601719960731, -1.099342792201368324 ) ) ;
#94827=CARTESIAN_POINT ( 'NONE',  ( -11.68195787049182854, 7.294744277220263307, 2.753462545645998016 ) ) ;
#94832=DIRECTION ( 'NONE',  ( 1.000000000000000000, -0.000000000000000000, -0.000000000000000000 ) ) ;
#94836=CARTESIAN_POINT ( 'NONE',  ( -11.94017496638997500, 8.960613251662856271, 1.236227153985048677 ) ) ;
#94858=CARTESIAN_POINT ( 'NONE',  ( 0.000000000000000000, 18.91999999999999815, 0.000000000000000000 ) ) ;
#94866=CARTESIAN_POINT ( 'NONE',  ( -11.58085191697663241, 6.132731128919016506, 5.153920277027906671 ) ) ;
#94874=B_SPLINE_CURVE_WITH_KNOTS ( 'NONE', 3,
 ( #204597, #137511, #55182, #139656, #159075, #191554, #175345, #121328, #124533, #172135, #90897, #56249, #23730, #155884, #171052, #58377 ),
 .UNSPECIFIED., .F., .F.,
 ( 4, 2, 2, 2, 2, 2, 2, 4 ),
 ( 8.701399832109953910E-22, 0.001350634887644582482, 0.002701269775289164964, 0.004051904662933747230, 0.005402539550578328194, 0.006753174438222909158, 0.008103809325867490990, 0.01080507910115665465 ),
 .UNSPECIFIED. ) ;
#94886=CARTESIAN_POINT ( 'NONE',  ( -11.84103413958623818, 12.48995521526850361, 1.443924719788817423 ) ) ;
#94910=CARTESIAN_POINT ( 'NONE',  ( 9.453622214572602545, 4.518459228531209959, 7.392429638475896070 ) ) ;
#94920=ORIENTED_EDGE ( 'NONE', *, *, #185104, .F. ) ;
#94941=CARTESIAN_POINT ( 'NONE',  ( -11.55090974143167060, 4.033601484819619110, -5.407241547083907918 ) ) ;
#94989=CARTESIAN_POINT ( 'NONE',  ( 0.000000000000000000, 9.719999999999998863, 0.000000000000000000 ) ) ;
#95020=CARTESIAN_POINT ( 'NONE',  ( -11.86239285000045918, 12.21999999999998288, 1.812080536912751061 ) ) ;
#95037=CARTESIAN_POINT ( 'NONE',  ( 9.969705528599281052, 9.873875388196676539, 6.618200077599721176 ) ) ;
#95041=CYLINDRICAL_SURFACE ( 'NONE', #111199, 0.3999999999999997446 ) ;
#95045=FACE_OUTER_BOUND ( 'NONE', #42591, .T. ) ;
#95069=CARTESIAN_POINT ( 'NONE',  ( -11.84668730067608600, 10.89999999999998259, 1.399999999999998579 ) ) ;
#95080=CARTESIAN_POINT ( 'NONE',  ( 9.105083262974959624, 14.28913828790224194, -7.747438832664901298 ) ) ;
#95096=AXIS2_PLACEMENT_3D ( 'NONE', #201079, #184836, #205363 ) ;
#95105=DIRECTION ( 'NONE',  ( 0.000000000000000000, 0.000000000000000000, 1.000000000000000000 ) ) ;
#95116=CARTESIAN_POINT ( 'NONE',  ( -11.48243876534946217, 12.29999999999998295, 3.199999999999997957 ) ) ;
#95131=CARTESIAN_POINT ( 'NONE',  ( 11.09909601403977852, 9.551700265434966752, 4.072285437489899351 ) ) ;
#95137=FACE_OUTER_BOUND ( 'NONE', #20784, .T. ) ;
#95192=CARTESIAN_POINT ( 'NONE',  ( 9.527745260137857386, 12.67567440174593152, -7.221966599662466457 ) ) ;
#95204=AXIS2_PLACEMENT_3D ( 'NONE', #55484, #205987, #24032 ) ;
#95216=CARTESIAN_POINT ( 'NONE',  ( 0.000000000000000000, 0.000000000000000000, 0.000000000000000000 ) ) ;
#95230=EDGE_CURVE ( 'NONE', #102449, #138623, #98936, .T. ) ;
#95247=CARTESIAN_POINT ( 'NONE',  ( -11.92619526913699879, 10.90000000000000036, -1.328859060402686199 ) ) ;
#95275=CARTESIAN_POINT ( 'NONE',  ( -9.453429866517900848, 14.52868746961063096, 7.391430727348221374 ) ) ;
#95283=CARTESIAN_POINT ( 'NONE',  ( 11.96215121607992771, 12.27166446219175988, -0.9565349792967603459 ) ) ;
#95287=CARTESIAN_POINT ( 'NONE',  ( -9.811677024507259759, 4.107325997343203028, 6.339424533126782002 ) ) ;
#95314=ADVANCED_FACE ( 'NONE', ( #57344 ), #81605, .T. ) ;
#95318=CIRCLE ( 'NONE', #5258, 0.08000000000000040412 ) ;
#95339=CARTESIAN_POINT ( 'NONE',  ( -1.667727920668650388, 14.55184893431462356, 11.87324708719159183 ) ) ;
#95365=VERTEX_POINT ( 'NONE', #31250 ) ;
#95371=CARTESIAN_POINT ( 'NONE',  ( 11.91826848676304529, 11.00833707238745696, 1.400000051402190193 ) ) ;
#95389=FACE_OUTER_BOUND ( 'NONE', #30934, .T. ) ;
#95391=CARTESIAN_POINT ( 'NONE',  ( -11.07790593930098311, 11.29999999999999893, -0.7000000000000009548 ) ) ;
#95404=SURFACE_SIDE_STYLE ('',( #177699 ) ) ;
#95408=ORIENTED_EDGE ( 'NONE', *, *, #23468, .F. ) ;
#95415=ORIENTED_EDGE ( 'NONE', *, *, #125962, .T. ) ;
#95465=( BOUNDED_SURFACE ( )  B_SPLINE_SURFACE ( 3, 2, ( 
 ( #26596, #58036, #61239 ),
 ( #110058, #123149, #92697 ),
 ( #76411, #142521, #126321 ),
 ( #192282, #176070, #193368 ),
 ( #177126, #146788, #145737 ),
 ( #46076, #163018, #13546 ),
 ( #213852, #178202, #62308 ),
 ( #95903, #63375, #94827 ),
 ( #211737, #16726, #79618 ),
 ( #161955, #129531, #195511 ),
 ( #47148, #128467, #98031 ),
 ( #64441, #112196, #197621 ),
 ( #113264, #194435, #29819 ),
 ( #181381, #212803, #14600 ),
 ( #160879, #180325, #148887 ),
 ( #196575, #114329, #48217 ),
 ( #78548, #31947, #165135 ),
 ( #80697, #164085, #179269 ),
 ( #30892, #96970, #130585 ),
 ( #99083, #15666, #81753 ),
 ( #49266, #147835, #28743 ),
 ( #65473, #131623, #115387 ),
 ( #66528, #33004, #82810 ),
 ( #144666, #460, #132671 ),
 ( #198677, #111123, #12473 ),
 ( #210679, #183507, #22043 ),
 ( #103335, #53514, #185631 ),
 ( #199749, #87080, #166194 ) ),
 .UNSPECIFIED., .F., .F., .T. ) 
 B_SPLINE_SURFACE_WITH_KNOTS ( ( 4, 2, 2, 2, 2, 2, 2, 2, 2, 2, 2, 2, 2, 4 ),
 ( 3, 3 ),
 ( 1.301042606982605321E-18, 0.001582303952082990970, 0.002373455928124485696, 0.003164607904165980638, 0.003955759880207476015, 0.004746911856248970524, 0.006329215808331960409, 0.007120367784373455786, 0.007911519760414950295, 0.008702671736456444804, 0.009493823712497939313, 0.01028497568853943556, 0.01107612766458093007, 0.01265843161666391908 ),
 ( 0.000000000000000000, 1.000000000000000000 ),
 .UNSPECIFIED. ) 
 GEOMETRIC_REPRESENTATION_ITEM ( )  RATIONAL_B_SPLINE_SURFACE ( (
 ( 1.000000000000000000, 0.8462409035377600475, 1.000000000000000000),
 ( 1.000000000000000000, 0.8465427114078758475, 1.000000000000000000),
 ( 1.000000000000000000, 0.8465641366848090099, 1.000000000000000000),
 ( 1.000000000000000000, 0.8467900531823037147, 1.000000000000000000),
 ( 1.000000000000000000, 0.8468781625786160339, 1.000000000000000000),
 ( 1.000000000000000000, 0.8471120945301685579, 1.000000000000000000),
 ( 1.000000000000000000, 0.8472463485371222180, 1.000000000000000000),
 ( 1.000000000000000000, 0.8473012231814394113, 1.000000000000000000),
 ( 1.000000000000000000, 0.8468507819384271107, 1.000000000000000000),
 ( 1.000000000000000000, 0.8460871546575347013, 1.000000000000000000),
 ( 1.000000000000000000, 0.8457728595780946712, 1.000000000000000000),
 ( 1.000000000000000000, 0.8456955564162187411, 1.000000000000000000),
 ( 1.000000000000000000, 0.8472150014537547236, 1.000000000000000000),
 ( 1.000000000000000000, 0.8472169592757342604, 1.000000000000000000),
 ( 1.000000000000000000, 0.8467840124556752501, 1.000000000000000000),
 ( 1.000000000000000000, 0.8461344581662409992, 1.000000000000000000),
 ( 1.000000000000000000, 0.8459097183282422439, 1.000000000000000000),
 ( 1.000000000000000000, 0.8459637398922701390, 1.000000000000000000),
 ( 1.000000000000000000, 0.8462437954697883402, 1.000000000000000000),
 ( 1.000000000000000000, 0.8469148800072623384, 1.000000000000000000),
 ( 1.000000000000000000, 0.8472862011760097234, 1.000000000000000000),
 ( 1.000000000000000000, 0.8472609020320528428, 1.000000000000000000),
 ( 1.000000000000000000, 0.8471586627785127055, 1.000000000000000000),
 ( 1.000000000000000000, 0.8469901278039179138, 1.000000000000000000),
 ( 1.000000000000000000, 0.8469207196612665856, 1.000000000000000000),
 ( 1.000000000000000000, 0.8466859688974881504, 1.000000000000000000),
 ( 1.000000000000000000, 0.8465495423952427156, 1.000000000000000000),
 ( 1.000000000000000000, 0.8462407054814423679, 1.000000000000000000) ) ) 
 REPRESENTATION_ITEM ( '' )  SURFACE ( )  );
#95477=CARTESIAN_POINT ( 'NONE',  ( 8.133143982689912121, 14.25145509247576570, 8.763746397669734733 ) ) ;
#95482=EDGE_LOOP ( 'NONE', ( #160901, #43735, #34267, #190104, #175458, #204454, #167647, #25162 ) ) ;
#95485=CARTESIAN_POINT ( 'NONE',  ( -11.52460864928264961, 13.87999999999998302, 3.346683403123524858 ) ) ;
#95486=CARTESIAN_POINT ( 'NONE',  ( -10.31399889198507402, 4.822877898269746666, -6.141096068735103053 ) ) ;
#95488=VERTEX_POINT ( 'NONE', #154707 ) ;
#95507=CARTESIAN_POINT ( 'NONE',  ( 11.55950211276791251, 11.37999999999998302, 3.221476510067114329 ) ) ;
#95519=DIRECTION ( 'NONE',  ( 0.000000000000000000, 0.000000000000000000, -1.000000000000000000 ) ) ;
#95541=DIRECTION ( 'NONE',  ( 0.000000000000000000, -1.000000000000000000, 0.000000000000000000 ) ) ;
#95601=ORIENTED_EDGE ( 'NONE', *, *, #191572, .F. ) ;
#95608=CARTESIAN_POINT ( 'NONE',  ( -15.75000000000000000, 12.69999999999999929, -1.100000000000000311 ) ) ;
#95623=PRESENTATION_STYLE_ASSIGNMENT (( #29531 ) ) ;
#95661=DIRECTION ( 'NONE',  ( 0.000000000000000000, 0.000000000000000000, 1.000000000000000000 ) ) ;
#95664=CARTESIAN_POINT ( 'NONE',  ( 11.96215121607992771, 9.771664462191758105, -0.9565349792967603459 ) ) ;
#95666=ORIENTED_EDGE ( 'NONE', *, *, #117363, .F. ) ;
#95678=DIRECTION ( 'NONE',  ( 0.000000000000000000, 0.000000000000000000, 1.000000000000000000 ) ) ;
#95689=CARTESIAN_POINT ( 'NONE',  ( 12.51849242037993371, 7.545148564283970849, -4.094730316256000258 ) ) ;
#95712=CARTESIAN_POINT ( 'NONE',  ( 0.000000000000000000, 8.500000000000000000, 0.000000000000000000 ) ) ;
#95719=CARTESIAN_POINT ( 'NONE',  ( -11.97929049433705551, 11.29999999999999893, -0.7046979865771820783 ) ) ;
#95744=CARTESIAN_POINT ( 'NONE',  ( -11.95450884322492158, 8.100199754937611019, 0.5427143782397774174 ) ) ;
#95784=CARTESIAN_POINT ( 'NONE',  ( -9.604686356149276349, 3.999999999999997335, 7.193747284969079558 ) ) ;
#95788=CARTESIAN_POINT ( 'NONE',  ( 9.796344284928359514, 14.76695548050556894, -7.811462394769543849 ) ) ;
#95791=CARTESIAN_POINT ( 'NONE',  ( 8.296867357720381975, 13.24864518393002832, 8.548329535528976564 ) ) ;
#95800=CARTESIAN_POINT ( 'NONE',  ( -11.33772463945037146, 11.00902469614650236, -3.600000000000000977 ) ) ;
#95822=CARTESIAN_POINT ( 'NONE',  ( -11.82816107619417778, 7.167718870070345361, 1.885585305228718589 ) ) ;
#95824=EDGE_CURVE ( 'NONE', #124513, #45649, #184616, .T. ) ;
#95835=ADVANCED_FACE ( 'NONE', ( #89727 ), #44170, .F. ) ;
#95843=CARTESIAN_POINT ( 'NONE',  ( -9.523545777995696682, 15.37723649748560284, 7.300907475062111907 ) ) ;
#95851=CARTESIAN_POINT ( 'NONE',  ( 11.28150220813606452, 8.887219049998511977, 4.094115087793253061 ) ) ;
#95862=CARTESIAN_POINT ( 'NONE',  ( 0.000000000000000000, 7.000000000000000000, 0.000000000000000000 ) ) ;
#95903=CARTESIAN_POINT ( 'NONE',  ( -11.62998601542303945, 7.357621451758071807, 2.777426515790095696 ) ) ;
#95910=CARTESIAN_POINT ( 'NONE',  ( -11.94110265860324560, 8.911089186573638798, 1.226694517427904696 ) ) ;
#95929=CARTESIAN_POINT ( 'NONE',  ( -11.94655611907589865, 12.44799055453095882, -1.134828163062138628 ) ) ;
#95939=CARTESIAN_POINT ( 'NONE',  ( -10.90754186426655004, 4.636108433425617292, 4.485516275142084730 ) ) ;
#95942=VERTEX_POINT ( 'NONE', #10570 ) ;
#95944=FACE_OUTER_BOUND ( 'NONE', #158160, .T. ) ;
#95954=EDGE_CURVE ( 'NONE', #7565, #212473, #74525, .T. ) ;
#95960=SURFACE_STYLE_USAGE ( .BOTH. , #211796 ) ;
#95962=CARTESIAN_POINT ( 'NONE',  ( 11.43190902327453529, 13.65522128257866363, -3.649704988378122739 ) ) ;
#95968=FACE_OUTER_BOUND ( 'NONE', #113034, .T. ) ;
#95972=EDGE_CURVE ( 'NONE', #702, #7565, #96412, .T. ) ;
#95976=TOROIDAL_SURFACE ( 'NONE', #140825, 11.92000000000000348, 0.08000000000000000167 ) ;
#96011=CIRCLE ( 'NONE', #61354, 0.07999999999999961309 ) ;
#96057=DIRECTION ( 'NONE',  ( 0.000000000000000000, 1.000000000000000000, 0.000000000000000000 ) ) ;
#96075=CARTESIAN_POINT ( 'NONE',  ( 0.08053691275167890185, 14.48153890507870223, 11.99972973886013961 ) ) ;
#96092=VERTEX_POINT ( 'NONE', #162182 ) ;
#96102=ORIENTED_EDGE ( 'NONE', *, *, #37661, .F. ) ;
#96107=CARTESIAN_POINT ( 'NONE',  ( 8.812662591969752768, 13.17658495047174760, -8.076872458326402437 ) ) ;
#96129=CIRCLE ( 'NONE', #82169, 12.00000000000000178 ) ;
#96149=CARTESIAN_POINT ( 'NONE',  ( 9.171693111243110152, 14.14829661376107772, -7.667865116287802429 ) ) ;
#96183=CARTESIAN_POINT ( 'NONE',  ( -11.97181073603049839, 13.88000000000000256, -0.8318477717169578955 ) ) ;
#96198=CARTESIAN_POINT ( 'NONE',  ( 0.000000000000000000, 9.719999999999998863, 0.000000000000000000 ) ) ;
#96199=CARTESIAN_POINT ( 'NONE',  ( 11.86429981771095754, 8.354644167381561459, 1.610253852115079543 ) ) ;
#96308=ORIENTED_EDGE ( 'NONE', *, *, #16302, .T. ) ;
#96314=CARTESIAN_POINT ( 'NONE',  ( 11.52463353791760348, 13.87999999999998479, 3.346594096177638367 ) ) ;
#96338=CARTESIAN_POINT ( 'NONE',  ( -9.523113341625002448, 14.62187147401989407, 7.301473412126905593 ) ) ;
#96347=CARTESIAN_POINT ( 'NONE',  ( 11.97181073603049306, 12.22000000000000064, -0.8318477717169578955 ) ) ;
#96360=STYLED_ITEM ( 'NONE', ( #15380 ), #40567 ) ;
#96369=CARTESIAN_POINT ( 'NONE',  ( -11.52463353791760348, 9.719999999999982876, 3.346594096177640143 ) ) ;
#96410=CARTESIAN_POINT ( 'NONE',  ( 7.885016188448159546, 14.36996334327324476, 9.048771281106397169 ) ) ;
#96412=B_SPLINE_CURVE_WITH_KNOTS ( 'NONE', 3,
 ( #140627, #161108, #79844, #12695, #213027, #93997, #97193 ),
 .UNSPECIFIED., .F., .F.,
 ( 4, 3, 4 ),
 ( 0.000000000000000000, 3.302246092615816574E-05, 4.223956139718768900E-05 ),
 .UNSPECIFIED. ) ;
#96440=VECTOR ( 'NONE', #126450, 1000.000000000000000 ) ;
#96455=PLANE ( 'NONE',  #131309 ) ;
#96493=LINE ( 'NONE', #63955, #15739 ) ;
#96509=EDGE_LOOP ( 'NONE', ( #129732, #65135, #181172, #124800 ) ) ;
#96547=CARTESIAN_POINT ( 'NONE',  ( -9.569358774130439116, 4.446955548196708463, -7.167287524826070566 ) ) ;
#96551=ADVANCED_FACE ( 'NONE', ( #65482 ), #164332, .T. ) ;
#96565=CARTESIAN_POINT ( 'NONE',  ( 11.84668730067608244, 10.90000000000000036, -1.400000000000001688 ) ) ;
#96568=CARTESIAN_POINT ( 'NONE',  ( -11.33772467203841572, 12.59267152018143854, 3.599999999999999201 ) ) ;
#96576=VERTEX_POINT ( 'NONE', #99091 ) ;
#96590=ORIENTED_EDGE ( 'NONE', *, *, #204859, .F. ) ;
#96601=CYLINDRICAL_SURFACE ( 'NONE', #200626, 0.08000000000000020983 ) ;
#96607=CARTESIAN_POINT ( 'NONE',  ( 11.97929049433705373, 12.22000000000000064, 0.7046979865771783036 ) ) ;
#96610=CARTESIAN_POINT ( 'NONE',  ( 11.88168509644349058, 9.719999999999998863, -1.685788023084331400 ) ) ;
#96611=ORIENTED_EDGE ( 'NONE', *, *, #99741, .T. ) ;
#96617=EDGE_LOOP ( 'NONE', ( #164031, #95666, #39746, #144857 ) ) ;
#96668=B_SPLINE_CURVE_WITH_KNOTS ( 'NONE', 3,
 ( #58987, #5933, #156502, #171661, #188977, #125144, #191101, #108876, #57917, #174900, #73079, #121936, #23257, #139180 ),
 .UNSPECIFIED., .F., .F.,
 ( 4, 2, 2, 2, 2, 2, 4 ),
 ( 0.000000000000000000, 0.2499999999999998890, 0.3750000000000000000, 0.5000000000000000000, 0.6250000000000000000, 0.7499999999999998890, 1.000000000000000000 ),
 .UNSPECIFIED. ) ;
#96669=CARTESIAN_POINT ( 'NONE',  ( -11.97181042169641074, 11.37999999999999901, 0.8318531151397159373 ) ) ;
#96671=EDGE_CURVE ( 'NONE', #70986, #148656, #103343, .T. ) ;
#96672=CARTESIAN_POINT ( 'NONE',  ( 11.48784849554592924, 11.33049527181923111, -3.469614872287849927 ) ) ;
#96681=( BOUNDED_CURVE ( )  B_SPLINE_CURVE ( 3, ( #184741, #85126, #119831, #103520 ),
 .UNSPECIFIED., .F., .T. ) 
 B_SPLINE_CURVE_WITH_KNOTS ( ( 4, 4 ),
 ( 1.683648326080136037, 1.706346174174820041 ),
 .UNSPECIFIED. ) 
 CURVE ( )  GEOMETRIC_REPRESENTATION_ITEM ( )  RATIONAL_B_SPLINE_CURVE ( ( 1.000000000000000000, 0.9999570677684579412, 0.9999570677684579412, 1.000000000000000000 ) ) 
 REPRESENTATION_ITEM ( '' )  );
#96732=ORIENTED_EDGE ( 'NONE', *, *, #211523, .T. ) ;
#96747=CARTESIAN_POINT ( 'NONE',  ( -10.50000000000000000, 10.19999999999998153, 3.599999999999999201 ) ) ;
#96748=DIRECTION ( 'NONE',  ( 0.000000000000000000, 0.000000000000000000, -1.000000000000000000 ) ) ;
#96758=CARTESIAN_POINT ( 'NONE',  ( 11.40264643788129639, 9.090283821728826652, -6.596144476283479996 ) ) ;
#96789=CARTESIAN_POINT ( 'NONE',  ( -11.96209379583854293, 11.32792940594236519, -0.9572398070798617820 ) ) ;
#96815=CARTESIAN_POINT ( 'NONE',  ( -9.898321827459618305, 15.00000000000623857, 7.924999999990495425 ) ) ;
#96854=CARTESIAN_POINT ( 'NONE',  ( -10.47807565189556911, 4.462864196998284960, -5.860964803283929214 ) ) ;
#96858=CARTESIAN_POINT ( 'NONE',  ( 9.645118626927368766, 13.59280469987849216, -8.209452448563446580 ) ) ;
#96861=CARTESIAN_POINT ( 'NONE',  ( 9.211430769240257277, 13.21586787862255363, 9.027972232310341738 ) ) ;
#96893=CARTESIAN_POINT ( 'NONE',  ( -10.47476631618627252, 5.237304525980054137, 5.169966676860812349 ) ) ;
#96919=CARTESIAN_POINT ( 'NONE',  ( 11.81165604110238299, 7.954580463409317126, -2.158456547454505881 ) ) ;
#96921=EDGE_CURVE ( 'NONE', #45318, #96984, #213018, .T. ) ;
#96949=CARTESIAN_POINT ( 'NONE',  ( 11.01135777277262306, 13.50632581993708570, 1.399999999999998579 ) ) ;
#96970=CARTESIAN_POINT ( 'NONE',  ( -11.82276436367499883, 7.680992254652674767, -2.069180822227531635 ) ) ;
#96978=CARTESIAN_POINT ( 'NONE',  ( -11.63550830110499135, 8.311017141679082343, -2.948455737676608290 ) ) ;
#96984=VERTEX_POINT ( 'NONE', #17793 ) ;
#97000=FACE_OUTER_BOUND ( 'NONE', #83362, .T. ) ;
#97007=CARTESIAN_POINT ( 'NONE',  ( -11.82198925196379946, 4.889592154110854239, -4.884635108899213485 ) ) ;
#97011=CARTESIAN_POINT ( 'NONE',  ( -15.75000000000000000, 11.29999999999999893, -1.800000000000001155 ) ) ;
#97014=EDGE_LOOP ( 'NONE', ( #138020, #87095, #5452, #153618, #79661 ) ) ;
#97025=CARTESIAN_POINT ( 'NONE',  ( -11.84668729410370602, 12.59379487675469278, 1.399999999999998357 ) ) ;
#97029=DIRECTION ( 'NONE',  ( 0.2684563758389248433, 0.000000000000000000, 0.9632918427306597087 ) ) ;
#97035=SURFACE_SIDE_STYLE ('',( #65540 ) ) ;
#97066=DIRECTION ( 'NONE',  ( -0.000000000000000000, -1.000000000000000000, -0.000000000000000000 ) ) ;
#97075=CARTESIAN_POINT ( 'NONE',  ( -10.49139461985735977, 3.038394114823554482, -7.128631142076787164 ) ) ;
#97084=CARTESIAN_POINT ( 'NONE',  ( -11.84668730067608777, 12.59365272245204892, -1.400000000000002132 ) ) ;
#97098=VERTEX_POINT ( 'NONE', #121811 ) ;
#97117=UNCERTAINTY_MEASURE_WITH_UNIT (LENGTH_MEASURE( 1.000000000000000082E-05 ), #74601, 'distance_accuracy_value', 'NONE');
#97124=AXIS2_PLACEMENT_3D ( 'NONE', #50386, #100197, #103400 ) ;
#97142=CARTESIAN_POINT ( 'NONE',  ( 10.97031310326519282, 9.799999999999998934, -1.695146482106562269 ) ) ;
#97176=CARTESIAN_POINT ( 'NONE',  ( 10.50000000000000178, 12.69999999999998153, 3.599999999999999201 ) ) ;
#97182=ORIENTED_EDGE ( 'NONE', *, *, #3914, .F. ) ;
#97185=AXIS2_PLACEMENT_3D ( 'NONE', #36689, #136354, #4169 ) ;
#97191=ADVANCED_FACE ( 'NONE', ( #189922 ), #89710, .T. ) ;
#97193=CARTESIAN_POINT ( 'NONE',  ( 1.734723475976807094E-15, 15.42733875946000133, 11.91973154060105955 ) ) ;
#97201=( LENGTH_UNIT ( ) NAMED_UNIT ( * ) SI_UNIT ( .MILLI., .METRE. ) );
#97211=CARTESIAN_POINT ( 'NONE',  ( 9.398454900782844845, 13.71746517427355627, -7.461324637964940720 ) ) ;
#97231=CIRCLE ( 'NONE', #20963, 0.5000000000000015543 ) ;
#97234=CARTESIAN_POINT ( 'NONE',  ( -9.348561386899501002, 3.999985931113709814, -7.001914024221969512 ) ) ;
#97248=CARTESIAN_POINT ( 'NONE',  ( 8.360103901485762989, 14.02891420676280987, -8.609295381564869842 ) ) ;
#97256=FILL_AREA_STYLE ('',( #195807 ) ) ;
#97257=CARTESIAN_POINT ( 'NONE',  ( 9.898415338264832997, 12.56653357618227318, -7.886274193477667893 ) ) ;
#97267=CARTESIAN_POINT ( 'NONE',  ( 8.223666246221556619, 14.19229986755559558, -8.739774625693256027 ) ) ;
#97270=EDGE_LOOP ( 'NONE', ( #167324, #83529, #59960, #124882 ) ) ;
#97274=CARTESIAN_POINT ( 'NONE',  ( -11.06297021485807797, 13.75669301487472218, 0.9089447062504983910 ) ) ;
#97275=CARTESIAN_POINT ( 'NONE',  ( 11.84668730067608777, 11.00634727754795250, -1.400000000000001910 ) ) ;
#97276=CARTESIAN_POINT ( 'NONE',  ( 0.04160618626039885859, 14.52029232702615325, 11.99061297704356299 ) ) ;
#97287=CARTESIAN_POINT ( 'NONE',  ( 1.313174662617483834, 8.310476012147658409, 10.86148356754323885 ) ) ;
#97300=CARTESIAN_POINT ( 'NONE',  ( -9.523113340799540083, 15.37812852751596004, -7.301473413204503160 ) ) ;
#97335=EDGE_LOOP ( 'NONE', ( #60810, #183818, #184861, #77651 ) ) ;
#97373=FILL_AREA_STYLE_COLOUR ( '', #146715 ) ;
#97386=AXIS2_PLACEMENT_3D ( 'NONE', #18565, #83570, #84641 ) ;
#97389=DIRECTION ( 'NONE',  ( 0.000000000000000000, 0.000000000000000000, 1.000000000000000000 ) ) ;
#97404=( NAMED_UNIT ( * ) SI_UNIT ( $, .STERADIAN. ) SOLID_ANGLE_UNIT ( ) );
#97435=MECHANICAL_DESIGN_GEOMETRIC_PRESENTATION_REPRESENTATION('',(#176897),#194204);
#97437=LINE ( 'NONE', #213276, #132193 ) ;
#97465=CARTESIAN_POINT ( 'NONE',  ( 7.695957533950816831, 14.38956844792682688, 9.210281496461904638 ) ) ;
#97473=VECTOR ( 'NONE', #189425, 1000.000000000000000 ) ;
#97488=EDGE_CURVE ( 'NONE', #176917, #99973, #85004, .T. ) ;
#97492=EDGE_LOOP ( 'NONE', ( #68934, #44809, #26612, #21881 ) ) ;
#97501=B_SPLINE_CURVE_WITH_KNOTS ( 'NONE', 3,
 ( #172873, #74294, #140390, #24444, #125256, #107928 ),
 .UNSPECIFIED., .F., .F.,
 ( 4, 2, 4 ),
 ( 1.997645371451378118E-16, 3.619701867389574191E-05, 7.239403734759171957E-05 ),
 .UNSPECIFIED. ) ;
#97540=ORIENTED_EDGE ( 'NONE', *, *, #153308, .F. ) ;
#97546=VECTOR ( 'NONE', #186694, 1000.000000000000000 ) ;
#97548=CARTESIAN_POINT ( 'NONE',  ( -11.55950211276791428, 11.37999999999998302, 3.221476510067114329 ) ) ;
#97554=CARTESIAN_POINT ( 'NONE',  ( -11.94105721839855327, 10.07301656658874833, -1.187919402540362768 ) ) ;
#97603=LINE ( 'NONE', #12057, #47473 ) ;
#97605=VERTEX_POINT ( 'NONE', #147592 ) ;
#97624=CARTESIAN_POINT ( 'NONE',  ( -11.96209379583854293, 13.82792940594236519, -0.9572398070798617820 ) ) ;
#97637=CARTESIAN_POINT ( 'NONE',  ( -10.50000000000000355, 10.09281572507203606, 3.599999999999998312 ) ) ;
#97668=( NAMED_UNIT ( * ) SI_UNIT ( $, .STERADIAN. ) SOLID_ANGLE_UNIT ( ) );
#97682=ORIENTED_EDGE ( 'NONE', *, *, #25088, .T. ) ;
#97701=FACE_OUTER_BOUND ( 'NONE', #90780, .T. ) ;
#97705=AXIS2_PLACEMENT_3D ( 'NONE', #160636, #157454, #12237 ) ;
#97721=VERTEX_POINT ( 'NONE', #28495 ) ;
#97745=EDGE_CURVE ( 'NONE', #144610, #13289, #43756, .T. ) ;
#97750=CARTESIAN_POINT ( 'NONE',  ( 6.882015208740354772, 15.51845925587262798, -9.732639244658484401 ) ) ;
#97754=ADVANCED_FACE ( 'NONE', ( #132436 ), #12638, .T. ) ;
#97790=ORIENTED_EDGE ( 'NONE', *, *, #50048, .F. ) ;
#97796=CARTESIAN_POINT ( 'NONE',  ( -11.89321938400731860, 9.837447216393279348, -1.599605898944130189 ) ) ;
#97814=CARTESIAN_POINT ( 'NONE',  ( 9.692997807120237397, 13.38204337665774624, -8.150562841249751500 ) ) ;
#97828=CIRCLE ( 'NONE', #94282, 11.09999999999999964 ) ;
#97844=AXIS2_PLACEMENT_3D ( 'NONE', #122296, #123364, #186115 ) ;
#97855=DIRECTION ( 'NONE',  ( 6.873509095275333662E-09, -1.000000000000000000, 0.000000000000000000 ) ) ;
#97916=CARTESIAN_POINT ( 'NONE',  ( 10.11376083457019526, 13.81646513174396951, -7.343696251440634093 ) ) ;
#97945=AXIS2_PLACEMENT_3D ( 'NONE', #56932, #120949, #7085 ) ;
#97953=CARTESIAN_POINT ( 'NONE',  ( -11.13230441903222534, 5.430351611223322550, 4.009938051813186632 ) ) ;
#97966=CARTESIAN_POINT ( 'NONE',  ( 0.000000000000000000, 0.000000000000000000, 0.000000000000000000 ) ) ;
#97972=VERTEX_POINT ( 'NONE', #34871 ) ;
#97977=ORIENTED_EDGE ( 'NONE', *, *, #61570, .T. ) ;
#97979=CARTESIAN_POINT ( 'NONE',  ( 9.528027380766250332, 12.67459186834941320, -7.221597964460605645 ) ) ;
#97992=CARTESIAN_POINT ( 'NONE',  ( 11.84100621633422179, 9.989584257766640718, -1.444132586618106728 ) ) ;
#97999=EDGE_CURVE ( 'NONE', #163825, #145411, #114476, .T. ) ;
#98007=MECHANICAL_DESIGN_GEOMETRIC_PRESENTATION_REPRESENTATION('',(#163702),#149782);
#98026=SURFACE_STYLE_FILL_AREA ( #114324 ) ;
#98031=CARTESIAN_POINT ( 'NONE',  ( -11.86531349175653105, 7.722710556319649200, 1.810764415104959779 ) ) ;
#98040=CARTESIAN_POINT ( 'NONE',  ( -11.81671913857781853, 8.671847271708829297, 2.110070278039765768 ) ) ;
#98050=ORIENTED_EDGE ( 'NONE', *, *, #58273, .F. ) ;
#98056=CARTESIAN_POINT ( 'NONE',  ( -11.94105721237522921, 12.57259215598210744, -1.187919463087249605 ) ) ;
#98085=PRESENTATION_STYLE_ASSIGNMENT (( #95960 ) ) ;
#98088=CARTESIAN_POINT ( 'NONE',  ( -10.59763834280244232, 13.79999999999999716, -3.303285708550594890 ) ) ;
#98102=CIRCLE ( 'NONE', #170742, 0.08000000000000052902 ) ;
#98123=EDGE_CURVE ( 'NONE', #85120, #144017, #202225, .T. ) ;
#98151=AXIS2_PLACEMENT_3D ( 'NONE', #25102, #40313, #91204 ) ;
#98154=ORIENTED_EDGE ( 'NONE', *, *, #183845, .F. ) ;
#98160=CIRCLE ( 'NONE', #60097, 11.09999999999999964 ) ;
#98259=CARTESIAN_POINT ( 'NONE',  ( 11.94980361058169116, 10.19999999999999929, -1.099999999999998535 ) ) ;
#98262=CARTESIAN_POINT ( 'NONE',  ( 11.89197415570408900, 9.799999999999998934, -0.8055989572471863314 ) ) ;
#98287=CARTESIAN_POINT ( 'NONE',  ( -9.956244568750863166, 5.504298494775027528, -6.025958004757996811 ) ) ;
#98309=CARTESIAN_POINT ( 'NONE',  ( 9.348030350560099677, 12.83729060537138089, -6.611360045021780429 ) ) ;
#98326=DIRECTION ( 'NONE',  ( -0.7806247490453480653, -4.396526966619892032E-05, 0.6249999993959538536 ) ) ;
#98352=ADVANCED_FACE ( 'NONE', ( #187532 ), #136675, .F. ) ;
#98363=DIRECTION ( 'NONE',  ( -0.000000000000000000, -1.000000000000000000, -0.000000000000000000 ) ) ;
#98365=CARTESIAN_POINT ( 'NONE',  ( 11.04986227068298277, 11.10939997844336347, -1.056429153205399984 ) ) ;
#98392=FACE_OUTER_BOUND ( 'NONE', #109452, .T. ) ;
#98398=CARTESIAN_POINT ( 'NONE',  ( 11.94105721237523277, 10.19999999999999929, 1.187919463087244720 ) ) ;
#98419=ORIENTED_EDGE ( 'NONE', *, *, #35037, .F. ) ;
#98421=PRESENTATION_STYLE_ASSIGNMENT (( #210012 ) ) ;
#98425=PLANE ( 'NONE',  #158752 ) ;
#98438=CARTESIAN_POINT ( 'NONE',  ( 0.000000000000000000, 11.29999999999999893, 0.000000000000000000 ) ) ;
#98443=CIRCLE ( 'NONE', #32733, 12.00000000000000178 ) ;
#98451=CARTESIAN_POINT ( 'NONE',  ( -9.497657700844911233, 15.42018113367679888, 7.334628298493624854 ) ) ;
#98457=STYLED_ITEM ( 'NONE', ( #171071 ), #180544 ) ;
#98472=CARTESIAN_POINT ( 'NONE',  ( -9.367496997608917297, 14.57669131241553728, -7.413898975919227752 ) ) ;
#98516=CARTESIAN_POINT ( 'NONE',  ( 7.130034971365033059, 14.53133652881233573, 9.655242375037330405 ) ) ;
#98524=B_SPLINE_CURVE_WITH_KNOTS ( 'NONE', 3,
 ( #193060, #161657, #44713, #110820, #202641, #134506, #166980, #84649 ),
 .UNSPECIFIED., .F., .F.,
 ( 4, 2, 2, 4 ),
 ( 0.000000000000000000, 0.0004845678193365327946, 0.0009691356386730655892, 0.001938271277346135515 ),
 .UNSPECIFIED. ) ;
#98571=ORIENTED_EDGE ( 'NONE', *, *, #193499, .T. ) ;
#98587=CARTESIAN_POINT ( 'NONE',  ( -15.75000000000000000, 12.69999999999998153, 3.199999999999997957 ) ) ;
#98597=CARTESIAN_POINT ( 'NONE',  ( -11.48806469435255373, 11.33089772872447121, 3.468902948106700634 ) ) ;
#98607=PRESENTATION_STYLE_ASSIGNMENT (( #128005 ) ) ;
#98624=EDGE_CURVE ( 'NONE', #197365, #159860, #133752, .T. ) ;
#98646=DIRECTION ( 'NONE',  ( -0.000000000000000000, -1.000000000000000000, -0.000000000000000000 ) ) ;
#98658=EDGE_CURVE ( 'NONE', #113953, #198880, #108495, .T. ) ;
#98660=LINE ( 'NONE', #212381, #162253 ) ;
#98674=CARTESIAN_POINT ( 'NONE',  ( -11.41381678389398502, 12.57120581758917055, 3.704697885617667996 ) ) ;
#98681=ORIENTED_EDGE ( 'NONE', *, *, #85583, .T. ) ;
#98686=CARTESIAN_POINT ( 'NONE',  ( -10.56536251450128994, 9.840389374505219777, 3.404319718479181578 ) ) ;
#98692=( NAMED_UNIT ( * ) SI_UNIT ( $, .STERADIAN. ) SOLID_ANGLE_UNIT ( ) );
#98712=CARTESIAN_POINT ( 'NONE',  ( 11.86145016429273191, 12.59412123665269512, 1.099999999999996758 ) ) ;
#98720=CARTESIAN_POINT ( 'NONE',  ( -10.10575425844435138, 4.358269247758318699, 5.859476710806498900 ) ) ;
#98721=ORIENTED_EDGE ( 'NONE', *, *, #20380, .F. ) ;
#98727=EDGE_CURVE ( 'NONE', #21587, #117081, #93719, .T. ) ;
#98753=CARTESIAN_POINT ( 'NONE',  ( -9.421011374587449083, 15.43484797186988011, -7.432750069690781558 ) ) ;
#98761=B_SPLINE_CURVE_WITH_KNOTS ( 'NONE', 3,
 ( #88850, #43303, #175428, #138664, #174372, #121416 ),
 .UNSPECIFIED., .F., .F.,
 ( 4, 2, 4 ),
 ( 0.000000000000000000, 0.0003778774010236168619, 0.0007557548020472337237 ),
 .UNSPECIFIED. ) ;
#98770=ADVANCED_FACE ( 'NONE', ( #178771 ), #62861, .F. ) ;
#98777=CARTESIAN_POINT ( 'NONE',  ( -15.75000000000000000, 10.90000000000000036, -3.600000000000002309 ) ) ;
#98783=DIRECTION ( 'NONE',  ( 0.000000000000000000, -1.000000000000000000, 0.000000000000000000 ) ) ;
#98810=CIRCLE ( 'NONE', #157558, 0.5000000000000016653 ) ;
#98822=EDGE_CURVE ( 'NONE', #151228, #51181, #213156, .T. ) ;
#98839=DIRECTION ( 'NONE',  ( 0.000000000000000000, 1.000000000000000000, 0.000000000000000000 ) ) ;
#98841=CARTESIAN_POINT ( 'NONE',  ( 11.88235317400313917, 11.25664239773029607, 0.9089793033029930358 ) ) ;
#98870=CARTESIAN_POINT ( 'NONE',  ( 9.940066813768632770, 11.27778190843423545, -8.363988134642921679 ) ) ;
#98891=CARTESIAN_POINT ( 'NONE',  ( 11.35605497252127272, 11.11418145951645542, -3.553547709190210124 ) ) ;
#98904=( GEOMETRIC_REPRESENTATION_CONTEXT ( 3 ) GLOBAL_UNCERTAINTY_ASSIGNED_CONTEXT ( ( #76828 ) ) GLOBAL_UNIT_ASSIGNED_CONTEXT ( ( #12589, #79733, #127522 ) ) REPRESENTATION_CONTEXT ( 'NONE', 'WORKASPACE' ) );
#98911=CARTESIAN_POINT ( 'NONE',  ( -4.900611166869239810E-10, 15.51845925587262798, -11.92000000000000171 ) ) ;
#98914=DIRECTION ( 'NONE',  ( 7.993605777301127091E-15, 0.000000000000000000, -1.000000000000000000 ) ) ;
#98922=CARTESIAN_POINT ( 'NONE',  ( -9.645001968711920171, 4.042125922905831281, 6.587946042608958663 ) ) ;
#98936=CIRCLE ( 'NONE', #185344, 0.5000000000000008882 ) ;
#98945=EDGE_CURVE ( 'NONE', #159860, #142717, #36756, .T. ) ;
#98948=EDGE_CURVE ( 'NONE', #51181, #116972, #194185, .T. ) ;
#98950=CIRCLE ( 'NONE', #92006, 0.08000000000000014044 ) ;
#98970=CARTESIAN_POINT ( 'NONE',  ( 7.864583096620019198, 14.80247548031949201, -8.638774414189107631 ) ) ;
#99019=ADVANCED_FACE ( 'NONE', ( #15164 ), #64981, .F. ) ;
#99022=CARTESIAN_POINT ( 'NONE',  ( -9.549485338732782935, 14.79470350949243951, 7.267374014142787608 ) ) ;
#99023=ORIENTED_EDGE ( 'NONE', *, *, #195893, .T. ) ;
#99030=MECHANICAL_DESIGN_GEOMETRIC_PRESENTATION_REPRESENTATION('',(#119793),#133689);
#99031=CARTESIAN_POINT ( 'NONE',  ( 9.843279382890161244, 11.92209134021086037, -6.866670447127348531 ) ) ;
#99038=CARTESIAN_POINT ( 'NONE',  ( 8.641284494170047736, 13.75145223737358613, -8.262855152994331931 ) ) ;
#99083=CARTESIAN_POINT ( 'NONE',  ( -11.68315434942572217, 7.483877878977486020, -2.545616869505754831 ) ) ;
#99091=CARTESIAN_POINT ( 'NONE',  ( -10.50060100873255031, 5.377693802073529206, 5.808388628131297970 ) ) ;
#99127=ORIENTED_EDGE ( 'NONE', *, *, #165199, .F. ) ;
#99142=CARTESIAN_POINT ( 'NONE',  ( 11.44779964734654776, 13.49810470129596318, -3.599999963171534478 ) ) ;
#99158=CARTESIAN_POINT ( 'NONE',  ( 9.649010003797931390, 3.730310916805957167, 7.134817918383254742 ) ) ;
#99209=CARTESIAN_POINT ( 'NONE',  ( -11.89844258446855285, 13.82852689329959439, 1.560502987793273233 ) ) ;
#99231=UNCERTAINTY_MEASURE_WITH_UNIT (LENGTH_MEASURE( 1.000000000000000082E-05 ), #194148, 'distance_accuracy_value', 'NONE');
#99232=CARTESIAN_POINT ( 'NONE',  ( 11.06298571000738917, 11.25678692636136979, 0.9087567263023067499 ) ) ;
#99256=CARTESIAN_POINT ( 'NONE',  ( -1.878313713276733132, 14.99999999999692157, -12.68000002627077905 ) ) ;
#99258=CARTESIAN_POINT ( 'NONE',  ( -10.47476631618627252, 5.237304525980054137, 5.169966676860812349 ) ) ;
#99271=AXIS2_PLACEMENT_3D ( 'NONE', #115506, #165258, #49387 ) ;
#99290=( NAMED_UNIT ( * ) SI_UNIT ( $, .STERADIAN. ) SOLID_ANGLE_UNIT ( ) );
#99321=ORIENTED_EDGE ( 'NONE', *, *, #162091, .T. ) ;
#99325=DIRECTION ( 'NONE',  ( 1.000000000000000000, -0.000000000000000000, -0.000000000000000000 ) ) ;
#99349=EDGE_CURVE ( 'NONE', #62746, #57689, #57235, .T. ) ;
#99354=CARTESIAN_POINT ( 'NONE',  ( -10.81015953665327345, 5.524082113754967160, -6.547048903644186346 ) ) ;
#99369=LINE ( 'NONE', #180604, #7651 ) ;
#99378=CARTESIAN_POINT ( 'NONE',  ( 10.43308898320764833, 8.755712671243168543, -3.803521280157781792 ) ) ;
#99381=ORIENTED_EDGE ( 'NONE', *, *, #92162, .F. ) ;
#99383=COLOUR_RGB ( '', 0.72549020, 0.75294118, 0.79215686) ;
#99389=FACE_OUTER_BOUND ( 'NONE', #20636, .T. ) ;
#99404=DIRECTION ( 'NONE',  ( 0.000000000000000000, 0.000000000000000000, -1.000000000000000000 ) ) ;
#99407=CARTESIAN_POINT ( 'NONE',  ( -11.97929049433705373, 12.22000000000000064, -0.7046979865771834106 ) ) ;
#99461=SURFACE_SIDE_STYLE ('',( #181749 ) ) ;
#99483=CARTESIAN_POINT ( 'NONE',  ( -11.96533679318059917, 9.847539888129954733, 0.9151144679398905968 ) ) ;
#99496=DIRECTION ( 'NONE',  ( 0.000000000000000000, -0.000000000000000000, 1.000000000000000000 ) ) ;
#99531=VERTEX_POINT ( 'NONE', #58346 ) ;
#99551=CARTESIAN_POINT ( 'NONE',  ( 11.49966000274946332, 11.24232845564745809, 3.429881629453402248 ) ) ;
#99633=CARTESIAN_POINT ( 'NONE',  ( 7.499003223742838564, 15.48049048347138879, 9.369984475626267795 ) ) ;
#99663=SURFACE_STYLE_FILL_AREA ( #32532 ) ;
#99669=ORIENTED_EDGE ( 'NONE', *, *, #121307, .T. ) ;
#99689=VECTOR ( 'NONE', #201119, 1000.000000000000000 ) ;
#99705=ORIENTED_EDGE ( 'NONE', *, *, #200040, .F. ) ;
#99710=CARTESIAN_POINT ( 'NONE',  ( -15.75000000000000000, 12.30000000000000071, -1.800000000000001155 ) ) ;
#99729=DIRECTION ( 'NONE',  ( 0.000000000000000000, -1.000000000000000000, -1.804652791718263484E-16 ) ) ;
#99741=EDGE_CURVE ( 'NONE', #143955, #66223, #2257, .T. ) ;
#99743=( NAMED_UNIT ( * ) PLANE_ANGLE_UNIT ( ) SI_UNIT ( $, .RADIAN. ) );
#99781=CARTESIAN_POINT ( 'NONE',  ( -10.37901820579008039, 4.889546506944066451, 5.358714317323078014 ) ) ;
#99782=ORIENTED_EDGE ( 'NONE', *, *, #168889, .T. ) ;
#99797=AXIS2_PLACEMENT_3D ( 'NONE', #21590, #5337, #198234 ) ;
#99800=ORIENTED_EDGE ( 'NONE', *, *, #157010, .F. ) ;
#99834=CARTESIAN_POINT ( 'NONE',  ( -10.17648486856286816, 3.632311211988387800, -6.360307065827860207 ) ) ;
#99841=CARTESIAN_POINT ( 'NONE',  ( -11.84104725192624130, 12.49016462548582851, -1.443823348526935169 ) ) ;
#99845=DIRECTION ( 'NONE',  ( 0.000000000000000000, 1.000000000000000000, 0.000000000000000000 ) ) ;
#99848=COLOUR_RGB ( '', 0.09019608, 0.27058824, 0.51372549) ;
#99857=DIRECTION ( 'NONE',  ( -0.000000000000000000, -1.000000000000000000, -0.000000000000000000 ) ) ;
#99868=DIRECTION ( 'NONE',  ( -0.000000000000000000, -1.000000000000000000, -0.000000000000000000 ) ) ;
#99900=DIRECTION ( 'NONE',  ( -1.124869321039521280E-29, -7.437565543542506798E-15, -1.000000000000000000 ) ) ;
#99903=EDGE_LOOP ( 'NONE', ( #197833, #60111, #208572, #135316 ) ) ;
#99930=CARTESIAN_POINT ( 'NONE',  ( 10.17148340815012020, 11.75186938811109627, -7.510838954888964025 ) ) ;
#99941=CARTESIAN_POINT ( 'NONE',  ( -8.150208238660177074, 14.48038068602284056, 8.818988908991837405 ) ) ;
#99967=CARTESIAN_POINT ( 'NONE',  ( -11.07790593930098311, 9.799999999999998934, 0.6999999999999992895 ) ) ;
#99971=CARTESIAN_POINT ( 'NONE',  ( 0.08053691275167890185, 19.00000000000000000, 11.99972973886014316 ) ) ;
#99973=VERTEX_POINT ( 'NONE', #48502 ) ;
#99986=AXIS2_PLACEMENT_3D ( 'NONE', #173652, #185583, #155240 ) ;
#99998=CARTESIAN_POINT ( 'NONE',  ( 10.50000000000000178, 12.69999999999999929, -3.600000000000000977 ) ) ;
#100006=VECTOR ( 'NONE', #99868, 1000.000000000000000 ) ;
#100035=ORIENTED_EDGE ( 'NONE', *, *, #150613, .T. ) ;
#100057=CARTESIAN_POINT ( 'NONE',  ( -11.52570357830391323, 8.091488070261075194, -2.173620758456770830 ) ) ;
#100076=CARTESIAN_POINT ( 'NONE',  ( -9.438074502436650803, 15.48601905264195899, 7.411038320713698724 ) ) ;
#100084=CARTESIAN_POINT ( 'NONE',  ( 10.24619468639153652, 10.82263080639484976, -6.252197070581264171 ) ) ;
#100088=CARTESIAN_POINT ( 'NONE',  ( 11.97929049433705728, 13.88000000000000078, -0.7046979865771821894 ) ) ;
#100092=CARTESIAN_POINT ( 'NONE',  ( 7.304951286220124906, 14.53038845894318953, -9.465418723554037683 ) ) ;
#100099=CARTESIAN_POINT ( 'NONE',  ( 11.07790593930098311, 13.79999999999999893, -0.7000000000000009548 ) ) ;
#100121=CARTESIAN_POINT ( 'NONE',  ( -11.89942855770814134, 11.29999999999999893, -0.7000000000000009548 ) ) ;
#100122=CARTESIAN_POINT ( 'NONE',  ( -4.779899193377088906, 14.55303452941223341, -10.96779284377108077 ) ) ;
#100151=EDGE_CURVE ( 'NONE', #183827, #181742, #101502, .T. ) ;
#100155=ADVANCED_FACE ( 'NONE', ( #214135 ), #68975, .F. ) ;
#100159=SURFACE_SIDE_STYLE ('',( #34088 ) ) ;
#100187=DIRECTION ( 'NONE',  ( 0.1510067114093955887, 0.000000000000000000, 0.9885327375000383388 ) ) ;
#100190=CARTESIAN_POINT ( 'NONE',  ( 11.52901446936659013, 13.79425527467587465, -3.330874149800854944 ) ) ;
#100197=DIRECTION ( 'NONE',  ( 0.9486832980505138790, -0.3162277660168376636, -3.312310031615527152E-15 ) ) ;
#100254=( NAMED_UNIT ( * ) SI_UNIT ( $, .STERADIAN. ) SOLID_ANGLE_UNIT ( ) );
#100256=CARTESIAN_POINT ( 'NONE',  ( -15.75000000000000000, 9.799999999999998934, -1.800000000000001155 ) ) ;
#100264=ADVANCED_FACE ( 'NONE', ( #21290 ), #196030, .T. ) ;
#100299=B_SPLINE_CURVE_WITH_KNOTS ( 'NONE', 3,
 ( #196643, #77551, #46148, #143674, #163089, #177198, #64506, #27741, #80764, #180390, #129595, #113333, #93836, #195582, #112261, #160949 ),
 .UNSPECIFIED., .F., .F.,
 ( 4, 2, 2, 2, 2, 2, 2, 4 ),
 ( 8.553866477534004096E-06, 0.002693891933807479599, 0.004036560967472453514, 0.005379230001137425693, 0.006721899034802396138, 0.008064568068467368317, 0.009407237102132339629, 0.01074990613579731094 ),
 .UNSPECIFIED. ) ;
#100305=CARTESIAN_POINT ( 'NONE',  ( 0.3554123170485448124, 15.00000000000058265, -12.67999999502907471 ) ) ;
#100307=CARTESIAN_POINT ( 'NONE',  ( -10.07159190936562432, 5.946254181132138328, -5.792974557957699666 ) ) ;
#100337=( NAMED_UNIT ( * ) SI_UNIT ( $, .STERADIAN. ) SOLID_ANGLE_UNIT ( ) );
#100364=CARTESIAN_POINT ( 'NONE',  ( -10.87339650836132776, 5.131772588966429183, -5.487095527168452058 ) ) ;
#100406=CARTESIAN_POINT ( 'NONE',  ( -10.14895191580505163, 4.000029896383376027, -7.601392964056682189 ) ) ;
#100421=CARTESIAN_POINT ( 'NONE',  ( 11.87652835678391128, 6.750173569295289333, -1.734648985301914470 ) ) ;
#100430=EDGE_LOOP ( 'NONE', ( #196941, #25979 ) ) ;
#100433=CARTESIAN_POINT ( 'NONE',  ( 10.67342974040751180, 8.362853195376180437, 3.128047310392558344 ) ) ;
#100444=CARTESIAN_POINT ( 'NONE',  ( 7.325202985640204112, 14.51512205016421397, -9.507936040486299589 ) ) ;
#100449=CARTESIAN_POINT ( 'NONE',  ( -11.04536101718726293, 13.40000000000000036, -1.100000000000002087 ) ) ;
#100483=TOROIDAL_SURFACE ( 'NONE', #155855, 11.92000000000000171, 0.08000000000000000167 ) ;
#100489=CARTESIAN_POINT ( 'NONE',  ( 0.000000000000000000, 4.518459255872631530, 0.000000000000000000 ) ) ;
#100491=( BOUNDED_SURFACE ( )  B_SPLINE_SURFACE ( 3, 2, ( 
 ( #17845, #65534, #62364 ),
 ( #112254, #100190, #128526 ),
 ( #131680, #115444, #146845 ),
 ( #33064, #178267, #95962 ),
 ( #162016, #99142, #165191 ),
 ( #16785, #82868, #148946 ) ),
 .UNSPECIFIED., .F., .F., .T. ) 
 B_SPLINE_SURFACE_WITH_KNOTS ( ( 4, 2, 4 ),
 ( 3, 3 ),
 ( 0.000000000000000000, 0.0003831416164015018179, 0.0007662832328030036357 ),
 ( 0.000000000000000000, 1.000000000000000000 ),
 .UNSPECIFIED. ) 
 GEOMETRIC_REPRESENTATION_ITEM ( )  RATIONAL_B_SPLINE_SURFACE ( (
 ( 1.000000000000000000, 0.7071067811865399122, 1.000000000000000000),
 ( 1.000000000000000000, 0.6829713513653468127, 1.000000000000000000),
 ( 1.000000000000000000, 0.6534833722372194176, 1.000000000000000000),
 ( 1.000000000000000000, 0.6054027484662655167, 1.000000000000000000),
 ( 1.000000000000000000, 0.5875453974414891478, 1.000000000000000000),
 ( 1.000000000000000000, 0.5879095031487528988, 1.000000000000000000) ) ) 
 REPRESENTATION_ITEM ( '' )  SURFACE ( )  );
#100576=CARTESIAN_POINT ( 'NONE',  ( -9.608183788732286956, 15.11835436368665420, 7.189075342704710714 ) ) ;
#100637=CARTESIAN_POINT ( 'NONE',  ( 6.928203230280114866, 14.53133650447934144, 9.797958971139216544 ) ) ;
#100659=EDGE_CURVE ( 'NONE', #121123, #119038, #161558, .T. ) ;
#100701=COLOUR_RGB ( '', 0.09019608, 0.27058824, 0.51372549) ;
#100705=SURFACE_STYLE_FILL_AREA ( #129043 ) ;
#100720=CARTESIAN_POINT ( 'NONE',  ( -11.13119402894544763, 7.260262539292284600, -4.367170956698847029 ) ) ;
#100747=CARTESIAN_POINT ( 'NONE',  ( 11.33772463945036790, 10.90000000000000036, -3.600000000000002309 ) ) ;
#100767=DIRECTION ( 'NONE',  ( -0.000000000000000000, -1.000000000000000000, -0.000000000000000000 ) ) ;
#100795=FACE_OUTER_BOUND ( 'NONE', #200379, .T. ) ;
#100805=( NAMED_UNIT ( * ) PLANE_ANGLE_UNIT ( ) SI_UNIT ( $, .RADIAN. ) );
#100832=DIRECTION ( 'NONE',  ( 0.000000000000000000, 0.000000000000000000, -1.000000000000000000 ) ) ;
#100834=CARTESIAN_POINT ( 'NONE',  ( 11.01135777277262306, 10.90000000000000036, -1.400000000000001910 ) ) ;
#100835=CARTESIAN_POINT ( 'NONE',  ( -10.62873463776380056, 9.799999999999998934, -3.200000000000001510 ) ) ;
#100847=ORIENTED_EDGE ( 'NONE', *, *, #208563, .F. ) ;
#100857=AXIS2_PLACEMENT_3D ( 'NONE', #132458, #59686, #72732 ) ;
#100866=CARTESIAN_POINT ( 'NONE',  ( -9.549485338617042629, 15.20529649091228919, -7.267374014294610163 ) ) ;
#100887=CARTESIAN_POINT ( 'NONE',  ( 11.80248046418316044, 12.30000000000000071, -1.695421849633145017 ) ) ;
#100965=CARTESIAN_POINT ( 'NONE',  ( -11.65681998539108655, 6.358950688113277572, -4.978640985104797245 ) ) ;
#100968=PRESENTATION_STYLE_ASSIGNMENT (( #133520 ) ) ;
#100977=CARTESIAN_POINT ( 'NONE',  ( 9.963343620504341303, 12.35838256557349979, -7.799456358664951239 ) ) ;
#100994=CARTESIAN_POINT ( 'NONE',  ( 0.000000000000000000, 4.000007913748540922, 0.000000000000000000 ) ) ;
#101021=B_SPLINE_CURVE_WITH_KNOTS ( 'NONE', 3,
 ( #47806, #161541, #78135, #162603, #131223, #180965 ),
 .UNSPECIFIED., .F., .F.,
 ( 4, 2, 4 ),
 ( 0.000000000000000000, 0.0003845013059668467856, 0.0007690026119336935712 ),
 .UNSPECIFIED. ) ;
#101060=AXIS2_PLACEMENT_3D ( 'NONE', #109480, #191699, #91044 ) ;
#101078=CARTESIAN_POINT ( 'NONE',  ( 8.655961103042326243, 13.72543968248328561, -9.385390936148914065 ) ) ;
#101096=CARTESIAN_POINT ( 'NONE',  ( 11.88172094500853504, 13.87999994398406045, -1.685553348215862446 ) ) ;
#101098=( BOUNDED_SURFACE ( )  B_SPLINE_SURFACE ( 3, 2, ( 
 ( #73825, #89028, #142062 ),
 ( #6669, #75959, #7738 ),
 ( #27198, #191822, #122675 ),
 ( #60773, #139919, #22912 ),
 ( #57581, #109605, #126932 ),
 ( #175610, #41353, #157224 ) ),
 .UNSPECIFIED., .F., .F., .T. ) 
 B_SPLINE_SURFACE_WITH_KNOTS ( ( 4, 2, 4 ),
 ( 3, 3 ),
 ( 0.000000000000000000, 0.0003754689591423960443, 0.0007509379182847920886 ),
 ( 0.000000000000000000, 1.000000000000000000 ),
 .UNSPECIFIED. ) 
 GEOMETRIC_REPRESENTATION_ITEM ( )  RATIONAL_B_SPLINE_SURFACE ( (
 ( 1.000000000000000000, 0.7071067811865551223, 1.000000000000000000),
 ( 1.000000000000000000, 0.7018599272026829761, 1.000000000000000000),
 ( 1.000000000000000000, 0.6927733177256546471, 1.000000000000000000),
 ( 1.000000000000000000, 0.6772007068877438085, 1.000000000000000000),
 ( 1.000000000000000000, 0.6709974581634302604, 1.000000000000000000),
 ( 1.000000000000000000, 0.6711954675835395401, 1.000000000000000000) ) ) 
 REPRESENTATION_ITEM ( '' )  SURFACE ( )  );
#101103=ADVANCED_FACE ( 'NONE', ( #144723 ), #102789, .F. ) ;
#101132=CARTESIAN_POINT ( 'NONE',  ( 0.000000000000000000, 11.29999999999999893, 0.000000000000000000 ) ) ;
#101138=CARTESIAN_POINT ( 'NONE',  ( 11.86145017031113902, 13.50581953513848710, -1.100000000000000533 ) ) ;
#101145=CARTESIAN_POINT ( 'NONE',  ( 10.51568781791557328, 11.11256730203912468, 3.554797817682051164 ) ) ;
#101193=CIRCLE ( 'NONE', #90868, 0.08000000000000014044 ) ;
#101199=CARTESIAN_POINT ( 'NONE',  ( -10.83760360872516060, 4.885615726745599297, 4.963138928152970308 ) ) ;
#101202=ORIENTED_EDGE ( 'NONE', *, *, #207506, .T. ) ;
#101222=ADVANCED_FACE ( 'NONE', ( #209280 ), #54896, .T. ) ;
#101241=ORIENTED_EDGE ( 'NONE', *, *, #148232, .T. ) ;
#101245=CARTESIAN_POINT ( 'NONE',  ( -11.92619526913700057, 19.00000000000000000, -1.328859060402686199 ) ) ;
#101315=CARTESIAN_POINT ( 'NONE',  ( -11.89321938400720491, 13.76255278360659062, 1.599605898944226334 ) ) ;
#101317=CARTESIAN_POINT ( 'NONE',  ( 0.000000000000000000, 3.481548657788671619, 0.000000000000000000 ) ) ;
#101332=( NAMED_UNIT ( * ) SI_UNIT ( $, .STERADIAN. ) SOLID_ANGLE_UNIT ( ) );
#101366=CARTESIAN_POINT ( 'NONE',  ( 0.3554123170487776817, 16.00000000000087397, -12.67999999502907649 ) ) ;
#101368=CARTESIAN_POINT ( 'NONE',  ( -10.48266952940149466, 5.268049057482275366, -5.154014898524191146 ) ) ;
#101408=CARTESIAN_POINT ( 'NONE',  ( 0.000000000000000000, 12.30000000000000071, 0.000000000000000000 ) ) ;
#101412=DIRECTION ( 'NONE',  ( 0.000000000000000000, 0.000000000000000000, -1.000000000000000000 ) ) ;
#101413=CARTESIAN_POINT ( 'NONE',  ( -11.86145016429273191, 10.19999999999999929, 1.099999999999996758 ) ) ;
#101430=DIRECTION ( 'NONE',  ( -0.2150645590070936197, 0.8781765503997437383, 0.4272624273056206401 ) ) ;
#101472=CARTESIAN_POINT ( 'NONE',  ( -10.96415609372974131, 4.387140345944800401, -6.371816014364277692 ) ) ;
#101488=VERTEX_POINT ( 'NONE', #117995 ) ;
#101491=CARTESIAN_POINT ( 'NONE',  ( 9.977304178207173635, 9.828474135482244023, 6.693966201985774411 ) ) ;
#101502=LINE ( 'NONE', #151334, #168349 ) ;
#101503=CARTESIAN_POINT ( 'NONE',  ( 9.273181387935053976, 13.51005744372143091, 6.801679163151792551 ) ) ;
#101512=CARTESIAN_POINT ( 'NONE',  ( -11.86145016429273014, 13.40000000000000036, -1.100000000000002087 ) ) ;
#101513=CARTESIAN_POINT ( 'NONE',  ( 7.129428853186368542, 14.53091783984007357, -9.655670968535163823 ) ) ;
#101517=CARTESIAN_POINT ( 'NONE',  ( 11.81905481421901705, 11.25735655617266673, -1.592167362352180149 ) ) ;
#101526=AXIS2_PLACEMENT_3D ( 'NONE', #58550, #210110, #160317 ) ;
#101529=( LENGTH_UNIT ( ) NAMED_UNIT ( * ) SI_UNIT ( .MILLI., .METRE. ) );
#101531=CARTESIAN_POINT ( 'NONE',  ( -15.75000000000000000, 10.19999999999999929, 0.6999999999999992895 ) ) ;
#101535=AXIS2_PLACEMENT_3D ( 'NONE', #108755, #159569, #90311 ) ;
#101557=DIRECTION ( 'NONE',  ( -0.000000000000000000, -1.000000000000000000, -0.000000000000000000 ) ) ;
#101579=ORIENTED_EDGE ( 'NONE', *, *, #212713, .T. ) ;
#101610=CARTESIAN_POINT ( 'NONE',  ( -11.89942855770813956, 9.799999999999998934, 0.6999999999999992895 ) ) ;
#101621=AXIS2_PLACEMENT_3D ( 'NONE', #53472, #19892, #119609 ) ;
#101626=CARTESIAN_POINT ( 'NONE',  ( -11.94105721237523277, 19.00000000000000000, -1.187919463087249827 ) ) ;
#101629=CARTESIAN_POINT ( 'NONE',  ( 9.283847064513500058, 11.43438320747982750, -7.606630335864923431 ) ) ;
#101631=ADVANCED_FACE ( 'NONE', ( #202348 ), #170940, .F. ) ;
#101638=B_SPLINE_CURVE_WITH_KNOTS ( 'NONE', 3,
 ( #87836, #133420, #199426, #83555, #184247, #18550 ),
 .UNSPECIFIED., .F., .F.,
 ( 4, 2, 4 ),
 ( 0.000000000000000000, 0.0003767011250903908558, 0.0007534022501807817115 ),
 .UNSPECIFIED. ) ;
#101645=CARTESIAN_POINT ( 'NONE',  ( 11.89942855770814312, 12.30000000000000071, -0.7000000000000009548 ) ) ;
#101666=DIRECTION ( 'NONE',  ( 0.000000000000000000, 0.000000000000000000, 1.000000000000000000 ) ) ;
#101675=SURFACE_STYLE_FILL_AREA ( #117993 ) ;
#101677=CARTESIAN_POINT ( 'NONE',  ( 9.305047017613615523, 3.481540744127370690, 7.450000000000001954 ) ) ;
#101682=CARTESIAN_POINT ( 'NONE',  ( -15.75000000000000000, 13.79999999999998295, 3.199999999999997957 ) ) ;
#101685=COLOUR_RGB ( '', 0.66274510, 0.83137255, 0.94901961) ;
#101713=EDGE_CURVE ( 'NONE', #181174, #112981, #96011, .T. ) ;
#101734=AXIS2_PLACEMENT_3D ( 'NONE', #77703, #207702, #143823 ) ;
#101740=EDGE_CURVE ( 'NONE', #63230, #53115, #70247, .T. ) ;
#101745=EDGE_CURVE ( 'NONE', #37534, #61789, #109099, .T. ) ;
#101764=CARTESIAN_POINT ( 'NONE',  ( -9.970593900173907898, 5.552053933461305490, 5.997145116287158295 ) ) ;
#101774=CARTESIAN_POINT ( 'NONE',  ( -11.48243876534946040, 11.29999999999998117, 3.199999999999997957 ) ) ;
#101789=CARTESIAN_POINT ( 'NONE',  ( -11.94311415714975588, 8.978930693142787689, 0.6090307097988665319 ) ) ;
#101814=CARTESIAN_POINT ( 'NONE',  ( 1.500000000000035971, 7.000000000000000000, 9.886859966642587594 ) ) ;
#101818=FACE_OUTER_BOUND ( 'NONE', #25296, .T. ) ;
#101834=AXIS2_PLACEMENT_3D ( 'NONE', #63150, #80465, #96748 ) ;
#101841=DIRECTION ( 'NONE',  ( 0.000000000000000000, 0.000000000000000000, -1.000000000000000000 ) ) ;
#101875=DIRECTION ( 'NONE',  ( 0.000000000000000000, 1.000000000000000000, 0.000000000000000000 ) ) ;
#101876=DIRECTION ( 'NONE',  ( 0.000000000000000000, 0.000000000000000000, -1.000000000000000000 ) ) ;
#101912=CARTESIAN_POINT ( 'NONE',  ( -9.706334639731263536, 5.108299517166001280, 6.477055075394225092 ) ) ;
#101924=VERTEX_POINT ( 'NONE', #163726 ) ;
#101935=B_SPLINE_CURVE_WITH_KNOTS ( 'NONE', 3,
 ( #82297, #165693, #108752, #194194, #59926, #115934 ),
 .UNSPECIFIED., .F., .F.,
 ( 4, 2, 4 ),
 ( 0.000000000000000000, 0.0003844267940947825469, 0.0007688535881895650938 ),
 .UNSPECIFIED. ) ;
#101941=CARTESIAN_POINT ( 'NONE',  ( -9.333041836229964971, 15.44694763438214125, -7.472413793098273693 ) ) ;
#102004=DIRECTION ( 'NONE',  ( 0.000000000000000000, 0.000000000000000000, -1.000000000000000000 ) ) ;
#102012=VECTOR ( 'NONE', #172053, 1000.000000000000000 ) ;
#102037=VERTEX_POINT ( 'NONE', #33703 ) ;
#102048=CARTESIAN_POINT ( 'NONE',  ( -12.93621305287376089, 7.735084883283615653, -1.079074430401041118 ) ) ;
#102057=CIRCLE ( 'NONE', #198807, 11.92000000000000171 ) ;
#102074=CARTESIAN_POINT ( 'NONE',  ( 11.94980361723080264, 12.59761943414562957, -1.099999926404445771 ) ) ;
#102107=DIRECTION ( 'NONE',  ( 0.1510067114093955887, 0.000000000000000000, -0.9885327375000383388 ) ) ;
#102113=VECTOR ( 'NONE', #173403, 1000.000000000000000 ) ;
#102114=CARTESIAN_POINT ( 'NONE',  ( -11.32753564352527675, 6.357177643255160326, -3.964828284308058226 ) ) ;
#102160=CARTESIAN_POINT ( 'NONE',  ( 7.536566823016115357, 13.99512261572719929, -10.19722028184718532 ) ) ;
#102176=CARTESIAN_POINT ( 'NONE',  ( 11.86239285000045918, 13.88000000000000078, -1.812080536912753059 ) ) ;
#102192=CARTESIAN_POINT ( 'NONE',  ( 6.902720183911293717, 15.44694763437295570, -9.761920501353824164 ) ) ;
#102205=VERTEX_POINT ( 'NONE', #200451 ) ;
#102209=CARTESIAN_POINT ( 'NONE',  ( 7.979500612418553906, 15.27321092523385104, 8.904723856824006134 ) ) ;
#102210=CARTESIAN_POINT ( 'NONE',  ( -11.89835103415199313, 13.82893085832464131, 1.561208891256346876 ) ) ;
#102211=ORIENTED_EDGE ( 'NONE', *, *, #110606, .F. ) ;
#102259=CARTESIAN_POINT ( 'NONE',  ( -11.97185388258315086, 12.22000009279607546, -0.8311143155443164732 ) ) ;
#102261=ADVANCED_FACE ( 'NONE', ( #118224 ), #3311, .T. ) ;
#102284=FACE_OUTER_BOUND ( 'NONE', #26455, .T. ) ;
#102316=CARTESIAN_POINT ( 'NONE',  ( -0.008622056139523381901, 15.44694768828586540, 11.95585894197802013 ) ) ;
#102325=CARTESIAN_POINT ( 'NONE',  ( -1.499999999999946709, 7.750000000000000000, 15.75000000000000711 ) ) ;
#102330=UNCERTAINTY_MEASURE_WITH_UNIT (LENGTH_MEASURE( 1.000000000000000082E-05 ), #77369, 'distance_accuracy_value', 'NONE');
#102332=MECHANICAL_DESIGN_GEOMETRIC_PRESENTATION_REPRESENTATION('',(#8954),#12500);
#102376=( LENGTH_UNIT ( ) NAMED_UNIT ( * ) SI_UNIT ( .MILLI., .METRE. ) );
#102377=EDGE_CURVE ( 'NONE', #152468, #30835, #171171, .T. ) ;
#102386=PRESENTATION_STYLE_ASSIGNMENT (( #50446 ) ) ;
#102402=DIRECTION ( 'NONE',  ( -0.1510067114093955887, 0.000000000000000000, 0.9885327375000383388 ) ) ;
#102406=PRODUCT_CONTEXT ( 'NONE', #49107, 'mechanical' ) ;
#102436=CARTESIAN_POINT ( 'NONE',  ( -10.12885446735897510, 6.153639267710001803, -5.673676530672286944 ) ) ;
#102443=( GEOMETRIC_REPRESENTATION_CONTEXT ( 3 ) GLOBAL_UNCERTAINTY_ASSIGNED_CONTEXT ( ( #182863 ) ) GLOBAL_UNIT_ASSIGNED_CONTEXT ( ( #183635, #87207, #51518 ) ) REPRESENTATION_CONTEXT ( 'NONE', 'WORKASPACE' ) );
#102449=VERTEX_POINT ( 'NONE', #22761 ) ;
#102481=DIRECTION ( 'NONE',  ( 0.000000000000000000, 1.000000000000000000, 0.000000000000000000 ) ) ;
#102484=( GEOMETRIC_REPRESENTATION_CONTEXT ( 3 ) GLOBAL_UNCERTAINTY_ASSIGNED_CONTEXT ( ( #77125 ) ) GLOBAL_UNIT_ASSIGNED_CONTEXT ( ( #69234, #165699, #17288 ) ) REPRESENTATION_CONTEXT ( 'NONE', 'WORKASPACE' ) );
#102508=EDGE_LOOP ( 'NONE', ( #63315, #55490, #139621, #151607 ) ) ;
#102513=CARTESIAN_POINT ( 'NONE',  ( -10.87339650836132776, 5.131772588966429183, -5.487095527168452058 ) ) ;
#102536=EDGE_LOOP ( 'NONE', ( #75147, #111577, #146975, #81358 ) ) ;
#102542=CARTESIAN_POINT ( 'NONE',  ( -10.14891672641957499, 5.000029895416906456, -7.601366607803407227 ) ) ;
#102561=CARTESIAN_POINT ( 'NONE',  ( 11.76011352416511535, 6.974713285862789824, 2.433019384783116745 ) ) ;
#102565=ORIENTED_EDGE ( 'NONE', *, *, #179202, .F. ) ;
#102573=CARTESIAN_POINT ( 'NONE',  ( 10.16132735305258628, 13.50054059766859993, 7.251518808614104472 ) ) ;
#102580=B_SPLINE_CURVE_WITH_KNOTS ( 'NONE', 3,
 ( #203579, #9666, #173265, #157012, #73603, #189490 ),
 .UNSPECIFIED., .F., .F.,
 ( 4, 2, 4 ),
 ( 0.000000000000000000, 0.0003129201390360506364, 0.0006258402780721015980 ),
 .UNSPECIFIED. ) ;
#102587=CARTESIAN_POINT ( 'NONE',  ( -4.379492900960898716, 15.46945218216220219, -11.18131077117918792 ) ) ;
#102589=ORIENTED_EDGE ( 'NONE', *, *, #59134, .F. ) ;
#102591=EDGE_CURVE ( 'NONE', #198330, #702, #209495, .T. ) ;
#102613=ORIENTED_EDGE ( 'NONE', *, *, #120570, .F. ) ;
#102621=CARTESIAN_POINT ( 'NONE',  ( -9.367496997901325173, 14.48154074412966175, -7.499999999620646562 ) ) ;
#102632=CARTESIAN_POINT ( 'NONE',  ( 11.86687934130374522, 13.60951949616558565, -1.056332641424308827 ) ) ;
#102654=ORIENTED_EDGE ( 'NONE', *, *, #207872, .T. ) ;
#102666=COLOUR_RGB ( '', 0.09019608, 0.27058824, 0.51372549) ;
#102687=B_SPLINE_CURVE_WITH_KNOTS ( 'NONE', 3,
 ( #42672, #55685, #204036, #23163, #39438, #105532, #206195, #10130, #171566, #57823, #72988, #41602, #157479, #89279, #104452, #22082 ),
 .UNSPECIFIED., .F., .F.,
 ( 4, 2, 2, 2, 2, 2, 2, 4 ),
 ( 8.673617379884027768E-19, 0.001349084649940009107, 0.002698169299880017347, 0.004047253949820025370, 0.005396338599760033827, 0.006745423249700042284, 0.008094507899640049006, 0.01079267719952006592 ),
 .UNSPECIFIED. ) ;
#102693=ORIENTED_EDGE ( 'NONE', *, *, #139910, .F. ) ;
#102698=UNCERTAINTY_MEASURE_WITH_UNIT (LENGTH_MEASURE( 1.000000000000000082E-05 ), #111481, 'distance_accuracy_value', 'NONE');
#102711=EDGE_CURVE ( 'NONE', #96984, #73222, #92465, .T. ) ;
#102726=SURFACE_SIDE_STYLE ('',( #72333 ) ) ;
#102751=DIRECTION ( 'NONE',  ( -3.706092522800016599E-15, 0.000000000000000000, -1.000000000000000000 ) ) ;
#102759=CARTESIAN_POINT ( 'NONE',  ( 11.52888687719611305, 13.79423125104975689, 3.331331986263551315 ) ) ;
#102775=( LENGTH_UNIT ( ) NAMED_UNIT ( * ) SI_UNIT ( .MILLI., .METRE. ) );
#102789=CONICAL_SURFACE ( 'NONE', #120175, 10.75000000000000000, 0.5235987755983064762 ) ;
#102800=AXIS2_PLACEMENT_3D ( 'NONE', #170403, #21991, #201815 ) ;
#102836=CARTESIAN_POINT ( 'NONE',  ( -10.50000000000000000, 12.69999999999999929, -3.600000000000000977 ) ) ;
#102837=CARTESIAN_POINT ( 'NONE',  ( -10.37901820579008039, 4.889546506944066451, 5.358714317323078014 ) ) ;
#102845=CARTESIAN_POINT ( 'NONE',  ( -11.41381676900475917, 11.03041960022397561, 3.704697931490214646 ) ) ;
#102873=CIRCLE ( 'NONE', #43984, 0.07999999999999977962 ) ;
#102879=CARTESIAN_POINT ( 'NONE',  ( -15.75000000000000000, 10.89999999999998259, 1.399999999999998579 ) ) ;
#102910=ORIENTED_EDGE ( 'NONE', *, *, #24698, .T. ) ;
#102914=CARTESIAN_POINT ( 'NONE',  ( -11.81900460097218186, 13.75757134874138465, -1.592493057836596337 ) ) ;
#102944=DIRECTION ( 'NONE',  ( -0.000000000000000000, 1.000000000000000000, 0.000000000000000000 ) ) ;
#102945=DIRECTION ( 'NONE',  ( 0.000000000000000000, 0.000000000000000000, -1.000000000000000000 ) ) ;
#102980=CARTESIAN_POINT ( 'NONE',  ( -10.48284956170200921, 5.077895721165493370, 7.121295720048954614 ) ) ;
#103033=CARTESIAN_POINT ( 'NONE',  ( -10.36154070669560134, 3.772592418234324896, -6.054033915187476467 ) ) ;
#103048=EDGE_CURVE ( 'NONE', #80885, #44585, #92902, .T. ) ;
#103066=CARTESIAN_POINT ( 'NONE',  ( -7.790615780789408085, 15.44814080676280277, -9.079613476728765065 ) ) ;
#103069=CIRCLE ( 'NONE', #26964, 0.07999999999999998779 ) ;
#103092=ORIENTED_EDGE ( 'NONE', *, *, #136534, .T. ) ;
#103100=EDGE_LOOP ( 'NONE', ( #40524, #148476, #212992, #51251 ) ) ;
#103118=DIRECTION ( 'NONE',  ( 0.000000000000000000, 0.000000000000000000, 1.000000000000000000 ) ) ;
#103119=FILL_AREA_STYLE_COLOUR ( '', #188035 ) ;
#103130=CARTESIAN_POINT ( 'NONE',  ( 9.703911172298809618, 13.32558040432908619, 8.137536601084995880 ) ) ;
#103148=DIRECTION ( 'NONE',  ( 1.000000000000000000, -0.000000000000000000, -0.000000000000000000 ) ) ;
#103182=CARTESIAN_POINT ( 'NONE',  ( -10.33392256004288079, 4.765625372279607141, 5.445010993851796322 ) ) ;
#103222=EDGE_CURVE ( 'NONE', #210726, #58569, #54546, .T. ) ;
#103230=CARTESIAN_POINT ( 'NONE',  ( 9.681426354872444406, 13.43812210156014686, -8.165041025796163865 ) ) ;
#103263=CARTESIAN_POINT ( 'NONE',  ( 8.561438655473816439, 14.95580071018964041, -8.346266854202061936 ) ) ;
#103279=CARTESIAN_POINT ( 'NONE',  ( 8.559698219247815487, 14.95637777618389208, 8.348061575730120865 ) ) ;
#103284=LINE ( 'NONE', #68619, #30292 ) ;
#103305=CIRCLE ( 'NONE', #207039, 11.18000000000000149 ) ;
#103335=CARTESIAN_POINT ( 'NONE',  ( -10.94883623364795966, 5.391122956802682609, -4.806613302849912728 ) ) ;
#103343=LINE ( 'NONE', #165143, #46999 ) ;
#103346=DIRECTION ( 'NONE',  ( 0.000000000000000000, -0.000000000000000000, 1.000000000000000000 ) ) ;
#103350=B_SPLINE_CURVE_WITH_KNOTS ( 'NONE', 3,
 ( #77925, #127849, #177572, #30254, #95275, #161323, #96338, #13971, #32386, #100576, #167711, #82184, #98451, #163458, #151477, #19315 ),
 .UNSPECIFIED., .F., .F.,
 ( 4, 2, 2, 2, 2, 2, 2, 4 ),
 ( 2.453269466693426431E-18, 8.859500147854104581E-05, 0.0001771900029570796522, 0.0003543800059141551844, 0.0007087600118283104772, 0.001063140017742465445, 0.001240330020699543633, 0.001417520023656621822 ),
 .UNSPECIFIED. ) ;
#103362=DIRECTION ( 'NONE',  ( 0.000000000000000000, 0.000000000000000000, 1.000000000000000000 ) ) ;
#103379=ORIENTED_EDGE ( 'NONE', *, *, #191821, .T. ) ;
#103387=STYLED_ITEM ( 'NONE', ( #168756 ), #21012 ) ;
#103391=CARTESIAN_POINT ( 'NONE',  ( -0.03829719982252339366, 15.47641828198856295, 11.98867496343628680 ) ) ;
#103399=CARTESIAN_POINT ( 'NONE',  ( -11.15698333951949195, 7.317141096829810287, 4.424938813521728243 ) ) ;
#103400=DIRECTION ( 'NONE',  ( 0.3162277660168376636, 0.9486832980505138790, 0.000000000000000000 ) ) ;
#103413=B_SPLINE_CURVE_WITH_KNOTS ( 'NONE', 3,
 ( #132727, #98088, #183564, #68729, #147894, #48274 ),
 .UNSPECIFIED., .F., .F.,
 ( 4, 2, 4 ),
 ( 0.001916662113439827377, 0.002237152494173779219, 0.002557642874907731494 ),
 .UNSPECIFIED. ) ;
#103430=AXIS2_PLACEMENT_3D ( 'NONE', #144346, #210346, #178949 ) ;
#103438=CARTESIAN_POINT ( 'NONE',  ( -11.04536101718726293, 0.000000000000000000, -1.100000000000002087 ) ) ;
#103451=CARTESIAN_POINT ( 'NONE',  ( 0.000000000000000000, 18.91999999999999815, 0.000000000000000000 ) ) ;
#103461=PLANE ( 'NONE',  #195827 ) ;
#103475=DIRECTION ( 'NONE',  ( 0.9885327375000381167, 0.000000000000000000, 0.1510067114093955609 ) ) ;
#103484=UNCERTAINTY_MEASURE_WITH_UNIT (LENGTH_MEASURE( 1.000000000000000082E-05 ), #172642, 'distance_accuracy_value', 'NONE');
#103513=CARTESIAN_POINT ( 'NONE',  ( -11.69243366784185945, 8.407932920124673970, 1.097391832464843286 ) ) ;
#103520=CARTESIAN_POINT ( 'NONE',  ( -1.499999999999963141, 7.750000000000000000, -10.99818166789402518 ) ) ;
#103532=CARTESIAN_POINT ( 'NONE',  ( -9.963041989461812520, 4.512757371444226173, 6.615979002877482529 ) ) ;
#103541=VERTEX_POINT ( 'NONE', #40945 ) ;
#103543=( LENGTH_UNIT ( ) NAMED_UNIT ( * ) SI_UNIT ( .MILLI., .METRE. ) );
#103553=SURFACE_STYLE_FILL_AREA ( #37475 ) ;
#103606=EDGE_LOOP ( 'NONE', ( #178251, #152903, #9508, #8555 ) ) ;
#103616=ADVANCED_FACE ( 'NONE', ( #39869 ), #141025, .T. ) ;
#103621=CARTESIAN_POINT ( 'NONE',  ( -9.979907920417568690, 3.147823346236176878, -6.101210848797135711 ) ) ;
#103622=SURFACE_STYLE_USAGE ( .BOTH. , #202141 ) ;
#103632=CARTESIAN_POINT ( 'NONE',  ( 11.07790593930098311, 9.799999999999998934, -0.7000000000000009548 ) ) ;
#103638=CARTESIAN_POINT ( 'NONE',  ( 11.95123587697795564, 6.644955863035443500, -0.4920656033008508623 ) ) ;
#103640=ORIENTED_EDGE ( 'NONE', *, *, #203982, .F. ) ;
#103665=CARTESIAN_POINT ( 'NONE',  ( -5.600700517108988308, 15.46906632287834071, -10.62221823295361567 ) ) ;
#103666=EDGE_LOOP ( 'NONE', ( #173809, #205775, #75152, #130166 ) ) ;
#103734=CARTESIAN_POINT ( 'NONE',  ( -15.75000000000000000, 10.19999999999999929, 0.6999999999999992895 ) ) ;
#103751=EDGE_CURVE ( 'NONE', #171829, #18446, #170771, .T. ) ;
#103777=CARTESIAN_POINT ( 'NONE',  ( 9.809231760985728243, 10.20995912723616428, -6.918706496639274839 ) ) ;
#103791=EDGE_CURVE ( 'NONE', #195702, #115034, #185942, .T. ) ;
#103792=PLANE ( 'NONE',  #120030 ) ;
#103800=SURFACE_STYLE_USAGE ( .BOTH. , #102726 ) ;
#103804=CARTESIAN_POINT ( 'NONE',  ( 11.96215121607992771, 13.82833553780823976, 0.9565349792967584586 ) ) ;
#103821=SURFACE_SIDE_STYLE ('',( #101675 ) ) ;
#103822=DIRECTION ( 'NONE',  ( -0.000000000000000000, -1.000000000000000000, -0.000000000000000000 ) ) ;
#103823=SURFACE_STYLE_FILL_AREA ( #137397 ) ;
#103868=CARTESIAN_POINT ( 'NONE',  ( -9.367496997601184816, 15.42330868760440410, -7.413898975931886959 ) ) ;
#103892=CARTESIAN_POINT ( 'NONE',  ( -11.80235830595197655, 9.799999999999982947, 1.696088231482817399 ) ) ;
#103900=CARTESIAN_POINT ( 'NONE',  ( -15.75000000000000000, 13.79999999999998295, 1.799999999999999600 ) ) ;
#103908=CARTESIAN_POINT ( 'NONE',  ( 9.710969956560674632, 13.29837910982962690, -8.127984515541683663 ) ) ;
#103909=CARTESIAN_POINT ( 'NONE',  ( -9.348561386651960348, 5.000000000000002665, 7.001914024036568485 ) ) ;
#103919=CARTESIAN_POINT ( 'NONE',  ( -10.62873463776380056, 11.29999999999998117, 3.199999999999997957 ) ) ;
#103942=CARTESIAN_POINT ( 'NONE',  ( 10.95308175811721085, 11.29999999999998117, 1.799999999999999600 ) ) ;
#103957=ORIENTED_EDGE ( 'NONE', *, *, #80728, .F. ) ;
#103959=DIRECTION ( 'NONE',  ( -3.491481338843133355E-15, 0.000000000000000000, -1.000000000000000000 ) ) ;
#103981=VERTEX_POINT ( 'NONE', #100099 ) ;
#103987=EDGE_LOOP ( 'NONE', ( #137822, #88801, #38896, #45736, #168439, #81403, #46944, #188037 ) ) ;
#104006=CARTESIAN_POINT ( 'NONE',  ( -9.367496997397941172, 15.46908218389366851, 7.500000000249372079 ) ) ;
#104027=CIRCLE ( 'NONE', #83280, 12.00000000000000178 ) ;
#104042=ADVANCED_FACE ( 'NONE', ( #152056 ), #143509, .T. ) ;
#104053=CARTESIAN_POINT ( 'NONE',  ( -11.55001508359621987, 4.031797291955615314, 5.408777164504234847 ) ) ;
#104067=CARTESIAN_POINT ( 'NONE',  ( -15.75000000000000000, 12.69999999999999929, -3.200000000000001510 ) ) ;
#104074=CARTESIAN_POINT ( 'NONE',  ( 1.734723475976807094E-15, 15.42691958146951414, 11.91973154060106665 ) ) ;
#104083=CARTESIAN_POINT ( 'NONE',  ( -1.863116269212363063, 15.51999112189398033, 11.88797926174050268 ) ) ;
#104103=CARTESIAN_POINT ( 'NONE',  ( -10.47216923660538335, 4.011714437494937613, -5.771917547288382799 ) ) ;
#104108=CARTESIAN_POINT ( 'NONE',  ( 11.91826848330682331, 12.59270354043007067, 1.400000080589832052 ) ) ;
#104111=EDGE_CURVE ( 'NONE', #37563, #62806, #193761, .T. ) ;
#104113=DIRECTION ( 'NONE',  ( -0.000000000000000000, 1.000000000000000000, 9.023263958591317418E-17 ) ) ;
#104122=AXIS2_PLACEMENT_3D ( 'NONE', #11814, #32347, #28078 ) ;
#104148=ADVANCED_FACE ( 'NONE', ( #37228 ), #17545, .T. ) ;
#104153=FILL_AREA_STYLE ('',( #186444 ) ) ;
#104188=( NAMED_UNIT ( * ) PLANE_ANGLE_UNIT ( ) SI_UNIT ( $, .RADIAN. ) );
#104189=CARTESIAN_POINT ( 'NONE',  ( -11.01578653029999266, 5.045029590669321884, -4.264301349201883085 ) ) ;
#104207=CARTESIAN_POINT ( 'NONE',  ( -15.75000000000000000, 12.69999999999999929, 1.099999999999996758 ) ) ;
#104211=CARTESIAN_POINT ( 'NONE',  ( -10.56513397747884397, 13.75900096514340198, 3.405015282931166620 ) ) ;
#104214=CARTESIAN_POINT ( 'NONE',  ( 11.97929049433705373, 13.88000000000000078, -0.7046979865771834106 ) ) ;
#104215=COLOUR_RGB ( '', 0.40784314, 0.44705882, 0.49803922) ;
#104242=FILL_AREA_STYLE ('',( #53346 ) ) ;
#104301=CARTESIAN_POINT ( 'NONE',  ( 7.577342237528466029, 14.99429123645997919, -10.16790800466224987 ) ) ;
#104305=B_SPLINE_CURVE_WITH_KNOTS ( 'NONE', 3,
 ( #9166, #7002, #141353, #124082, #155418, #105633 ),
 .UNSPECIFIED., .F., .F.,
 ( 4, 2, 4 ),
 ( 0.000000000000000000, 0.5000000000000000000, 1.000000000000000000 ),
 .UNSPECIFIED. ) ;
#104319=EDGE_LOOP ( 'NONE', ( #140715, #95601, #130875, #200412 ) ) ;
#104333=EDGE_CURVE ( 'NONE', #208480, #124513, #26858, .T. ) ;
#104348=EDGE_LOOP ( 'NONE', ( #169039, #182001, #132859, #54000, #4490, #78594 ) ) ;
#104353=CARTESIAN_POINT ( 'NONE',  ( 1.734723475976807094E-15, 14.57308041853048231, 11.91973154060107376 ) ) ;
#104354=CARTESIAN_POINT ( 'NONE',  ( -11.92046840572485777, 13.65252124794268873, 1.382231356234940867 ) ) ;
#104417=DIRECTION ( 'NONE',  ( -0.1700204568168937336, 0.9655305911742121383, 0.1970881066187179509 ) ) ;
#104418=CARTESIAN_POINT ( 'NONE',  ( -11.33772463945036968, 10.90000000000000036, -3.600000000000000977 ) ) ;
#104438=ORIENTED_EDGE ( 'NONE', *, *, #205622, .F. ) ;
#104452=CARTESIAN_POINT ( 'NONE',  ( -0.8999481596081082557, 14.48154075026957877, -12.00000000000000178 ) ) ;
#104475=CARTESIAN_POINT ( 'NONE',  ( -11.56045418304177197, 8.213790699071104484, -3.228785083172883486 ) ) ;
#104483=CIRCLE ( 'NONE', #159831, 12.00000000000000178 ) ;
#104508=AXIS2_PLACEMENT_3D ( 'NONE', #22994, #9964, #88024 ) ;
#104528=SURFACE_STYLE_USAGE ( .BOTH. , #4836 ) ;
#104538=CARTESIAN_POINT ( 'NONE',  ( -10.98549472050129694, 13.75729797278727773, -1.592011381755360722 ) ) ;
#104546=CARTESIAN_POINT ( 'NONE',  ( 7.879630799735125812, 14.91438228929072274, -9.066625182108625225 ) ) ;
#104554=CARTESIAN_POINT ( 'NONE',  ( 10.11573063517565707, 13.81601979175187545, 7.347423794093835170 ) ) ;
#104588=CARTESIAN_POINT ( 'NONE',  ( -10.60630082101195804, 5.715768461961713953, -4.896526734066639186 ) ) ;
#104616=ORIENTED_EDGE ( 'NONE', *, *, #3410, .T. ) ;
#104628=SURFACE_SIDE_STYLE ('',( #136060 ) ) ;
#104629=CARTESIAN_POINT ( 'NONE',  ( 1.500000000000035971, 7.750000000000000000, 10.64483442802187696 ) ) ;
#104645=DIRECTION ( 'NONE',  ( -0.05872483221476467591, -7.952201780260630618E-17, 0.9982742078614211811 ) ) ;
#104663=CARTESIAN_POINT ( 'NONE',  ( 11.86145016429273191, 13.40000000000000036, 1.099999999999996758 ) ) ;
#104674=STYLED_ITEM ( 'NONE', ( #25945 ), #175851 ) ;
#104694=CARTESIAN_POINT ( 'NONE',  ( -10.32649671959996596, 5.020010808682577874, -7.354824260697566451 ) ) ;
#104704=CARTESIAN_POINT ( 'NONE',  ( -10.60630588279735242, 5.715763139788331948, 4.896273837757428637 ) ) ;
#104709=ORIENTED_EDGE ( 'NONE', *, *, #93908, .T. ) ;
#104711=CARTESIAN_POINT ( 'NONE',  ( 11.05144304286076640, 8.019042783312965383, 4.564752377278145978 ) ) ;
#104714=ORIENTED_EDGE ( 'NONE', *, *, #77470, .T. ) ;
#104732=AXIS2_PLACEMENT_3D ( 'NONE', #49252, #165120, #16712 ) ;
#104736=CARTESIAN_POINT ( 'NONE',  ( -3.531151798259720476, 15.47001910837518857, -11.47749989083732203 ) ) ;
#104749=SURFACE_STYLE_USAGE ( .BOTH. , #188106 ) ;
#104784=CARTESIAN_POINT ( 'NONE',  ( -10.28140399934106242, 4.005782094233665269, -7.421933058660648008 ) ) ;
#104800=STYLED_ITEM ( 'NONE', ( #207847 ), #111664 ) ;
#104810=( NAMED_UNIT ( * ) SI_UNIT ( $, .STERADIAN. ) SOLID_ANGLE_UNIT ( ) );
#104881=CARTESIAN_POINT ( 'NONE',  ( 11.06299035296667732, 13.75683704376094774, -0.9087041361035911313 ) ) ;
#104882=DIRECTION ( 'NONE',  ( -0.000000000000000000, -1.000000000000000000, -0.000000000000000000 ) ) ;
#104889=( GEOMETRIC_REPRESENTATION_CONTEXT ( 3 ) GLOBAL_UNCERTAINTY_ASSIGNED_CONTEXT ( ( #160505 ) ) GLOBAL_UNIT_ASSIGNED_CONTEXT ( ( #102376, #55761, #138097 ) ) REPRESENTATION_CONTEXT ( 'NONE', 'WORKASPACE' ) );
#104891=CARTESIAN_POINT ( 'NONE',  ( 11.92619526913699879, 12.69999999999999929, -1.328859060402686199 ) ) ;
#104900=DIRECTION ( 'NONE',  ( -0.000000000000000000, -1.000000000000000000, -0.000000000000000000 ) ) ;
#104947=VERTEX_POINT ( 'NONE', #84334 ) ;
#104967=AXIS2_PLACEMENT_3D ( 'NONE', #20590, #151694, #50984 ) ;
#104985=CARTESIAN_POINT ( 'NONE',  ( -9.748179543381699119, 3.057003318903428912, 6.445181705109019887 ) ) ;
#105023=FILL_AREA_STYLE ('',( #73563 ) ) ;
#105033=FILL_AREA_STYLE ('',( #56269 ) ) ;
#105037=CIRCLE ( 'NONE', #80908, 0.07999999999999946043 ) ;
#105052=ADVANCED_FACE ( 'NONE', ( #153614 ), #206612, .F. ) ;
#105059=VERTEX_POINT ( 'NONE', #9487 ) ;
#105065=CARTESIAN_POINT ( 'NONE',  ( 1.734723475976807094E-15, 14.99962766111844736, 11.68000013863625774 ) ) ;
#105095=CARTESIAN_POINT ( 'NONE',  ( 11.33772463945036790, 13.40000000000000036, -3.680000000000002824 ) ) ;
#105097=CARTESIAN_POINT ( 'NONE',  ( 9.768581443174442214, 11.88588759030453268, -6.891829356553425434 ) ) ;
#105102=DIRECTION ( 'NONE',  ( 8.881784197001252323E-15, 0.000000000000000000, -1.000000000000000000 ) ) ;
#105132=CARTESIAN_POINT ( 'NONE',  ( -10.76112648294250462, 4.189587671054875173, 6.709456861673908534 ) ) ;
#105147=CYLINDRICAL_SURFACE ( 'NONE', #24621, 0.3999999999999997446 ) ;
#105167=ADVANCED_FACE ( 'NONE', ( #69244 ), #14998, .T. ) ;
#105206=ORIENTED_EDGE ( 'NONE', *, *, #168035, .F. ) ;
#105235=( LENGTH_UNIT ( ) NAMED_UNIT ( * ) SI_UNIT ( .MILLI., .METRE. ) );
#105266=STYLED_ITEM ( 'NONE', ( #98421 ), #116367 ) ;
#105268=CARTESIAN_POINT ( 'NONE',  ( -10.71026998871754721, 6.055660674263378951, 4.667787751035539223 ) ) ;
#105295=ORIENTED_EDGE ( 'NONE', *, *, #123377, .F. ) ;
#105297=CARTESIAN_POINT ( 'NONE',  ( 11.33772463945037146, 10.89999999999998259, 3.599999999999999201 ) ) ;
#105302=CARTESIAN_POINT ( 'NONE',  ( -11.94105721237523099, 12.69999999999999929, -1.187919463087249827 ) ) ;
#105315=CARTESIAN_POINT ( 'NONE',  ( 11.92619526913700057, 13.52781666661241466, 1.328859060402684644 ) ) ;
#105335=CARTESIAN_POINT ( 'NONE',  ( -1.386567914617467867, 8.090296256147714971, -10.72428812184711511 ) ) ;
#105339=CARTESIAN_POINT ( 'NONE',  ( 11.33772463945037146, 10.09088423488572062, 3.599999999999998757 ) ) ;
#105382=CARTESIAN_POINT ( 'NONE',  ( 8.739888343381572611, 14.93516617432513982, 8.229140924179734640 ) ) ;
#105394=AXIS2_PLACEMENT_3D ( 'NONE', #31500, #198227, #130138 ) ;
#105424=( GEOMETRIC_REPRESENTATION_CONTEXT ( 3 ) GLOBAL_UNCERTAINTY_ASSIGNED_CONTEXT ( ( #167474 ) ) GLOBAL_UNIT_ASSIGNED_CONTEXT ( ( #30665, #62088, #129314 ) ) REPRESENTATION_CONTEXT ( 'NONE', 'WORKASPACE' ) );
#105444=CARTESIAN_POINT ( 'NONE',  ( 1.469576158976824144E-15, 15.51887838114830132, 12.00000000000000178 ) ) ;
#105449=CARTESIAN_POINT ( 'NONE',  ( -3.543819111236696795, 14.48034520802695724, -11.47346693889574176 ) ) ;
#105457=VERTEX_POINT ( 'NONE', #9596 ) ;
#105485=DIRECTION ( 'NONE',  ( 1.000000000000000000, -0.000000000000000000, -0.000000000000000000 ) ) ;
#105504=CARTESIAN_POINT ( 'NONE',  ( -11.55950211276791073, 11.29999999999999893, -3.221476510067115662 ) ) ;
#105509=ORIENTED_EDGE ( 'NONE', *, *, #108367, .F. ) ;
#105532=CARTESIAN_POINT ( 'NONE',  ( -7.120058540175079997, 14.48019278289790002, -9.669703550014270732 ) ) ;
#105541=AXIS2_PLACEMENT_3D ( 'NONE', #204673, #142941, #90973 ) ;
#105543=VERTEX_POINT ( 'NONE', #103919 ) ;
#105549=CARTESIAN_POINT ( 'NONE',  ( 11.84668730067608600, 19.00000000000000000, 1.319999999999998286 ) ) ;
#105556=SURFACE_SIDE_STYLE ('',( #57844 ) ) ;
#105569=COLOUR_RGB ( '', 0.31764706, 0.68627451, 0.89019608) ;
#105592=ADVANCED_FACE ( 'NONE', ( #30117 ), #47454, .F. ) ;
#105612=SURFACE_STYLE_FILL_AREA ( #21093 ) ;
#105633=CARTESIAN_POINT ( 'NONE',  ( 6.928203230275520319, 15.00000000000000000, 9.797958971132713302 ) ) ;
#105640=CARTESIAN_POINT ( 'NONE',  ( 7.910363579994360350, 15.96602505221457058, 9.911917230698591652 ) ) ;
#105661=CARTESIAN_POINT ( 'NONE',  ( 11.89204169242350595, 9.799999999999998934, 0.8046421800351223341 ) ) ;
#105674=CARTESIAN_POINT ( 'NONE',  ( -11.36822525729066413, 5.406166865499119289, 5.610767994321700591 ) ) ;
#105683=CARTESIAN_POINT ( 'NONE',  ( -11.07131503167114772, 9.799999999999998934, 0.8043049353970799231 ) ) ;
#105691=CARTESIAN_POINT ( 'NONE',  ( -15.75000000000000000, 12.69999999999999929, 1.099999999999996758 ) ) ;
#105694=DIRECTION ( 'NONE',  ( 1.509903313490213211E-14, 0.000000000000000000, -1.000000000000000000 ) ) ;
#105705=CARTESIAN_POINT ( 'NONE',  ( 9.423147110355582612, 13.09353312253862178, 7.356331950284607402 ) ) ;
#105724=EDGE_CURVE ( 'NONE', #129573, #134499, #69440, .T. ) ;
#105732=CIRCLE ( 'NONE', #140204, 0.08000000000000040412 ) ;
#105755=( BOUNDED_SURFACE ( )  B_SPLINE_SURFACE ( 3, 2, ( 
 ( #110938, #145555, #14417 ),
 ( #210493, #77303, #13364 ),
 ( #194251, #78366, #209409 ),
 ( #93582, #159627, #96789 ),
 ( #130407, #129352, #80506 ),
 ( #146603, #95719, #162839 ) ),
 .UNSPECIFIED., .F., .F., .T. ) 
 B_SPLINE_SURFACE_WITH_KNOTS ( ( 4, 2, 4 ),
 ( 3, 3 ),
 ( 0.000000000000000000, 0.0003754691837024766443, 0.0007509383674049532886 ),
 ( 0.000000000000000000, 1.000000000000000000 ),
 .UNSPECIFIED. ) 
 GEOMETRIC_REPRESENTATION_ITEM ( )  RATIONAL_B_SPLINE_SURFACE ( (
 ( 1.000000000000000000, 0.6711954675835484219, 1.000000000000000000),
 ( 1.000000000000000000, 0.6709646295267019944, 1.000000000000000000),
 ( 1.000000000000000000, 0.6771840716659748294, 1.000000000000000000),
 ( 1.000000000000000000, 0.6927481755866885527, 1.000000000000000000),
 ( 1.000000000000000000, 0.7017972101310294697, 1.000000000000000000),
 ( 1.000000000000000000, 0.7071067811865475727, 1.000000000000000000) ) ) 
 REPRESENTATION_ITEM ( '' )  SURFACE ( )  );
#105783=ORIENTED_EDGE ( 'NONE', *, *, #203843, .T. ) ;
#105794=LINE ( 'NONE', #155576, #212590 ) ;
#105801=CARTESIAN_POINT ( 'NONE',  ( -9.986127180934126102, 5.615481227002261377, 5.966285604742011195 ) ) ;
#105818=CARTESIAN_POINT ( 'NONE',  ( 0.000000000000000000, 13.88000000000000078, 0.000000000000000000 ) ) ;
#105821=LINE ( 'NONE', #192342, #106703 ) ;
#105829=EDGE_CURVE ( 'NONE', #117790, #90065, #2914, .T. ) ;
#105867=ORIENTED_EDGE ( 'NONE', *, *, #6305, .T. ) ;
#105877=CARTESIAN_POINT ( 'NONE',  ( -9.470156251935129887, 4.005132839944305800, -6.837168546664702085 ) ) ;
#105948=CARTESIAN_POINT ( 'NONE',  ( 11.53060642766661736, 7.261346649532379516, 3.356656312893389948 ) ) ;
#105951=COLOUR_RGB ( '', 0.40784314, 0.44705882, 0.49803922) ;
#105986=CARTESIAN_POINT ( 'NONE',  ( 11.86145016429273191, 10.90000000000000036, 1.099999999999996980 ) ) ;
#106003=DIRECTION ( 'NONE',  ( 0.000000000000000000, 0.000000000000000000, -1.000000000000000000 ) ) ;
#106004=CARTESIAN_POINT ( 'NONE',  ( 11.35610322553117157, 12.48578371070824744, -3.553412924323506861 ) ) ;
#106034=CARTESIAN_POINT ( 'NONE',  ( -1.423205080756925867, 7.980384757729337863, -10.65537363484301636 ) ) ;
#106044=DIRECTION ( 'NONE',  ( 0.6250000000000000000, 1.408756634010579545E-16, -0.7806247497997997886 ) ) ;
#106055=CARTESIAN_POINT ( 'NONE',  ( 0.000000000000000000, 18.91999999999999815, 0.000000000000000000 ) ) ;
#106056=AXIS2_PLACEMENT_3D ( 'NONE', #205164, #56806, #115229 ) ;
#106084=CARTESIAN_POINT ( 'NONE',  ( -11.88237264505823987, 13.75677038468317015, 0.9087825512662228711 ) ) ;
#106085=CARTESIAN_POINT ( 'NONE',  ( -10.89402507593495351, 4.580915115640823210, 4.512369680550198936 ) ) ;
#106089=AXIS2_PLACEMENT_3D ( 'NONE', #26095, #120489, #88994 ) ;
#106119=ORIENTED_EDGE ( 'NONE', *, *, #142360, .T. ) ;
#106150=SURFACE_SIDE_STYLE ('',( #209967 ) ) ;
#106152=CARTESIAN_POINT ( 'NONE',  ( 0.000000000000000000, 3.481548657788669843, 0.000000000000000000 ) ) ;
#106161=CARTESIAN_POINT ( 'NONE',  ( 1.474529836884923328E-15, 14.99975178945622822, 11.68000004620062526 ) ) ;
#106182=CARTESIAN_POINT ( 'NONE',  ( -3.069665630396485323, 15.47024000507179231, 11.60952187717502326 ) ) ;
#106195=DIRECTION ( 'NONE',  ( 0.000000000000000000, 0.000000000000000000, 1.000000000000000000 ) ) ;
#106196=CARTESIAN_POINT ( 'NONE',  ( -10.95308175811721085, 9.799999999999982947, 1.799999999999999600 ) ) ;
#106205=COLOUR_RGB ( '', 0.72549020, 0.75294118, 0.79215686) ;
#106228=CARTESIAN_POINT ( 'NONE',  ( -9.348561386651960348, 2.999999999999999112, 7.001914024036568485 ) ) ;
#106229=VERTEX_POINT ( 'NONE', #101512 ) ;
#106237=ORIENTED_EDGE ( 'NONE', *, *, #207506, .F. ) ;
#106243=( LENGTH_UNIT ( ) NAMED_UNIT ( * ) SI_UNIT ( .MILLI., .METRE. ) );
#106245=( GEOMETRIC_REPRESENTATION_CONTEXT ( 3 ) GLOBAL_UNCERTAINTY_ASSIGNED_CONTEXT ( ( #27305 ) ) GLOBAL_UNIT_ASSIGNED_CONTEXT ( ( #197918, #168632, #172929 ) ) REPRESENTATION_CONTEXT ( 'NONE', 'WORKASPACE' ) );
#106258=( GEOMETRIC_REPRESENTATION_CONTEXT ( 3 ) GLOBAL_UNCERTAINTY_ASSIGNED_CONTEXT ( ( #83518 ) ) GLOBAL_UNIT_ASSIGNED_CONTEXT ( ( #149343, #66990, #199127 ) ) REPRESENTATION_CONTEXT ( 'NONE', 'WORKASPACE' ) );
#106271=STYLED_ITEM ( 'NONE', ( #50962 ), #145317 ) ;
#106272=CARTESIAN_POINT ( 'NONE',  ( 11.97178994924802353, 13.87999993797205356, 0.8322011300497295094 ) ) ;
#106281=CARTESIAN_POINT ( 'NONE',  ( -8.795148599269996481, 14.53091781150858885, 8.214862920035907123 ) ) ;
#106341=ORIENTED_EDGE ( 'NONE', *, *, #136534, .F. ) ;
#106347=CARTESIAN_POINT ( 'NONE',  ( 11.35573736746281348, 9.987295855867177607, -3.554362808847921773 ) ) ;
#106360=ADVANCED_FACE ( 'NONE', ( #9470 ), #40928, .F. ) ;
#106366=CARTESIAN_POINT ( 'NONE',  ( -10.99931038725301846, 6.873658557531565627, -3.960823121322395224 ) ) ;
#106367=CIRCLE ( 'NONE', #109794, 12.00000000000000178 ) ;
#106369=CARTESIAN_POINT ( 'NONE',  ( 7.947120472790364154, 14.95225098152464582, 9.881210053433072460 ) ) ;
#106379=DIRECTION ( 'NONE',  ( 0.6249999999996046496, -1.033735393388932873E-14, 0.7806247498001164242 ) ) ;
#106397=AXIS2_PLACEMENT_3D ( 'NONE', #152792, #55296, #68317 ) ;
#106403=EDGE_CURVE ( 'NONE', #79124, #181635, #92759, .T. ) ;
#106405=AXIS2_PLACEMENT_3D ( 'NONE', #7675, #140935, #11948 ) ;
#106422=CARTESIAN_POINT ( 'NONE',  ( 11.55950211276791251, 12.21999999999998288, 3.221476510067110777 ) ) ;
#106425=ORIENTED_EDGE ( 'NONE', *, *, #138826, .F. ) ;
#106455=DIRECTION ( 'NONE',  ( 0.000000000000000000, -1.000000000000000000, -0.000000000000000000 ) ) ;
#106475=CARTESIAN_POINT ( 'NONE',  ( 8.279175489589290393, 15.22702719263014615, 8.688122134494948412 ) ) ;
#106480=DIRECTION ( 'NONE',  ( 0.000000000000000000, 7.228014483236694583E-17, -1.000000000000000000 ) ) ;
#106486=ORIENTED_EDGE ( 'NONE', *, *, #137412, .T. ) ;
#106521=CARTESIAN_POINT ( 'NONE',  ( -10.41437568897905486, 3.950072978995299522, 5.872581675051923966 ) ) ;
#106535=CARTESIAN_POINT ( 'NONE',  ( 11.86145016429273191, 10.19999999999999929, 1.099999999999996758 ) ) ;
#106540=CARTESIAN_POINT ( 'NONE',  ( -1.797304807700269569, 14.48004927660067764, -11.89862588611542726 ) ) ;
#106547=VERTEX_POINT ( 'NONE', #130761 ) ;
#106571=( BOUNDED_SURFACE ( )  B_SPLINE_SURFACE ( 3, 3, ( 
 ( #185995, #120019, #203304, #54951, #121104, #33354, #139418, #92811, #39772, #23499, #205453, #123251, #6171, #105877, #157801, #7238 ),
 ( #106961, #10452, #204364, #73315, #125365, #88531, #56020, #72239, #24565, #171901, #141581, #8325, #191328, #57086, #189215, #138347 ),
 ( #206520, #109107, #142636, #140509, #42994, #75469, #76525, #91748, #207589, #154592, #188140, #9397, #158854, #175122, #59208, #122174 ),
 ( #26708, #89605, #40855, #155656, #172986, #74409, #38704, #208645, #90671, #60277, #156734, #187071, #58152, #104784, #124311, #190270 ),
 ( #41927, #108038, #25636, #174064, #170830, #22421, #94941, #11524, #2440, #18706, #209709, #159919, #97075, #179380, #12581, #126434 ),
 ( #79725, #145841, #133584, #128576, #78653, #46187, #93881, #110172, #129638, #63484, #211846, #67439, #150877, #117355, #34957, #61353 ),
 ( #29927, #1378, #176183, #160989, #31000, #84789, #195625, #199588, #47260, #111237, #27782, #177240, #144781, #62412, #192397, #166044 ) ),
 .UNSPECIFIED., .T., .F., .F. ) 
 B_SPLINE_SURFACE_WITH_KNOTS ( ( 4, 3, 4 ),
 ( 4, 2, 2, 2, 2, 2, 2, 4 ),
 ( 0.000000000000000000, 0.5000000000000000000, 1.000000000000000000 ),
 ( 0.6095821870314059865, 0.6120980958896804491, 0.6146140047479549118, 0.6196458224645037260, 0.6297094578976014656, 0.6397880689092279027, 0.6448273744150412323, 0.6498666799208544509 ),
 .UNSPECIFIED. ) 
 GEOMETRIC_REPRESENTATION_ITEM ( )  RATIONAL_B_SPLINE_SURFACE ( (
 ( 1.000000000000000000, 1.000000000000000000, 1.000000000000000000, 1.000000000000000000, 1.000000000000000000, 1.000000000000000000, 1.000000000000000000, 1.000000000000000000, 1.000000000000000000, 1.000000000000000000, 1.000000000000000000, 1.000000000000000000, 1.000000000000000000, 1.000000000000000000, 1.000000000000000000, 1.000000000000000000),
 ( 0.3333333333333333703, 0.3333333333333333703, 0.3333333333333333703, 0.3333333333333333703, 0.3333333333333333703, 0.3333333333333333703, 0.3333333333333333703, 0.3333333333333333703, 0.3333333333333333703, 0.3333333333333333703, 0.3333333333333333703, 0.3333333333333333703, 0.3333333333333333703, 0.3333333333333333703, 0.3333333333333333703, 0.3333333333333333703),
 ( 0.3333333333333333703, 0.3333333333333333703, 0.3333333333333333703, 0.3333333333333333703, 0.3333333333333333703, 0.3333333333333333703, 0.3333333333333333703, 0.3333333333333333703, 0.3333333333333333703, 0.3333333333333333703, 0.3333333333333333703, 0.3333333333333333703, 0.3333333333333333703, 0.3333333333333333703, 0.3333333333333333703, 0.3333333333333333703),
 ( 1.000000000000000000, 1.000000000000000000, 1.000000000000000000, 1.000000000000000000, 1.000000000000000000, 1.000000000000000000, 1.000000000000000000, 1.000000000000000000, 1.000000000000000000, 1.000000000000000000, 1.000000000000000000, 1.000000000000000000, 1.000000000000000000, 1.000000000000000000, 1.000000000000000000, 1.000000000000000000),
 ( 0.3333333333333333703, 0.3333333333333333703, 0.3333333333333333703, 0.3333333333333333703, 0.3333333333333333703, 0.3333333333333333703, 0.3333333333333333703, 0.3333333333333333703, 0.3333333333333333703, 0.3333333333333333703, 0.3333333333333333703, 0.3333333333333333703, 0.3333333333333333703, 0.3333333333333333703, 0.3333333333333333703, 0.3333333333333333703),
 ( 0.3333333333333333703, 0.3333333333333333703, 0.3333333333333333703, 0.3333333333333333703, 0.3333333333333333703, 0.3333333333333333703, 0.3333333333333333703, 0.3333333333333333703, 0.3333333333333333703, 0.3333333333333333703, 0.3333333333333333703, 0.3333333333333333703, 0.3333333333333333703, 0.3333333333333333703, 0.3333333333333333703, 0.3333333333333333703),
 ( 1.000000000000000000, 1.000000000000000000, 1.000000000000000000, 1.000000000000000000, 1.000000000000000000, 1.000000000000000000, 1.000000000000000000, 1.000000000000000000, 1.000000000000000000, 1.000000000000000000, 1.000000000000000000, 1.000000000000000000, 1.000000000000000000, 1.000000000000000000, 1.000000000000000000, 1.000000000000000000) ) ) 
 REPRESENTATION_ITEM ( '' )  SURFACE ( )  );
#106586=B_SPLINE_CURVE_WITH_KNOTS ( 'NONE', 3,
 ( #51983, #16247, #81284, #34650, #146311, #131163, #150560, #33588, #1062, #163612, #17317, #180906, #18391, #113861, #82333, #101789, #63964, #114908, #183034, #35712, #62647, #67127, #197154, #50911, #184093, #100720, #84468, #48791, #2120, #68195 ),
 .UNSPECIFIED., .F., .F.,
 ( 4, 2, 2, 2, 2, 2, 2, 2, 2, 2, 2, 2, 2, 2, 4 ),
 ( -5.999999999772596264E-08, 0.0009256177583834637734, 0.001851295516766925239, 0.002776973275150386271, 0.003702651033533847953, 0.004628328791917308768, 0.005554006550300769583, 0.006479684308684230398, 0.007405362067067692081, 0.009256717583834615445, 0.01018239534221807886, 0.01110807310060153881, 0.01203375085898500049, 0.01295942861736846217, 0.01481078413413538554 ),
 .UNSPECIFIED. ) ;
#106615=SURFACE_STYLE_USAGE ( .BOTH. , #142301 ) ;
#106617=ORIENTED_EDGE ( 'NONE', *, *, #32909, .T. ) ;
#106625=CARTESIAN_POINT ( 'NONE',  ( 9.013329340612937557, 11.11377505082129069, -8.022259956411712523 ) ) ;
#106629=CARTESIAN_POINT ( 'NONE',  ( -11.48243876534946040, 9.799999999999998934, -3.200000000000001510 ) ) ;
#106632=ORIENTED_EDGE ( 'NONE', *, *, #51505, .T. ) ;
#106640=CARTESIAN_POINT ( 'NONE',  ( 9.333041836227119248, 3.553052365627043407, -7.472413793103452662 ) ) ;
#106651=CARTESIAN_POINT ( 'NONE',  ( -11.95061148709128140, 8.982475982309534146, -1.242198177808604198 ) ) ;
#106703=VECTOR ( 'NONE', #127459, 1000.000000000000000 ) ;
#106706=FACE_OUTER_BOUND ( 'NONE', #18379, .T. ) ;
#106724=CARTESIAN_POINT ( 'NONE',  ( 7.416522329255045065, 14.99999999999999645, -9.452665224861386051 ) ) ;
#106731=CARTESIAN_POINT ( 'NONE',  ( 9.257559171758622085, 13.68169161456526162, 6.840446529487702598 ) ) ;
#106751=CARTESIAN_POINT ( 'NONE',  ( -11.04536101718726293, 10.19999999999999929, -1.100000000000000311 ) ) ;
#106763=AXIS2_PLACEMENT_3D ( 'NONE', #46852, #99845, #131338 ) ;
#106765=CARTESIAN_POINT ( 'NONE',  ( -11.79406710134376191, 4.782197168659454434, 4.941180684906744780 ) ) ;
#106768=CARTESIAN_POINT ( 'NONE',  ( -10.95308175811721085, 12.30000000000000071, -1.800000000000001155 ) ) ;
#106779=DIRECTION ( 'NONE',  ( 1.000000000000000000, -0.000000000000000000, -0.000000000000000000 ) ) ;
#106785=ORIENTED_EDGE ( 'NONE', *, *, #89006, .F. ) ;
#106790=EDGE_LOOP ( 'NONE', ( #34878, #119835, #51225, #32839 ) ) ;
#106792=CARTESIAN_POINT ( 'NONE',  ( 9.768119350134290002, 11.88398385152791903, 6.892589425638673717 ) ) ;
#106822=B_SPLINE_CURVE_WITH_KNOTS ( 'NONE', 3,
 ( #206911, #122575, #140900, #188537, #123640, #109499 ),
 .UNSPECIFIED., .F., .F.,
 ( 4, 2, 4 ),
 ( 0.000000000000000000, 0.0003132070624402877746, 0.0006264141248805755492 ),
 .UNSPECIFIED. ) ;
#106829=FILL_AREA_STYLE ('',( #90542 ) ) ;
#106842=FILL_AREA_STYLE_COLOUR ( '', #101685 ) ;
#106857=SURFACE_STYLE_FILL_AREA ( #139319 ) ;
#106868=ORIENTED_EDGE ( 'NONE', *, *, #191917, .T. ) ;
#106874=( NAMED_UNIT ( * ) SI_UNIT ( $, .STERADIAN. ) SOLID_ANGLE_UNIT ( ) );
#106881=EDGE_CURVE ( 'NONE', #19175, #54861, #96681, .T. ) ;
#106885=CARTESIAN_POINT ( 'NONE',  ( -10.88575987782614796, 5.812703298851592315, -6.395352192321499984 ) ) ;
#106890=CARTESIAN_POINT ( 'NONE',  ( 8.361447513987284808, 14.02696274858952030, 8.607981746264741219 ) ) ;
#106907=CARTESIAN_POINT ( 'NONE',  ( -11.78331023100045627, 12.29999999999998295, 1.799999999999999600 ) ) ;
#106916=ORIENTED_EDGE ( 'NONE', *, *, #151300, .T. ) ;
#106929=DIRECTION ( 'NONE',  ( 1.000000000000000000, 0.000000000000000000, 0.000000000000000000 ) ) ;
#106961=CARTESIAN_POINT ( 'NONE',  ( -9.979823206198361163, 5.589814398814591634, -5.978750339097100408 ) ) ;
#106962=STYLED_ITEM ( 'NONE', ( #184660 ), #213132 ) ;
#106985=CARTESIAN_POINT ( 'NONE',  ( -15.75000000000000000, 10.19999999999998153, 3.199999999999997957 ) ) ;
#107014=EDGE_LOOP ( 'NONE', ( #160259, #71249, #22437, #70535 ) ) ;
#107024=CARTESIAN_POINT ( 'NONE',  ( 11.87716655177446157, 6.749247459756340994, -1.730190197624842829 ) ) ;
#107032=CARTESIAN_POINT ( 'NONE',  ( -15.75000000000000000, 10.90000000000000036, -3.600000000000002309 ) ) ;
#107039=( LENGTH_UNIT ( ) NAMED_UNIT ( * ) SI_UNIT ( .MILLI., .METRE. ) );
#107058=DIRECTION ( 'NONE',  ( -0.000000000000000000, -1.000000000000000000, -0.000000000000000000 ) ) ;
#107144=CARTESIAN_POINT ( 'NONE',  ( 11.41381675112453387, 13.40000000000000036, -3.704697986577182522 ) ) ;
#107145=CARTESIAN_POINT ( 'NONE',  ( -11.33772463945037146, 10.19999999999998153, 3.599999999999999201 ) ) ;
#107159=CARTESIAN_POINT ( 'NONE',  ( 0.001697632222342148299, 14.56227640660409683, 11.93887725717812209 ) ) ;
#107160=CARTESIAN_POINT ( 'NONE',  ( -11.86145016429273191, 13.40000000000000036, 1.099999999999996980 ) ) ;
#107161=CARTESIAN_POINT ( 'NONE',  ( -10.28135750008142324, 4.005690466847553033, 7.422021812076344816 ) ) ;
#107167=CARTESIAN_POINT ( 'NONE',  ( -11.84668730067608422, 10.90000000000000036, -1.400000000000001688 ) ) ;
#107204=DIRECTION ( 'NONE',  ( 1.000000000000000000, -0.000000000000000000, -0.000000000000000000 ) ) ;
#107209=ORIENTED_EDGE ( 'NONE', *, *, #117977, .T. ) ;
#107210=B_SPLINE_CURVE_WITH_KNOTS ( 'NONE', 3,
 ( #43448, #58610, #174521, #124765, #26097, #190724 ),
 .UNSPECIFIED., .F., .F.,
 ( 4, 2, 4 ),
 ( 0.000000000000000000, 0.0003168911866439334617, 0.0006337823732878669234 ),
 .UNSPECIFIED. ) ;
#107217=CARTESIAN_POINT ( 'NONE',  ( -9.052987461608243080, 14.55305228048848676, 7.822201588416328732 ) ) ;
#107218=DIRECTION ( 'NONE',  ( 0.000000000000000000, 0.000000000000000000, 1.000000000000000000 ) ) ;
#107229=DIRECTION ( 'NONE',  ( 0.000000000000000000, -1.000000000000000000, 0.000000000000000000 ) ) ;
#107237=ORIENTED_EDGE ( 'NONE', *, *, #100151, .F. ) ;
#107253=ORIENTED_EDGE ( 'NONE', *, *, #78683, .T. ) ;
#107261=CARTESIAN_POINT ( 'NONE',  ( 0.05568803613164878541, 15.46908327293036400, 11.99987078441405508 ) ) ;
#107276=CARTESIAN_POINT ( 'NONE',  ( 9.348381460497192208, 13.52536904890506797, 7.450314784081282227 ) ) ;
#107296=FACE_OUTER_BOUND ( 'NONE', #125728, .T. ) ;
#107305=CARTESIAN_POINT ( 'NONE',  ( -0.06970559732546230403, 15.50808405863728723, 11.99964040566943346 ) ) ;
#107306=CARTESIAN_POINT ( 'NONE',  ( -10.83925572545687999, 5.627432043407305962, 6.488667418600654102 ) ) ;
#107321=DIRECTION ( 'NONE',  ( 1.000000000000000000, -0.000000000000000000, -0.000000000000000000 ) ) ;
#107337=CARTESIAN_POINT ( 'NONE',  ( -11.48243876534946217, 12.21999999999998288, 3.199999999999997957 ) ) ;
#107357=CARTESIAN_POINT ( 'NONE',  ( -6.714760661030930500, 14.53011251428762840, 9.955875793587102507 ) ) ;
#107370=CYLINDRICAL_SURFACE ( 'NONE', #179386, 0.3999999999999997446 ) ;
#107386=ORIENTED_EDGE ( 'NONE', *, *, #173872, .T. ) ;
#107389=VECTOR ( 'NONE', #197687, 1000.000000000000000 ) ;
#107406=CARTESIAN_POINT ( 'NONE',  ( -11.41381675112453564, 11.03005666089993220, -3.704697986577182522 ) ) ;
#107421=ORIENTED_EDGE ( 'NONE', *, *, #207656, .T. ) ;
#107426=CARTESIAN_POINT ( 'NONE',  ( 11.52469724861194145, 9.720000066487687107, -3.346365485506883175 ) ) ;
#107431=CIRCLE ( 'NONE', #186806, 12.00000000000000355 ) ;
#107432=ORIENTED_EDGE ( 'NONE', *, *, #16992, .T. ) ;
#107447=CARTESIAN_POINT ( 'NONE',  ( -10.60630082101195804, 5.715768461961713953, -4.896526734066639186 ) ) ;
#107449=CARTESIAN_POINT ( 'NONE',  ( -11.44786932348540986, 9.799999999999982947, 3.303370173849762725 ) ) ;
#107451=DIRECTION ( 'NONE',  ( 0.000000000000000000, 0.000000000000000000, -1.000000000000000000 ) ) ;
#107455=CARTESIAN_POINT ( 'NONE',  ( -10.62873463776380056, 13.79999999999998295, 3.199999999999997957 ) ) ;
#107468=CARTESIAN_POINT ( 'NONE',  ( -11.48243876534946217, 9.719999999999998863, -3.200000000000001510 ) ) ;
#107473=EDGE_CURVE ( 'NONE', #212473, #30537, #4980, .T. ) ;
#107495=CARTESIAN_POINT ( 'NONE',  ( 11.92619526913699879, 13.39999999999998259, 1.328859060402684644 ) ) ;
#107516=DIRECTION ( 'NONE',  ( -0.000000000000000000, 1.000000000000000000, -0.000000000000000000 ) ) ;
#107557=DIRECTION ( 'NONE',  ( 0.000000000000000000, -1.000000000000000000, -1.804652791718263484E-16 ) ) ;
#107569=UNCERTAINTY_MEASURE_WITH_UNIT (LENGTH_MEASURE( 1.000000000000000082E-05 ), #50152, 'distance_accuracy_value', 'NONE');
#107574=CARTESIAN_POINT ( 'NONE',  ( 11.92619526913699879, 10.19999999999998153, 1.328859060402684644 ) ) ;
#107578=DIRECTION ( 'NONE',  ( -3.491481338843133750E-15, -0.000000000000000000, -1.000000000000000000 ) ) ;
#107589=VECTOR ( 'NONE', #47396, 1000.000000000000000 ) ;
#107618=CARTESIAN_POINT ( 'NONE',  ( -11.69380381030441107, 8.410673437356566140, -1.083569014401829955 ) ) ;
#107621=CARTESIAN_POINT ( 'NONE',  ( 11.89942855770814312, 11.29999999999999893, -0.7000000000000009548 ) ) ;
#107623=CARTESIAN_POINT ( 'NONE',  ( -11.89197369110780045, 9.800000000000000711, -0.8056055387119882560 ) ) ;
#107692=ORIENTED_EDGE ( 'NONE', *, *, #192009, .F. ) ;
#107698=FACE_OUTER_BOUND ( 'NONE', #189269, .T. ) ;
#107709=CARTESIAN_POINT ( 'NONE',  ( 8.816397291392808810, 13.32355858800980464, 7.672907388467486989 ) ) ;
#107712=ORIENTED_EDGE ( 'NONE', *, *, #75384, .F. ) ;
#107717=ORIENTED_EDGE ( 'NONE', *, *, #203982, .T. ) ;
#107726=CARTESIAN_POINT ( 'NONE',  ( 9.622290429756468200, 3.756446959784728534, -7.170831222936548066 ) ) ;
#107739=CARTESIAN_POINT ( 'NONE',  ( -10.50059885609813115, 5.377696206510352184, -5.808392519734754345 ) ) ;
#107755=CARTESIAN_POINT ( 'NONE',  ( 11.88168509644349058, 12.21999999999999886, -1.685788023084331400 ) ) ;
#107793=MECHANICAL_DESIGN_GEOMETRIC_PRESENTATION_REPRESENTATION('',(#149100),#35041);
#107812=CARTESIAN_POINT ( 'NONE',  ( 9.167121402339585501, 14.44227982134217569, -8.755495446810726889 ) ) ;
#107814=CARTESIAN_POINT ( 'NONE',  ( 9.227221554775363543, 13.86401727962134878, 6.887592563684543201 ) ) ;
#107846=CARTESIAN_POINT ( 'NONE',  ( -11.87988507903381219, 5.100570458969788668, 4.764376171217361566 ) ) ;
#107855=CARTESIAN_POINT ( 'NONE',  ( -15.75000000000000000, 13.40000000000000036, -3.600000000000002309 ) ) ;
#107860=EDGE_CURVE ( 'NONE', #134499, #12777, #167623, .T. ) ;
#107887=( NAMED_UNIT ( * ) SI_UNIT ( $, .STERADIAN. ) SOLID_ANGLE_UNIT ( ) );
#107893=AXIS2_PLACEMENT_3D ( 'NONE', #47971, #132428, #82557 ) ;
#107910=EDGE_CURVE ( 'NONE', #181742, #148656, #163121, .T. ) ;
#107928=CARTESIAN_POINT ( 'NONE',  ( -9.367496997608917297, 14.57669131241553728, -7.413898975919227752 ) ) ;
#107965=CARTESIAN_POINT ( 'NONE',  ( -12.15057777967900243, 9.234859088329544718, 2.778757836088345812 ) ) ;
#107970=PRESENTATION_STYLE_ASSIGNMENT (( #124242 ) ) ;
#107983=MECHANICAL_DESIGN_GEOMETRIC_PRESENTATION_REPRESENTATION('',(#145980),#163273);
#108005=( LENGTH_UNIT ( ) NAMED_UNIT ( * ) SI_UNIT ( .MILLI., .METRE. ) );
#108033=( NAMED_UNIT ( * ) PLANE_ANGLE_UNIT ( ) SI_UNIT ( $, .RADIAN. ) );
#108038=CARTESIAN_POINT ( 'NONE',  ( -11.75342398721120141, 4.618418902329548992, -5.022351803590792585 ) ) ;
#108043=MECHANICAL_DESIGN_GEOMETRIC_PRESENTATION_REPRESENTATION('',(#194545),#4186);
#108056=VERTEX_POINT ( 'NONE', #144031 ) ;
#108102=CARTESIAN_POINT ( 'NONE',  ( 10.50000000000000178, 10.89999999999998259, 3.599999999999999201 ) ) ;
#108141=CARTESIAN_POINT ( 'NONE',  ( -11.04536101718726293, 0.000000000000000000, 1.099999999999996758 ) ) ;
#108191=AXIS2_PLACEMENT_3D ( 'NONE', #152239, #153299, #4875 ) ;
#108198=CARTESIAN_POINT ( 'NONE',  ( 11.94105721237523277, 19.00000000000000000, 1.187919463087248273 ) ) ;
#108228=CARTESIAN_POINT ( 'NONE',  ( 11.78331023100045627, 13.79999999999998295, 1.799999999999999600 ) ) ;
#108230=ORIENTED_EDGE ( 'NONE', *, *, #14440, .T. ) ;
#108235=CARTESIAN_POINT ( 'NONE',  ( -11.29165584589917870, 5.103824637450834700, 5.764786465619509137 ) ) ;
#108250=MECHANICAL_DESIGN_GEOMETRIC_PRESENTATION_REPRESENTATION('',(#104800),#836);
#108263=CARTESIAN_POINT ( 'NONE',  ( -10.44369633504468631, 5.112959841837461994, -5.232137017608345708 ) ) ;
#108291=SURFACE_STYLE_FILL_AREA ( #24821 ) ;
#108300=EDGE_CURVE ( 'NONE', #91407, #122503, #163445, .T. ) ;
#108304=CARTESIAN_POINT ( 'NONE',  ( -10.41646471606764024, 3.952576377580180989, 5.868867284226453762 ) ) ;
#108313=( NAMED_UNIT ( * ) SI_UNIT ( $, .STERADIAN. ) SOLID_ANGLE_UNIT ( ) );
#108333=CARTESIAN_POINT ( 'NONE',  ( -1.748134023616016330, 15.47021538507039828, 11.90627320348867357 ) ) ;
#108366=SURFACE_STYLE_FILL_AREA ( #88868 ) ;
#108367=EDGE_CURVE ( 'NONE', #118849, #52465, #53337, .T. ) ;
#108369=PRESENTATION_STYLE_ASSIGNMENT (( #206853 ) ) ;
#108377=CARTESIAN_POINT ( 'NONE',  ( -10.87092197480563271, 4.494752981060541330, 4.557748927716649412 ) ) ;
#108395=CARTESIAN_POINT ( 'NONE',  ( -1.673491136019439323E-15, 4.000007913748541810, -11.67999999982603399 ) ) ;
#108406=VERTEX_POINT ( 'NONE', #211139 ) ;
#108416=EDGE_CURVE ( 'NONE', #4829, #115502, #87500, .T. ) ;
#108431=CARTESIAN_POINT ( 'NONE',  ( -5.520326499667782549, 14.55310517179796470, 10.61470576409842614 ) ) ;
#108448=B_SPLINE_CURVE_WITH_KNOTS ( 'NONE', 3,
 ( #208891, #107217, #7494, #174310, #57337, #126683, #172161, #11766, #24819, #10698, #76768, #90921, #188390, #156986, #205702, #125619, #44298, #124559 ),
 .UNSPECIFIED., .F., .F.,
 ( 4, 2, 2, 2, 2, 2, 2, 2, 4 ),
 ( -5.999999999904574585E-08, 0.001344200983021300467, 0.002688461966042599710, 0.004032722949063899387, 0.005376983932085199064, 0.006721244915106497873, 0.008065505898127794948, 0.009409766881149092890, 0.01075402786417039083 ),
 .UNSPECIFIED. ) ;
#108452=DIRECTION ( 'NONE',  ( 0.000000000000000000, -1.000000000000000000, 0.000000000000000000 ) ) ;
#108465=CARTESIAN_POINT ( 'NONE',  ( 10.56536251450128994, 13.75961062549474612, 3.404319718479180690 ) ) ;
#108475=CARTESIAN_POINT ( 'NONE',  ( -11.78331023100045627, 11.29999999999999893, -1.800000000000001155 ) ) ;
#108481=DIRECTION ( 'NONE',  ( 0.8736852521944931116, 0.05518364616837929254, 0.4833516786910004304 ) ) ;
#108486=CARTESIAN_POINT ( 'NONE',  ( -15.75000000000000000, 10.19999999999999929, -1.800000000000001155 ) ) ;
#108495=LINE ( 'NONE', #158260, #161238 ) ;
#108500=VERTEX_POINT ( 'NONE', #108395 ) ;
#108515=CARTESIAN_POINT ( 'NONE',  ( -11.52469724861192901, 9.720000066487669343, 3.346365485506925808 ) ) ;
#108540=CARTESIAN_POINT ( 'NONE',  ( -10.97010717055062656, 9.799999999999997158, -1.696399592028410952 ) ) ;
#108546=CARTESIAN_POINT ( 'NONE',  ( 1.359357947053562156E-15, 0.08000000000000020983, -11.09999999999999964 ) ) ;
#108560=CARTESIAN_POINT ( 'NONE',  ( -15.75000000000000000, 9.799999999999998934, 0.6999999999999992895 ) ) ;
#108571=EDGE_LOOP ( 'NONE', ( #6405, #6003, #144615, #88361, #135615, #175765, #167576, #15753 ) ) ;
#108574=ORIENTED_EDGE ( 'NONE', *, *, #98948, .T. ) ;
#108639=CARTESIAN_POINT ( 'NONE',  ( 11.86239285000045740, 9.719999999999982876, 1.812080536912751061 ) ) ;
#108640=VERTEX_POINT ( 'NONE', #104891 ) ;
#108644=LINE ( 'NONE', #21951, #15840 ) ;
#108669=CARTESIAN_POINT ( 'NONE',  ( -1.499999999999964029, 7.000000000000000000, 9.886859966642596476 ) ) ;
#108696=LINE ( 'NONE', #174724, #135218 ) ;
#108717=CARTESIAN_POINT ( 'NONE',  ( 11.97185388258315264, 11.37999990720392418, -0.8311143155443054820 ) ) ;
#108722=COLOUR_RGB ( '', 0.31764706, 0.68627451, 0.89019608) ;
#108729=FILL_AREA_STYLE ('',( #126058 ) ) ;
#108736=DIRECTION ( 'NONE',  ( 0.5773502691896272854, 0.000000000000000000, -0.8164965809277250353 ) ) ;
#108752=CARTESIAN_POINT ( 'NONE',  ( -11.43209210103587559, 12.44403924016082819, 3.649125173352122609 ) ) ;
#108755=CARTESIAN_POINT ( 'NONE',  ( -11.89942855770814134, 11.37999999999999901, -0.7000000000000009548 ) ) ;
#108764=( NAMED_UNIT ( * ) PLANE_ANGLE_UNIT ( ) SI_UNIT ( $, .RADIAN. ) );
#108776=CARTESIAN_POINT ( 'NONE',  ( 8.847373858153110504, 13.14833187437462314, 7.638329839124071263 ) ) ;
#108782=EDGE_LOOP ( 'NONE', ( #20239, #59165, #208835, #34637 ) ) ;
#108791=CARTESIAN_POINT ( 'NONE',  ( -4.379728263269426769, 15.51893462896019038, -11.18122698975924223 ) ) ;
#108793=CARTESIAN_POINT ( 'NONE',  ( 9.649767104172513044, 4.268299563709507360, -7.133807922836931326 ) ) ;
#108821=DIRECTION ( 'NONE',  ( -0.000000000000000000, -1.000000000000000000, -0.000000000000000000 ) ) ;
#108834=CARTESIAN_POINT ( 'NONE',  ( -6.671583288098545061, 16.00000000000403588, 9.747470831330232954 ) ) ;
#108845=CARTESIAN_POINT ( 'NONE',  ( 11.07124251632621537, 9.800000000000000711, -0.8054525327832628978 ) ) ;
#108854=SURFACE_STYLE_FILL_AREA ( #191082 ) ;
#108862=SURFACE_SIDE_STYLE ('',( #157562 ) ) ;
#108876=CARTESIAN_POINT ( 'NONE',  ( 11.99904264826913725, 7.001436028495777286, 0.9608145573154694974 ) ) ;
#108883=CARTESIAN_POINT ( 'NONE',  ( -11.92619526913699879, 13.40000000000000036, -1.328859060402686199 ) ) ;
#108906=SURFACE_SIDE_STYLE ('',( #41728 ) ) ;
#108910=AXIS2_PLACEMENT_3D ( 'NONE', #119979, #152410, #202188 ) ;
#108916=CARTESIAN_POINT ( 'NONE',  ( -11.50790213655337979, 7.746734403679841563, -4.957264960544601529 ) ) ;
#108941=CARTESIAN_POINT ( 'NONE',  ( 10.85609235738973588, 9.597193135844154455, 5.125747691056198541 ) ) ;
#108972=EDGE_CURVE ( 'NONE', #19630, #97972, #150289, .T. ) ;
#108991=FACE_OUTER_BOUND ( 'NONE', #78809, .T. ) ;
#109004=SURFACE_SIDE_STYLE ('',( #106857 ) ) ;
#109030=CARTESIAN_POINT ( 'NONE',  ( -9.986107380900749675, 5.615474669794299878, -5.966265754238714969 ) ) ;
#109054=CIRCLE ( 'NONE', #160796, 11.09999999999999964 ) ;
#109066=AXIS2_PLACEMENT_3D ( 'NONE', #2885, #22341, #35406 ) ;
#109084=ORIENTED_EDGE ( 'NONE', *, *, #81005, .T. ) ;
#109099=B_SPLINE_CURVE_WITH_KNOTS ( 'NONE', 3,
 ( #15307, #115026, #198322, #146429, #81395, #100834 ),
 .UNSPECIFIED., .F., .F.,
 ( 4, 2, 4 ),
 ( 0.000000000000000000, 0.0003141588434155108628, 0.0006283176868310217256 ),
 .UNSPECIFIED. ) ;
#109107=CARTESIAN_POINT ( 'NONE',  ( -10.82993273518205690, 5.589502548902120616, -6.507125152095314391 ) ) ;
#109161=DIRECTION ( 'NONE',  ( 0.5994789404140892231, -6.777585655618907357E-14, -0.8003905296791067325 ) ) ;
#109175=CARTESIAN_POINT ( 'NONE',  ( 11.84668730067608777, 13.50634727754795250, -1.400000000000001910 ) ) ;
#109183=DIRECTION ( 'NONE',  ( 0.000000000000000000, 7.254698431504986582E-17, -1.000000000000000000 ) ) ;
#109206=UNCERTAINTY_MEASURE_WITH_UNIT (LENGTH_MEASURE( 1.000000000000000082E-05 ), #79686, 'distance_accuracy_value', 'NONE');
#109211=CARTESIAN_POINT ( 'NONE',  ( 11.92008656065780947, 6.690339256190793726, -0.9868697903839722674 ) ) ;
#109214=CARTESIAN_POINT ( 'NONE',  ( -10.44512553078396344, 5.055828132299228450, 5.909874117198688381 ) ) ;
#109218=CARTESIAN_POINT ( 'NONE',  ( -4.428767733937130302, 15.51888673063479196, 11.16163516131764233 ) ) ;
#109231=CARTESIAN_POINT ( 'NONE',  ( 11.41157692552970815, 12.34089662913000573, -3.404533818002362100 ) ) ;
#109239=FACE_OUTER_BOUND ( 'NONE', #122049, .T. ) ;
#109252=LINE ( 'NONE', #195758, #107589 ) ;
#109297=CARTESIAN_POINT ( 'NONE',  ( 11.89839339040395139, 13.82877468403908772, 1.560885614203548100 ) ) ;
#109302=CARTESIAN_POINT ( 'NONE',  ( 11.57394138716773213, 8.953477593029530723, 4.723522898263817993 ) ) ;
#109303=CARTESIAN_POINT ( 'NONE',  ( -10.77299012366456310, 5.423410747438590640, 6.621146351739780833 ) ) ;
#109310=CARTESIAN_POINT ( 'NONE',  ( -15.75000000000000000, 12.69999999999999929, -0.7000000000000009548 ) ) ;
#109353=CARTESIAN_POINT ( 'NONE',  ( -11.01135777277262129, 13.39999999999998259, 1.399999999999998579 ) ) ;
#109370=SURFACE_SIDE_STYLE ('',( #43252 ) ) ;
#109374=CARTESIAN_POINT ( 'NONE',  ( -10.62413147216588527, 4.107683970518822392, 5.580188593819120690 ) ) ;
#109377=ORIENTED_EDGE ( 'NONE', *, *, #202242, .T. ) ;
#109386=CIRCLE ( 'NONE', #15902, 0.07999999999999946043 ) ;
#109405=CARTESIAN_POINT ( 'NONE',  ( -11.41381675112453387, 12.69999999999999929, -3.704697986577184299 ) ) ;
#109407=LINE ( 'NONE', #56317, #66040 ) ;
#109423=DIRECTION ( 'NONE',  ( 1.000000000000000000, -0.000000000000000000, -0.000000000000000000 ) ) ;
#109444=CARTESIAN_POINT ( 'NONE',  ( 11.41381675112453564, 12.56994333910006567, -3.704697986577182522 ) ) ;
#109446=CARTESIAN_POINT ( 'NONE',  ( 11.94654170777226021, 12.44825673841064173, -1.134972293687621647 ) ) ;
#109452=EDGE_LOOP ( 'NONE', ( #76823, #119153, #542, #198372 ) ) ;
#109455=UNCERTAINTY_MEASURE_WITH_UNIT (LENGTH_MEASURE( 1.000000000000000082E-05 ), #90516, 'distance_accuracy_value', 'NONE');
#109480=CARTESIAN_POINT ( 'NONE',  ( 0.000000000000000000, 4.518459255872631530, 11.92000000000000348 ) ) ;
#109488=DIRECTION ( 'NONE',  ( -0.000000000000000000, 1.000000000000000000, -0.000000000000000000 ) ) ;
#109499=CARTESIAN_POINT ( 'NONE',  ( -11.07790593930098311, 12.30000000000000071, -0.7000000000000009548 ) ) ;
#109505=CARTESIAN_POINT ( 'NONE',  ( 11.86239285000045562, 12.29999999999998472, 1.812080536912751061 ) ) ;
#109535=CARTESIAN_POINT ( 'NONE',  ( 11.78331023100045627, 11.29999999999998117, 1.799999999999999600 ) ) ;
#109553=PRESENTATION_STYLE_ASSIGNMENT (( #143086 ) ) ;
#109574=ORIENTED_EDGE ( 'NONE', *, *, #163044, .T. ) ;
#109578=VERTEX_POINT ( 'NONE', #163236 ) ;
#109588=CARTESIAN_POINT ( 'NONE',  ( -10.79318656363365569, 4.699712429332246089, -5.142077722257549333 ) ) ;
#109590=CARTESIAN_POINT ( 'NONE',  ( 7.322143911241490777, 14.00158514652465591, 10.35507522492528132 ) ) ;
#109592=DIRECTION ( 'NONE',  ( 0.6250000204279239080, -1.312437604053124089E-08, -0.7806247334443706665 ) ) ;
#109596=CARTESIAN_POINT ( 'NONE',  ( 0.000000000000000000, 9.799999999999998934, 0.000000000000000000 ) ) ;
#109597=B_SPLINE_CURVE_WITH_KNOTS ( 'NONE', 3,
 ( #1442, #67507, #203915, #171442, #88061, #76076 ),
 .UNSPECIFIED., .F., .F.,
 ( 4, 2, 4 ),
 ( 0.001916662113439827810, 0.002237152494173779652, 0.002557642874907731494 ),
 .UNSPECIFIED. ) ;
#109604=EDGE_CURVE ( 'NONE', #85120, #36225, #145943, .T. ) ;
#109605=CARTESIAN_POINT ( 'NONE',  ( 11.94980361490430099, 12.59667875264130288, 1.099999952233555733 ) ) ;
#109615=LINE ( 'NONE', #175620, #14627 ) ;
#109621=CARTESIAN_POINT ( 'NONE',  ( -11.33772463945037146, 19.00000000000000000, 3.679999999999999272 ) ) ;
#109622=LINE ( 'NONE', #207030, #30393 ) ;
#109640=FILL_AREA_STYLE ('',( #209167 ) ) ;
#109642=ORIENTED_EDGE ( 'NONE', *, *, #55681, .F. ) ;
#109646=CARTESIAN_POINT ( 'NONE',  ( -11.43204722947019825, 13.65592754026171818, 3.649275849833181429 ) ) ;
#109689=ORIENTED_EDGE ( 'NONE', *, *, #102711, .T. ) ;
#109697=STYLED_ITEM ( 'NONE', ( #102386 ), #143536 ) ;
#109698=CARTESIAN_POINT ( 'NONE',  ( 8.917979296484501717, 14.68769155229934142, 8.032863906691817490 ) ) ;
#109762=LINE ( 'NONE', #144372, #41262 ) ;
#109763=CARTESIAN_POINT ( 'NONE',  ( -4.369858682569394581, 14.55265096709559280, -11.13738628252537310 ) ) ;
#109764=CARTESIAN_POINT ( 'NONE',  ( -11.88237951145550042, 9.843193473787149372, -0.9087114598430712231 ) ) ;
#109768=CARTESIAN_POINT ( 'NONE',  ( -11.33772463945037146, 13.50902469614650414, -3.600000000000000977 ) ) ;
#109794=AXIS2_PLACEMENT_3D ( 'NONE', #165488, #98363, #196921 ) ;
#109795=ORIENTED_EDGE ( 'NONE', *, *, #93697, .F. ) ;
#109810=CARTESIAN_POINT ( 'NONE',  ( -11.94980361723156292, 12.59761943414563312, 1.099999926404457984 ) ) ;
#109818=CARTESIAN_POINT ( 'NONE',  ( 0.000000000000000000, 8.500000000000000000, 0.000000000000000000 ) ) ;
#109827=( LENGTH_UNIT ( ) NAMED_UNIT ( * ) SI_UNIT ( .MILLI., .METRE. ) );
#109846=CARTESIAN_POINT ( 'NONE',  ( 11.18441447305199077, 7.671075215653008428, 3.641562284844301889 ) ) ;
#109864=CARTESIAN_POINT ( 'NONE',  ( 11.86145016429273191, 12.69999999999999929, 1.099999999999996758 ) ) ;
#109903=FACE_OUTER_BOUND ( 'NONE', #59666, .T. ) ;
#109907=CARTESIAN_POINT ( 'NONE',  ( -8.752560967067513076, 14.99999998465384365, 9.356054886187056496 ) ) ;
#109921=ORIENTED_EDGE ( 'NONE', *, *, #183326, .F. ) ;
#109935=CARTESIAN_POINT ( 'NONE',  ( -11.86239285000045918, 9.719999999999998863, -1.812080536912752837 ) ) ;
#109946=CARTESIAN_POINT ( 'NONE',  ( -9.604686356149276349, 3.999999999999997335, 7.193747284969079558 ) ) ;
#109953=CARTESIAN_POINT ( 'NONE',  ( 7.591119599213490332, 13.85210394378908028, 8.823496455125575011 ) ) ;
#109977=FILL_AREA_STYLE_COLOUR ( '', #74680 ) ;
#109987=CARTESIAN_POINT ( 'NONE',  ( -12.65133343644925823, 8.691152131673410608, 1.253321570098529181 ) ) ;
#110004=ORIENTED_EDGE ( 'NONE', *, *, #209722, .F. ) ;
#110010=CARTESIAN_POINT ( 'NONE',  ( 11.57758243856749303, 8.192336405874874217, -2.990131717548606627 ) ) ;
#110028=EDGE_CURVE ( 'NONE', #118348, #169237, #90884, .T. ) ;
#110058=CARTESIAN_POINT ( 'NONE',  ( -10.94893285264089577, 5.391538659128299216, 4.806406785934876247 ) ) ;
#110099=CARTESIAN_POINT ( 'NONE',  ( -10.28823555840286552, 6.680969737303435352, 5.325637450257892702 ) ) ;
#110126=EDGE_LOOP ( 'NONE', ( #16384, #16371, #206054, #33306 ) ) ;
#110129=DIRECTION ( 'NONE',  ( 1.000000000000000000, -0.000000000000000000, -0.000000000000000000 ) ) ;
#110172=CARTESIAN_POINT ( 'NONE',  ( -10.52626310920980757, 3.679096435225583939, -5.196420034295205603 ) ) ;
#110186=EDGE_CURVE ( 'NONE', #61426, #177833, #48758, .T. ) ;
#110192=CARTESIAN_POINT ( 'NONE',  ( 11.94105721237523277, 19.00000000000000000, -1.187919463087249827 ) ) ;
#110212=UNCERTAINTY_MEASURE_WITH_UNIT (LENGTH_MEASURE( 1.000000000000000082E-05 ), #176099, 'distance_accuracy_value', 'NONE');
#110239=LINE ( 'NONE', #191397, #170635 ) ;
#110252=CARTESIAN_POINT ( 'NONE',  ( 11.84104725192634966, 9.990164625485805416, 1.443823348526939165 ) ) ;
#110277=CARTESIAN_POINT ( 'NONE',  ( -9.568394635526177083, 14.89572081425755812, -7.242253469718477277 ) ) ;
#110293=EDGE_CURVE ( 'NONE', #167139, #47238, #92505, .T. ) ;
#110310=CARTESIAN_POINT ( 'NONE',  ( 8.571448334701180727, 14.94795601790086437, -8.335953519237410347 ) ) ;
#110334=ORIENTED_EDGE ( 'NONE', *, *, #132306, .T. ) ;
#110359=CARTESIAN_POINT ( 'NONE',  ( 11.84668729410370602, 13.50620512324527134, 1.399999999999998357 ) ) ;
#110364=CARTESIAN_POINT ( 'NONE',  ( 10.81010058466664425, 10.31570469300483950, 6.498163104334348183 ) ) ;
#110369=CIRCLE ( 'NONE', #93007, 0.07999999999999998779 ) ;
#110373=DIRECTION ( 'NONE',  ( 0.000000000000000000, 0.000000000000000000, -1.000000000000000000 ) ) ;
#110375=ORIENTED_EDGE ( 'NONE', *, *, #208819, .F. ) ;
#110380=VECTOR ( 'NONE', #21081, 1000.000000000000000 ) ;
#110409=EDGE_CURVE ( 'NONE', #12777, #211051, #120939, .T. ) ;
#110420=CARTESIAN_POINT ( 'NONE',  ( -11.84668730067608244, 11.00636224908218530, -1.400000000000002132 ) ) ;
#110435=CARTESIAN_POINT ( 'NONE',  ( -9.869385822740339265, 3.553052390425875284, 6.766708219044660133 ) ) ;
#110460=UNCERTAINTY_MEASURE_WITH_UNIT (LENGTH_MEASURE( 1.000000000000000082E-05 ), #176010, 'distance_accuracy_value', 'NONE');
#110475=FACE_OUTER_BOUND ( 'NONE', #38621, .T. ) ;
#110536=ADVANCED_FACE ( 'NONE', ( #34815 ), #191194, .T. ) ;
#110539=EDGE_CURVE ( 'NONE', #20115, #210323, #132375, .T. ) ;
#110561=CARTESIAN_POINT ( 'NONE',  ( -0.7616041399369541942, 14.48136325226530019, 12.01010946711977567 ) ) ;
#110569=CARTESIAN_POINT ( 'NONE',  ( -11.01135777277262306, 11.00623004977699715, -1.400000000000002132 ) ) ;
#110572=CARTESIAN_POINT ( 'NONE',  ( 11.43204722947019825, 11.15592754026173949, -3.649275849833183649 ) ) ;
#110594=CARTESIAN_POINT ( 'NONE',  ( 11.52469724861194145, 12.22000006648768711, -3.346365485506883175 ) ) ;
#110606=EDGE_CURVE ( 'NONE', #66261, #115079, #4405, .T. ) ;
#110613=DIRECTION ( 'NONE',  ( 0.000000000000000000, -1.000000000000000000, 0.000000000000000000 ) ) ;
#110640=CARTESIAN_POINT ( 'NONE',  ( -1.499999999999963141, 7.750000000000000000, -10.99818166789402518 ) ) ;
#110663=LINE ( 'NONE', #179864, #22848 ) ;
#110671=CARTESIAN_POINT ( 'NONE',  ( -11.55950211276791251, 13.88000000000000078, -3.221476510067115662 ) ) ;
#110692=CARTESIAN_POINT ( 'NONE',  ( -11.94105721237523099, 10.90000000000000036, 1.187919463087248273 ) ) ;
#110702=CARTESIAN_POINT ( 'NONE',  ( -9.951069066757307624, 4.531349380723807663, -6.628891310175081486 ) ) ;
#110704=ORIENTED_EDGE ( 'NONE', *, *, #119125, .F. ) ;
#110713=CARTESIAN_POINT ( 'NONE',  ( -11.94105721237522921, 12.57259609010266921, 1.187919463087244720 ) ) ;
#110720=COLOUR_RGB ( '', 0.66274510, 0.83137255, 0.94901961) ;
#110725=CARTESIAN_POINT ( 'NONE',  ( -11.94980361058168938, 13.40000000000000036, -1.100000000000000311 ) ) ;
#110737=FACE_OUTER_BOUND ( 'NONE', #73981, .T. ) ;
#110772=EDGE_CURVE ( 'NONE', #10371, #7674, #146255, .T. ) ;
#110784=ORIENTED_EDGE ( 'NONE', *, *, #179909, .F. ) ;
#110820=CARTESIAN_POINT ( 'NONE',  ( -9.976233718008073126, 4.600059191775173417, -6.670817322401115135 ) ) ;
#110829=( GEOMETRIC_REPRESENTATION_CONTEXT ( 3 ) GLOBAL_UNCERTAINTY_ASSIGNED_CONTEXT ( ( #23023 ) ) GLOBAL_UNIT_ASSIGNED_CONTEXT ( ( #88293, #153280, #42769 ) ) REPRESENTATION_CONTEXT ( 'NONE', 'WORKASPACE' ) );
#110849=ORIENTED_EDGE ( 'NONE', *, *, #185104, .T. ) ;
#110890=ORIENTED_EDGE ( 'NONE', *, *, #207656, .F. ) ;
#110899=ORIENTED_EDGE ( 'NONE', *, *, #72048, .F. ) ;
#110907=CARTESIAN_POINT ( 'NONE',  ( 12.32702100841206239, 6.004295755469880369, 1.110179225836540162 ) ) ;
#110938=CARTESIAN_POINT ( 'NONE',  ( -11.86145016429273014, 10.90000000000000036, -1.100000000000000533 ) ) ;
#110964=CARTESIAN_POINT ( 'NONE',  ( -1.724555757181258864, 13.99999999999692513, 11.68000002332616205 ) ) ;
#110965=CYLINDRICAL_SURFACE ( 'NONE', #90174, 0.07999999999999998779 ) ;
#111007=CARTESIAN_POINT ( 'NONE',  ( -10.71870444596734195, 5.124999999999999112, -5.395310463726811001 ) ) ;
#111011=CARTESIAN_POINT ( 'NONE',  ( 8.132223770642788452, 15.75611528059600097, -8.453506921246367156 ) ) ;
#111014=CARTESIAN_POINT ( 'NONE',  ( 8.332566079752199428, 13.17553009179483148, 8.539185921479196750 ) ) ;
#111020=EDGE_LOOP ( 'NONE', ( #115635, #212303, #185197, #36293 ) ) ;
#111035=CARTESIAN_POINT ( 'NONE',  ( -9.928151704202875294, 5.423124072284297270, 6.082134274749043001 ) ) ;
#111046=CARTESIAN_POINT ( 'NONE',  ( -10.48267169704037727, 5.268073273308885973, 5.153989745587932880 ) ) ;
#111061=EDGE_CURVE ( 'NONE', #109578, #93416, #45900, .T. ) ;
#111064=CARTESIAN_POINT ( 'NONE',  ( -9.498276863272749893, 14.58059102403192320, 7.333831086845977509 ) ) ;
#111070=ORIENTED_EDGE ( 'NONE', *, *, #153873, .T. ) ;
#111071=CARTESIAN_POINT ( 'NONE',  ( 11.95134404050519272, 7.565927718848042716, -0.2102339791074976649 ) ) ;
#111076=ORIENTED_EDGE ( 'NONE', *, *, #212414, .F. ) ;
#111078=AXIS2_PLACEMENT_3D ( 'NONE', #157978, #23674, #89784 ) ;
#111123=CARTESIAN_POINT ( 'NONE',  ( -11.31504510220803894, 6.390522733111290599, -4.000539294108416577 ) ) ;
#111127=LINE ( 'NONE', #177130, #48238 ) ;
#111152=EDGE_CURVE ( 'NONE', #41918, #20303, #48362, .T. ) ;
#111156=CARTESIAN_POINT ( 'NONE',  ( -11.96217875511318063, 12.27145633421023341, -0.9561995067075080845 ) ) ;
#111158=DIRECTION ( 'NONE',  ( 0.000000000000000000, 0.000000000000000000, 1.000000000000000000 ) ) ;
#111165=CARTESIAN_POINT ( 'NONE',  ( -12.76914910123260682, 7.416938840849524262, -2.145643146812736823 ) ) ;
#111184=CARTESIAN_POINT ( 'NONE',  ( -10.95308175811721085, 12.29999999999998295, 1.799999999999999600 ) ) ;
#111191=ORIENTED_EDGE ( 'NONE', *, *, #148232, .F. ) ;
#111199=AXIS2_PLACEMENT_3D ( 'NONE', #181580, #671, #146994 ) ;
#111216=ORIENTED_EDGE ( 'NONE', *, *, #86952, .T. ) ;
#111237=CARTESIAN_POINT ( 'NONE',  ( -9.917242840447775265, 4.174869238508773783, -6.172972641688763140 ) ) ;
#111242=EDGE_LOOP ( 'NONE', ( #111920, #42560, #180341, #173071 ) ) ;
#111247=AXIS2_PLACEMENT_3D ( 'NONE', #98587, #212311, #32512 ) ;
#111258=FACE_OUTER_BOUND ( 'NONE', #28687, .T. ) ;
#111300=CIRCLE ( 'NONE', #100857, 11.92000000000000171 ) ;
#111316=ORIENTED_EDGE ( 'NONE', *, *, #104333, .T. ) ;
#111318=CARTESIAN_POINT ( 'NONE',  ( 11.86239285000045740, 9.719999999999982876, 1.812080536912751283 ) ) ;
#111334=CARTESIAN_POINT ( 'NONE',  ( 0.000000000000000000, 3.481540744127370690, 0.000000000000000000 ) ) ;
#111336=CARTESIAN_POINT ( 'NONE',  ( 9.287126810668082655, 11.47221324207556137, -7.528596418336154450 ) ) ;
#111364=CARTESIAN_POINT ( 'NONE',  ( 11.55950211276791251, 9.799999999999982947, 3.221476510067111665 ) ) ;
#111373=DIRECTION ( 'NONE',  ( 1.000000000000000000, -0.000000000000000000, -0.000000000000000000 ) ) ;
#111376=CARTESIAN_POINT ( 'NONE',  ( 8.349821703134351125, 15.09698064520563676, -8.558241530613692305 ) ) ;
#111417=CARTESIAN_POINT ( 'NONE',  ( 10.36376191611410746, 9.171481364675830861, -6.003992305501989257 ) ) ;
#111426=CARTESIAN_POINT ( 'NONE',  ( 11.86512089291903749, 8.353562777165519648, -1.599672920186862912 ) ) ;
#111434=CARTESIAN_POINT ( 'NONE',  ( -11.91826848676326200, 11.00833707238759374, -1.400000051401919077 ) ) ;
#111436=DIRECTION ( 'NONE',  ( 1.000000000000000000, -0.000000000000000000, -0.000000000000000000 ) ) ;
#111452=B_SPLINE_CURVE_WITH_KNOTS ( 'NONE', 3,
 ( #184523, #17743, #18820, #101145, #52414, #183468 ),
 .UNSPECIFIED., .F., .F.,
 ( 4, 2, 4 ),
 ( 0.0006378314054480060599, 0.0009584618939205532184, 0.001279092382393100377 ),
 .UNSPECIFIED. ) ;
#111481=( LENGTH_UNIT ( ) NAMED_UNIT ( * ) SI_UNIT ( .MILLI., .METRE. ) );
#111488=CARTESIAN_POINT ( 'NONE',  ( 9.406473150210953094, 3.553052365627046072, 7.380698111333699352 ) ) ;
#111498=CARTESIAN_POINT ( 'NONE',  ( -10.91033920341480723, 4.885615726745547782, 4.996448585388906238 ) ) ;
#111526=( GEOMETRIC_REPRESENTATION_CONTEXT ( 3 ) GLOBAL_UNCERTAINTY_ASSIGNED_CONTEXT ( ( #115579 ) ) GLOBAL_UNIT_ASSIGNED_CONTEXT ( ( #162627, #196188, #47830 ) ) REPRESENTATION_CONTEXT ( 'NONE', 'WORKASPACE' ) );
#111529=FACE_OUTER_BOUND ( 'NONE', #211869, .T. ) ;
#111538=( LENGTH_UNIT ( ) NAMED_UNIT ( * ) SI_UNIT ( .MILLI., .METRE. ) );
#111540=CARTESIAN_POINT ( 'NONE',  ( -15.75000000000000000, 13.79999999999998295, 3.199999999999997957 ) ) ;
#111577=ORIENTED_EDGE ( 'NONE', *, *, #61190, .T. ) ;
#111593=VECTOR ( 'NONE', #145550, 1000.000000000000000 ) ;
#111658=CARTESIAN_POINT ( 'NONE',  ( 11.92619526248521034, 11.02744613914163807, 1.328859120100916558 ) ) ;
#111664=ADVANCED_FACE ( 'NONE', ( #25896 ), #175378, .F. ) ;
#111692=TOROIDAL_SURFACE ( 'NONE', #56268, 11.92000000000000171, 0.08000000000000000167 ) ;
#111696=ORIENTED_EDGE ( 'NONE', *, *, #35037, .T. ) ;
#111721=CARTESIAN_POINT ( 'NONE',  ( -11.95360554405587017, 9.995550034974055365, -1.059413164304675359 ) ) ;
#111738=PRESENTATION_STYLE_ASSIGNMENT (( #48809 ) ) ;
#111757=EDGE_CURVE ( 'NONE', #197667, #148685, #7822, .T. ) ;
#111761=CARTESIAN_POINT ( 'NONE',  ( 7.690609288285140899, 14.45647329385417912, 9.157199668769314016 ) ) ;
#111791=CARTESIAN_POINT ( 'NONE',  ( 11.92619526913699701, 10.90000000000000036, -1.328859060402686199 ) ) ;
#111794=CARTESIAN_POINT ( 'NONE',  ( -11.41381675112453387, 12.69999999999998153, 3.704697986577180302 ) ) ;
#111806=ADVANCED_FACE ( 'NONE', ( #206782 ), #173252, .F. ) ;
#111807=CARTESIAN_POINT ( 'NONE',  ( -10.59781858645781405, 9.799999999999984723, 3.302687032930891498 ) ) ;
#111815=B_SPLINE_CURVE_WITH_KNOTS ( 'NONE', 3,
 ( #10232, #7007, #42774, #77372, #140278, #142414 ),
 .UNSPECIFIED., .F., .F.,
 ( 4, 2, 4 ),
 ( 0.000000000000000000, 0.0003845013059668469482, 0.0007690026119336938965 ),
 .UNSPECIFIED. ) ;
#111891=ORIENTED_EDGE ( 'NONE', *, *, #155462, .F. ) ;
#111920=ORIENTED_EDGE ( 'NONE', *, *, #80961, .T. ) ;
#111966=CARTESIAN_POINT ( 'NONE',  ( -15.75000000000000000, 11.29999999999998117, 1.799999999999999600 ) ) ;
#111976=FILL_AREA_STYLE_COLOUR ( '', #53439 ) ;
#111988=CARTESIAN_POINT ( 'NONE',  ( 9.272303875213562918, 13.02406837586111443, -8.983758935644893029 ) ) ;
#111993=ORIENTED_EDGE ( 'NONE', *, *, #160843, .T. ) ;
#112001=DIRECTION ( 'NONE',  ( 0.000000000000000000, 0.000000000000000000, -1.000000000000000000 ) ) ;
#112028=CARTESIAN_POINT ( 'NONE',  ( 0.000000000000000000, 0.08000000000000020983, 0.000000000000000000 ) ) ;
#112041=CARTESIAN_POINT ( 'NONE',  ( -10.84254087577847869, 4.919568073182958301, 5.035408296252059657 ) ) ;
#112044=CARTESIAN_POINT ( 'NONE',  ( -8.065673738752591859, 14.99999998464884854, 8.613976760015685130 ) ) ;
#112050=VECTOR ( 'NONE', #37035, 1000.000000000000000 ) ;
#112059=EDGE_LOOP ( 'NONE', ( #194903, #205919, #16256, #82854 ) ) ;
#112071=DIRECTION ( 'NONE',  ( -0.2684563758389304500, -5.222015543130708508E-15, 0.9632918427306581544 ) ) ;
#112084=FILL_AREA_STYLE ('',( #146672 ) ) ;
#112088=CARTESIAN_POINT ( 'NONE',  ( 9.885616400973860962, 14.58603459789345891, -7.683487713304058886 ) ) ;
#112091=CARTESIAN_POINT ( 'NONE',  ( 8.248303390504895916, 13.81254849593766565, 9.579712001821075518 ) ) ;
#112099=CARTESIAN_POINT ( 'NONE',  ( -11.41157692552970815, 11.25910337086999924, -3.404533818002362100 ) ) ;
#112122=CARTESIAN_POINT ( 'NONE',  ( -10.96033999287893224, 4.843182460328104177, 4.379153535238802242 ) ) ;
#112128=( GEOMETRIC_REPRESENTATION_CONTEXT ( 3 ) GLOBAL_UNCERTAINTY_ASSIGNED_CONTEXT ( ( #83008 ) ) GLOBAL_UNIT_ASSIGNED_CONTEXT ( ( #206182, #175848, #93537 ) ) REPRESENTATION_CONTEXT ( 'NONE', 'WORKASPACE' ) );
#112135=CARTESIAN_POINT ( 'NONE',  ( -11.92619526913700057, 19.00000000000000000, 1.328859060402684644 ) ) ;
#112140=CARTESIAN_POINT ( 'NONE',  ( -9.608223705632537914, 14.88228430527884605, 7.189021993539767230 ) ) ;
#112147=EDGE_LOOP ( 'NONE', ( #98154, #128490, #167473, #200836 ) ) ;
#112149=CARTESIAN_POINT ( 'NONE',  ( 11.08707159853939217, 9.067765128333563851, 4.459508006857516804 ) ) ;
#112153=DIRECTION ( 'NONE',  ( 0.000000000000000000, 0.000000000000000000, 1.000000000000000000 ) ) ;
#112193=DIRECTION ( 'NONE',  ( 1.000000000000000000, -0.000000000000000000, -0.000000000000000000 ) ) ;
#112196=CARTESIAN_POINT ( 'NONE',  ( -11.96362345633627200, 7.996868700864697921, 1.065082418458907609 ) ) ;
#112204=CARTESIAN_POINT ( 'NONE',  ( -11.89629718460002294, 8.889724561396670666, 1.217720464611954156 ) ) ;
#112215=ORIENTED_EDGE ( 'NONE', *, *, #76035, .T. ) ;
#112224=( NAMED_UNIT ( * ) SI_UNIT ( $, .STERADIAN. ) SOLID_ANGLE_UNIT ( ) );
#112234=CARTESIAN_POINT ( 'NONE',  ( -11.91002632418505058, 5.203875245307159503, 4.700031268430899800 ) ) ;
#112252=FILL_AREA_STYLE_COLOUR ( '', #172384 ) ;
#112254=CARTESIAN_POINT ( 'NONE',  ( 11.44800751629994906, 13.79999999999999893, -3.302956944461097777 ) ) ;
#112261=CARTESIAN_POINT ( 'NONE',  ( -9.053319117722196552, 15.44694771161291236, 7.821787350058786004 ) ) ;
#112272=CARTESIAN_POINT ( 'NONE',  ( 9.367496997597639208, 4.469082183885418225, 7.499999999999949374 ) ) ;
#112278=ADVANCED_FACE ( 'NONE', ( #70112 ), #86396, .T. ) ;
#112297=DIRECTION ( 'NONE',  ( 0.000000000000000000, 0.000000000000000000, -1.000000000000000000 ) ) ;
#112307=STYLED_ITEM ( 'NONE', ( #75641 ), #91304 ) ;
#112366=B_SPLINE_CURVE_WITH_KNOTS ( 'NONE', 3,
 ( #50634, #34376, #198988, #32256, #82060, #97276, #148152, #13852, #62609, #64747, #81004, #212044, #777 ),
 .UNSPECIFIED., .F., .F.,
 ( 4, 3, 3, 3, 4 ),
 ( 0.000000000000000000, 3.127676560591855702E-05, 7.184563044157459683E-05, 0.0001122497773744156145, 0.0001140446530104083958 ),
 .UNSPECIFIED. ) ;
#112398=FACE_OUTER_BOUND ( 'NONE', #115046, .T. ) ;
#112401=PRESENTATION_STYLE_ASSIGNMENT (( #162162 ) ) ;
#112404=CARTESIAN_POINT ( 'NONE',  ( -9.604686356149278126, 4.518459255872631530, 7.193747284969081335 ) ) ;
#112428=SURFACE_SIDE_STYLE ('',( #132902 ) ) ;
#112463=CARTESIAN_POINT ( 'NONE',  ( -10.95308175811721085, 11.29999999999998117, 1.799999999999999600 ) ) ;
#112488=CARTESIAN_POINT ( 'NONE',  ( 11.57754556164262993, 8.947311289249686439, -4.715264992745044736 ) ) ;
#112512=CARTESIAN_POINT ( 'NONE',  ( 9.333041836208478159, 3.553060279300227275, -7.472413793088525935 ) ) ;
#112531=CIRCLE ( 'NONE', #105541, 12.00000000000000178 ) ;
#112541=( BOUNDED_SURFACE ( )  B_SPLINE_SURFACE ( 3, 2, ( 
 ( #26810, #175225, #62511 ),
 ( #162166, #109214, #211949 ),
 ( #92912, #210886, #60376 ),
 ( #160023, #194645, #195724 ),
 ( #10553, #46287, #209814 ),
 ( #77696, #76627, #112404 ) ),
 .UNSPECIFIED., .F., .F., .T. ) 
 B_SPLINE_SURFACE_WITH_KNOTS ( ( 4, 2, 4 ),
 ( 3, 3 ),
 ( 1.843143693225357538E-18, 0.0009693014523152131655, 0.001938602904630424596 ),
 ( 0.000000000000000000, 1.000000000000000000 ),
 .UNSPECIFIED. ) 
 GEOMETRIC_REPRESENTATION_ITEM ( )  RATIONAL_B_SPLINE_SURFACE ( (
 ( 1.000000000000000000, 0.8462384754710218226, 1.000000000000000000),
 ( 1.000000000000000000, 0.8473855914980132908, 1.000000000000000000),
 ( 1.000000000000000000, 0.8490776175548976346, 1.000000000000000000),
 ( 1.000000000000000000, 0.8506485811854621604, 1.000000000000000000),
 ( 1.000000000000000000, 0.8507605089031664569, 1.000000000000000000),
 ( 1.000000000000000000, 0.8509629433967630385, 1.000000000000000000) ) ) 
 REPRESENTATION_ITEM ( '' )  SURFACE ( )  );
#112563=COLOUR_RGB ( '', 0.66274510, 0.83137255, 0.94901961) ;
#112613=CARTESIAN_POINT ( 'NONE',  ( -1.500000000000038636, 7.000000000000000000, -10.64483442802187874 ) ) ;
#112635=DIRECTION ( 'NONE',  ( 0.000000000000000000, 0.000000000000000000, -1.000000000000000000 ) ) ;
#112670=CARTESIAN_POINT ( 'NONE',  ( -11.89942855770814134, 11.29999999999999893, -0.7000000000000009548 ) ) ;
#112718=ORIENTED_EDGE ( 'NONE', *, *, #14697, .T. ) ;
#112726=CARTESIAN_POINT ( 'NONE',  ( 11.84103413958623818, 11.11004478473146229, 1.443924719788817423 ) ) ;
#112759=( NAMED_UNIT ( * ) PLANE_ANGLE_UNIT ( ) SI_UNIT ( $, .RADIAN. ) );
#112771=ORIENTED_EDGE ( 'NONE', *, *, #57003, .T. ) ;
#112775=PRESENTATION_STYLE_ASSIGNMENT (( #82316 ) ) ;
#112797=EDGE_LOOP ( 'NONE', ( #128249, #30017, #102654, #209249 ) ) ;
#112812=CARTESIAN_POINT ( 'NONE',  ( -10.50000000000000355, 12.59158320108480922, -3.600000000000000533 ) ) ;
#112837=ORIENTED_EDGE ( 'NONE', *, *, #74029, .T. ) ;
#112870=( LENGTH_UNIT ( ) NAMED_UNIT ( * ) SI_UNIT ( .MILLI., .METRE. ) );
#112880=EDGE_CURVE ( 'NONE', #142386, #204338, #128616, .T. ) ;
#112904=CARTESIAN_POINT ( 'NONE',  ( 11.89829993707161471, 9.770807717488739996, -1.561606677374349772 ) ) ;
#112917=ORIENTED_EDGE ( 'NONE', *, *, #170713, .F. ) ;
#112962=CARTESIAN_POINT ( 'NONE',  ( 11.52483635780546933, 11.37999991357535023, -3.345866325258015639 ) ) ;
#112978=( NAMED_UNIT ( * ) SI_UNIT ( $, .STERADIAN. ) SOLID_ANGLE_UNIT ( ) );
#112981=VERTEX_POINT ( 'NONE', #39581 ) ;
#112984=EDGE_CURVE ( 'NONE', #91093, #37173, #45672, .T. ) ;
#113008=VECTOR ( 'NONE', #49278, 1000.000000000000000 ) ;
#113019=DIRECTION ( 'NONE',  ( -0.000000000000000000, -1.000000000000000000, -0.000000000000000000 ) ) ;
#113021=FACE_OUTER_BOUND ( 'NONE', #86763, .T. ) ;
#113028=DIRECTION ( 'NONE',  ( 0.000000000000000000, -1.000000000000000000, -1.804652791718263484E-16 ) ) ;
#113029=ADVANCED_FACE ( 'NONE', ( #87267 ), #189030, .F. ) ;
#113034=EDGE_LOOP ( 'NONE', ( #187493, #134450, #90138, #62349 ) ) ;
#113035=CIRCLE ( 'NONE', #19551, 10.75000000000000000 ) ;
#113050=CARTESIAN_POINT ( 'NONE',  ( 11.39652004212136838, 9.097555222845741696, 6.605822843452838100 ) ) ;
#113064=DIRECTION ( 'NONE',  ( -0.000000000000000000, -1.000000000000000000, -0.000000000000000000 ) ) ;
#113067=CARTESIAN_POINT ( 'NONE',  ( 11.06298660227979802, 12.34319600374733383, -0.9087478855431304625 ) ) ;
#113094=AXIS2_PLACEMENT_3D ( 'NONE', #128344, #209468, #211607 ) ;
#113101=DIRECTION ( 'NONE',  ( -1.000000000000000000, 0.000000000000000000, 0.000000000000000000 ) ) ;
#113104=CARTESIAN_POINT ( 'NONE',  ( -11.35605497252127449, 13.61418145951644121, 3.553547709190206128 ) ) ;
#113105=EDGE_CURVE ( 'NONE', #182472, #108640, #66332, .T. ) ;
#113110=CARTESIAN_POINT ( 'NONE',  ( -1.249999999999964695, 8.500000000000000000, 11.02939254900287303 ) ) ;
#113145=CARTESIAN_POINT ( 'NONE',  ( 9.367496997597603681, 3.999999999999998224, -7.499999999999998224 ) ) ;
#113149=CARTESIAN_POINT ( 'NONE',  ( 10.03198553058017772, 14.16803135393298874, -7.469060636793986241 ) ) ;
#113152=CARTESIAN_POINT ( 'NONE',  ( 6.853823584984077399, 13.99925803066161478, 9.461486148285766618 ) ) ;
#113186=CARTESIAN_POINT ( 'NONE',  ( -11.50375155617990686, 6.427325993555151662, 3.051984382272954210 ) ) ;
#113199=PRESENTATION_STYLE_ASSIGNMENT (( #126264 ) ) ;
#113212=CARTESIAN_POINT ( 'NONE',  ( 11.90231137465227285, 7.647702690253872504, -1.097913969704247927 ) ) ;
#113232=AXIS2_PLACEMENT_3D ( 'NONE', #136307, #37725, #120115 ) ;
#113251=EDGE_CURVE ( 'NONE', #97972, #79300, #42713, .T. ) ;
#113263=CARTESIAN_POINT ( 'NONE',  ( -11.84101807917483740, 13.61021500260875428, 1.444039656437077879 ) ) ;
#113264=CARTESIAN_POINT ( 'NONE',  ( -11.95450533369660917, 8.100191672919370589, 0.5443015705738691867 ) ) ;
#113273=CARTESIAN_POINT ( 'NONE',  ( -10.79669699716785480, 6.389081389852535153, -5.150160299006881992 ) ) ;
#113303=CARTESIAN_POINT ( 'NONE',  ( -11.30309668167796922, 5.150585336095397260, -5.742054036728555744 ) ) ;
#113319=ORIENTED_EDGE ( 'NONE', *, *, #77746, .T. ) ;
#113323=CARTESIAN_POINT ( 'NONE',  ( -15.75000000000000000, 10.19999999999998153, 1.799999999999999600 ) ) ;
#113333=CARTESIAN_POINT ( 'NONE',  ( -7.789436271558764169, 15.44814005990453865, 9.080438957707684722 ) ) ;
#113374=AXIS2_PLACEMENT_3D ( 'NONE', #63821, #128904, #129979 ) ;
#113392=CARTESIAN_POINT ( 'NONE',  ( -11.91826848330638455, 13.50729645956978331, 1.400000080589927753 ) ) ;
#113412=FILL_AREA_STYLE ('',( #64587 ) ) ;
#113415=CARTESIAN_POINT ( 'NONE',  ( 11.07123322939518673, 11.29999999999999716, 0.8055995038523129370 ) ) ;
#113447=B_SPLINE_CURVE_WITH_KNOTS ( 'NONE', 3,
 ( #166255, #17844, #133795, #4777, #171583, #37316, #70855, #103391, #201918, #36238, #188898, #136969, #102316 ),
 .UNSPECIFIED., .F., .F.,
 ( 4, 3, 3, 3, 4 ),
 ( -1.794875636224401991E-06, 0.000000000000000000, 4.600594404842603212E-05, 8.489997069011644972E-05, 0.0001121994717586669222 ),
 .UNSPECIFIED. ) ;
#113463=CARTESIAN_POINT ( 'NONE',  ( 9.333041836227053523, 4.446947634372834912, 7.472413793103392265 ) ) ;
#113471=CARTESIAN_POINT ( 'NONE',  ( 8.836922018362429299, 13.05625752930196448, 8.050375269625257957 ) ) ;
#113492=VECTOR ( 'NONE', #156431, 1000.000000000000000 ) ;
#113506=LINE ( 'NONE', #148078, #10298 ) ;
#113560=CARTESIAN_POINT ( 'NONE',  ( 12.55138299807035551, 7.397854759914610057, -0.9335798560614338992 ) ) ;
#113563=EDGE_LOOP ( 'NONE', ( #23586, #136229, #89884 ) ) ;
#113570=CARTESIAN_POINT ( 'NONE',  ( 6.928203230275524760, 14.48154074412736847, -9.797958971132700867 ) ) ;
#113586=CARTESIAN_POINT ( 'NONE',  ( -11.89942855770814134, 13.88000000000000078, -0.7000000000000009548 ) ) ;
#113593=CARTESIAN_POINT ( 'NONE',  ( -9.495238110454886638, 15.17156879113547241, 7.231499654889550044 ) ) ;
#113666=CARTESIAN_POINT ( 'NONE',  ( 0.000000000000000000, 4.518459255872631530, 0.000000000000000000 ) ) ;
#113672=ORIENTED_EDGE ( 'NONE', *, *, #111152, .T. ) ;
#113683=CARTESIAN_POINT ( 'NONE',  ( 11.84101807917483740, 12.48978499739120629, 1.444039656437077657 ) ) ;
#113688=B_SPLINE_CURVE_WITH_KNOTS ( 'NONE', 3,
 ( #36332, #2748, #54729, #168478, #135991, #21126 ),
 .UNSPECIFIED., .F., .F.,
 ( 4, 2, 4 ),
 ( 0.001279092382393100377, 0.001599469101539997178, 0.001919845820686893979 ),
 .UNSPECIFIED. ) ;
#113692=DIRECTION ( 'NONE',  ( 0.000000000000000000, -1.000000000000000000, 0.000000000000000000 ) ) ;
#113706=( NAMED_UNIT ( * ) PLANE_ANGLE_UNIT ( ) SI_UNIT ( $, .RADIAN. ) );
#113720=DIRECTION ( 'NONE',  ( -0.000000000000000000, 1.000000000000000000, -0.000000000000000000 ) ) ;
#113728=CARTESIAN_POINT ( 'NONE',  ( 0.000000000000000000, 9.799999999999998934, 0.000000000000000000 ) ) ;
#113770=CARTESIAN_POINT ( 'NONE',  ( 6.902720145100436078, 14.55347103577509138, 9.761920446467003742 ) ) ;
#113810=EDGE_CURVE ( 'NONE', #155586, #144610, #143170, .T. ) ;
#113813=CARTESIAN_POINT ( 'NONE',  ( 11.84668730067608244, 10.19999999999999929, -1.400000000000001688 ) ) ;
#113819=EDGE_CURVE ( 'NONE', #60282, #93441, #18484, .T. ) ;
#113830=VECTOR ( 'NONE', #107058, 1000.000000000000000 ) ;
#113831=CARTESIAN_POINT ( 'NONE',  ( -9.340702556249551591, 14.55305236562982607, 7.462845556860540519 ) ) ;
#113861=CARTESIAN_POINT ( 'NONE',  ( -11.86161086955307198, 8.823445149503903906, 1.515882294691715204 ) ) ;
#113902=CYLINDRICAL_SURFACE ( 'NONE', #71942, 0.07999999999999998779 ) ;
#113927=CARTESIAN_POINT ( 'NONE',  ( 0.000000000000000000, 15.00000000000000000, -12.18000000000000149 ) ) ;
#113930=CARTESIAN_POINT ( 'NONE',  ( -11.88234649872613602, 13.75660782916751579, -0.9090484974825174813 ) ) ;
#113936=B_SPLINE_CURVE_WITH_KNOTS ( 'NONE', 3,
 ( #87033, #36137, #4680, #182383, #167226, #17735 ),
 .UNSPECIFIED., .F., .F.,
 ( 4, 2, 4 ),
 ( 0.000000000000000000, 0.0003157158648874031190, 0.0006314317297748062380 ),
 .UNSPECIFIED. ) ;
#113942=FILL_AREA_STYLE ('',( #46759 ) ) ;
#113953=VERTEX_POINT ( 'NONE', #183342 ) ;
#113975=CARTESIAN_POINT ( 'NONE',  ( 11.92619526913699879, 10.19999999999999929, -1.328859060402686199 ) ) ;
#113995=ORIENTED_EDGE ( 'NONE', *, *, #101713, .F. ) ;
#114009=CYLINDRICAL_SURFACE ( 'NONE', #103430, 0.07999999999999998779 ) ;
#114034=CARTESIAN_POINT ( 'NONE',  ( 11.06305611892948448, 13.75761539554391533, 0.9079708613958296093 ) ) ;
#114042=FACE_OUTER_BOUND ( 'NONE', #97492, .T. ) ;
#114079=CARTESIAN_POINT ( 'NONE',  ( 0.01291931824900593301, 14.54921173327639217, 11.96434918058137242 ) ) ;
#114086=ADVANCED_FACE ( 'NONE', ( #166033 ), #135678, .F. ) ;
#114103=CARTESIAN_POINT ( 'NONE',  ( -11.07790593930098311, 13.79999999999999893, 0.6999999999999992895 ) ) ;
#114124=CARTESIAN_POINT ( 'NONE',  ( 9.542125166518260926, 12.19240180423196485, 8.745854086120228743 ) ) ;
#114127=ORIENTED_EDGE ( 'NONE', *, *, #510, .T. ) ;
#114152=DIRECTION ( 'NONE',  ( 1.000000000000000000, -0.000000000000000000, -0.000000000000000000 ) ) ;
#114178=CARTESIAN_POINT ( 'NONE',  ( -11.82533409993242834, 7.631798484810768279, 2.053971879869906036 ) ) ;
#114197=DIRECTION ( 'NONE',  ( 0.000000000000000000, 0.000000000000000000, 1.000000000000000000 ) ) ;
#114219=CARTESIAN_POINT ( 'NONE',  ( 6.743451144134844810, 16.00000000000000000, -9.536680065235829673 ) ) ;
#114222=CARTESIAN_POINT ( 'NONE',  ( 8.344038675336102884, 13.15493340621088336, 8.539968482448076159 ) ) ;
#114243=STYLED_ITEM ( 'NONE', ( #212687 ), #24096 ) ;
#114254=CARTESIAN_POINT ( 'NONE',  ( -10.90754186426655004, 4.636108433425617292, 4.485516275142084730 ) ) ;
#114273=CARTESIAN_POINT ( 'NONE',  ( -9.434262096661420571, 14.57949301904344885, 7.415936068925672586 ) ) ;
#114282=CARTESIAN_POINT ( 'NONE',  ( 11.09214416354366861, 9.059100286490975762, -4.456786335284255607 ) ) ;
#114293=DIRECTION ( 'NONE',  ( 0.000000000000000000, 0.000000000000000000, 1.000000000000000000 ) ) ;
#114309=CARTESIAN_POINT ( 'NONE',  ( 10.95308175811721085, 13.79999999999998295, 1.799999999999999600 ) ) ;
#114324=FILL_AREA_STYLE ('',( #134792 ) ) ;
#114329=CARTESIAN_POINT ( 'NONE',  ( -11.95656167602934161, 7.981505742835744321, -1.053473157398042037 ) ) ;
#114338=CARTESIAN_POINT ( 'NONE',  ( -11.81223854822482622, 8.717195842676252582, -2.135728645746848287 ) ) ;
#114349=ORIENTED_EDGE ( 'NONE', *, *, #24376, .F. ) ;
#114357=ADVANCED_FACE ( 'NONE', ( #9924 ), #56545, .T. ) ;
#114382=ORIENTED_EDGE ( 'NONE', *, *, #94657, .F. ) ;
#114387=LINE ( 'NONE', #80755, #62812 ) ;
#114393=CARTESIAN_POINT ( 'NONE',  ( 11.86145016429272836, 10.19999999999999929, 1.179999999999997051 ) ) ;
#114394=CARTESIAN_POINT ( 'NONE',  ( -11.04536101718726293, 13.40000000000000036, -1.100000000000002087 ) ) ;
#114427=( LENGTH_UNIT ( ) NAMED_UNIT ( * ) SI_UNIT ( .MILLI., .METRE. ) );
#114476=B_SPLINE_CURVE_WITH_KNOTS ( 'NONE', 3,
 ( #201626, #119406, #98841, #167032, #17543, #1295 ),
 .UNSPECIFIED., .F., .F.,
 ( 4, 2, 4 ),
 ( 0.000000000000000000, 0.0003155923098472862933, 0.0006311846196945722614 ),
 .UNSPECIFIED. ) ;
#114498=EDGE_CURVE ( 'NONE', #204806, #158047, #7776, .T. ) ;
#114501=FACE_OUTER_BOUND ( 'NONE', #200056, .T. ) ;
#114530=DIRECTION ( 'NONE',  ( 0.000000000000000000, 0.000000000000000000, -1.000000000000000000 ) ) ;
#114532=DIRECTION ( 'NONE',  ( 0.000000000000000000, -1.000000000000000000, -0.000000000000000000 ) ) ;
#114540=CARTESIAN_POINT ( 'NONE',  ( -11.01135777277262129, 10.19999999999999929, -1.400000000000001910 ) ) ;
#114547=CIRCLE ( 'NONE', #104122, 11.67999999982603576 ) ;
#114582=CARTESIAN_POINT ( 'NONE',  ( 11.04536101718726293, 10.90000000000000036, 1.099999999999996758 ) ) ;
#114590=ORIENTED_EDGE ( 'NONE', *, *, #120681, .T. ) ;
#114593=ORIENTED_EDGE ( 'NONE', *, *, #210514, .T. ) ;
#114599=CARTESIAN_POINT ( 'NONE',  ( -10.43233925736708301, 5.066585305077033752, -5.254699789447807134 ) ) ;
#114607=CARTESIAN_POINT ( 'NONE',  ( -11.97929049433705373, 13.88000000000000078, -0.7046979865771834106 ) ) ;
#114622=CARTESIAN_POINT ( 'NONE',  ( 9.266412064734856457, 13.60091921773422641, 6.823019651404623964 ) ) ;
#114633=CARTESIAN_POINT ( 'NONE',  ( 8.116463737798994771, 14.26148076985399982, -8.779171398687106276 ) ) ;
#114656=CARTESIAN_POINT ( 'NONE',  ( -9.445420027513430128, 14.68120331434907300, 7.300025634049736922 ) ) ;
#114680=COLOUR_RGB ( '', 0.08235294, 0.09019608, 0.10196078) ;
#114736=FACE_OUTER_BOUND ( 'NONE', #75150, .T. ) ;
#114749=ORIENTED_EDGE ( 'NONE', *, *, #55036, .T. ) ;
#114834=AXIS2_PLACEMENT_3D ( 'NONE', #134552, #197375, #148644 ) ;
#114879=( GEOMETRIC_REPRESENTATION_CONTEXT ( 3 ) GLOBAL_UNCERTAINTY_ASSIGNED_CONTEXT ( ( #144821 ) ) GLOBAL_UNIT_ASSIGNED_CONTEXT ( ( #173998, #27715, #125301 ) ) REPRESENTATION_CONTEXT ( 'NONE', 'WORKASPACE' ) );
#114883=DIRECTION ( 'NONE',  ( 3.706092522800016599E-15, 0.000000000000000000, 1.000000000000000000 ) ) ;
#114890=DIRECTION ( 'NONE',  ( -0.000000000000000000, 1.000000000000000000, -0.000000000000000000 ) ) ;
#114896=EDGE_CURVE ( 'NONE', #120419, #24390, #136775, .T. ) ;
#114908=CARTESIAN_POINT ( 'NONE',  ( -11.95482906247546850, 9.001069635099803179, -0.6096848022493118746 ) ) ;
#114916=CARTESIAN_POINT ( 'NONE',  ( 1.250000000000037526, 8.500000000000000000, -11.02939254900286592 ) ) ;
#114917=VERTEX_POINT ( 'NONE', #99998 ) ;
#114926=SURFACE_SIDE_STYLE ('',( #67145 ) ) ;
#114949=ORIENTED_EDGE ( 'NONE', *, *, #131308, .T. ) ;
#114955=CARTESIAN_POINT ( 'NONE',  ( -9.705102360090382518, 4.469090025550438661, -7.059677490138621891 ) ) ;
#114976=CARTESIAN_POINT ( 'NONE',  ( -11.86685672517501899, 13.60918917859810584, -1.056525322636018727 ) ) ;
#114980=VECTOR ( 'NONE', #148251, 1000.000000000000000 ) ;
#114991=FACE_OUTER_BOUND ( 'NONE', #66895, .T. ) ;
#115007=ADVANCED_FACE ( 'NONE', ( #173565 ), #57655, .F. ) ;
#115026=CARTESIAN_POINT ( 'NONE',  ( 10.97030574691034843, 11.30000000000000249, -1.695191245859933193 ) ) ;
#115034=VERTEX_POINT ( 'NONE', #189775 ) ;
#115046=EDGE_LOOP ( 'NONE', ( #51163, #56902, #52783, #79562, #157094 ) ) ;
#115059=CARTESIAN_POINT ( 'NONE',  ( 11.86687934130374522, 9.990480503834419324, 1.056332641424306606 ) ) ;
#115079=VERTEX_POINT ( 'NONE', #8889 ) ;
#115113=FACE_BOUND ( 'NONE', #92889, .T. ) ;
#115117=ORIENTED_EDGE ( 'NONE', *, *, #53950, .F. ) ;
#115148=VECTOR ( 'NONE', #36829, 1000.000000000000000 ) ;
#115152=CIRCLE ( 'NONE', #21647, 12.00000000000000178 ) ;
#115157=CARTESIAN_POINT ( 'NONE',  ( -11.91826848330605593, 10.09270354043010798, -1.400000080589192120 ) ) ;
#115164=SURFACE_STYLE_USAGE ( .BOTH. , #162798 ) ;
#115176=CARTESIAN_POINT ( 'NONE',  ( 9.235375178776246585, 13.16128858080087660, -9.014701623559966848 ) ) ;
#115190=AXIS2_PLACEMENT_3D ( 'NONE', #185673, #182473, #37302 ) ;
#115215=CARTESIAN_POINT ( 'NONE',  ( 11.41157692552970815, 9.840896629130003959, -3.404533818002362100 ) ) ;
#115229=DIRECTION ( 'NONE',  ( 0.000000000000000000, 0.000000000000000000, -1.000000000000000000 ) ) ;
#115233=FACE_OUTER_BOUND ( 'NONE', #61360, .T. ) ;
#115273=CARTESIAN_POINT ( 'NONE',  ( 9.258966325506417405, 13.63624071251986258, -6.830021722722439570 ) ) ;
#115308=CARTESIAN_POINT ( 'NONE',  ( -11.78041000490145862, 4.728159582424554586, -4.968671142906706528 ) ) ;
#115312=CARTESIAN_POINT ( 'NONE',  ( 8.857846419285928974, 14.66713266182295250, -8.029988375369475406 ) ) ;
#115316=B_SPLINE_CURVE_WITH_KNOTS ( 'NONE', 3,
 ( #107574, #77131, #193005, #190871, #42536, #108639 ),
 .UNSPECIFIED., .F., .F.,
 ( 4, 2, 4 ),
 ( 0.000000000000000000, 0.0003778774010236168619, 0.0007557548020472337237 ),
 .UNSPECIFIED. ) ;
#115329=CARTESIAN_POINT ( 'NONE',  ( -9.523390464710169923, 14.62238631451544713, 7.301111590532052276 ) ) ;
#115330=VERTEX_POINT ( 'NONE', #37942 ) ;
#115345=CARTESIAN_POINT ( 'NONE',  ( 8.744138462177931004, 13.53963283848627697, -8.151542665958993794 ) ) ;
#115350=CARTESIAN_POINT ( 'NONE',  ( 11.88156762547253997, 12.22000008454031672, -1.686557021358706443 ) ) ;
#115363=CIRCLE ( 'NONE', #143013, 11.09999999999999964 ) ;
#115382=SURFACE_SIDE_STYLE ('',( #98026 ) ) ;
#115387=CARTESIAN_POINT ( 'NONE',  ( -11.57172163803348575, 7.019044685052739929, -3.185222216268118522 ) ) ;
#115396=CARTESIAN_POINT ( 'NONE',  ( -12.00000795471044945, 9.073126563016209900, 0.3090979129135709158 ) ) ;
#115424=ORIENTED_EDGE ( 'NONE', *, *, #197258, .T. ) ;
#115440=FACE_OUTER_BOUND ( 'NONE', #47603, .T. ) ;
#115442=AXIS2_PLACEMENT_3D ( 'NONE', #103451, #20045, #22155 ) ;
#115444=CARTESIAN_POINT ( 'NONE',  ( 11.49978884755361008, 13.74270821162803990, -3.429452816445331731 ) ) ;
#115447=COLOUR_RGB ( '', 0.72549020, 0.75294118, 0.79215686) ;
#115502=VERTEX_POINT ( 'NONE', #3274 ) ;
#115506=CARTESIAN_POINT ( 'NONE',  ( 11.89942855770814312, 11.37999999999999901, 0.6999999999999992895 ) ) ;
#115551=CARTESIAN_POINT ( 'NONE',  ( 1.050790385994986975, 15.00000000000000711, -12.64745918785790835 ) ) ;
#115572=ORIENTED_EDGE ( 'NONE', *, *, #183072, .T. ) ;
#115579=UNCERTAINTY_MEASURE_WITH_UNIT (LENGTH_MEASURE( 1.000000000000000082E-05 ), #162627, 'distance_accuracy_value', 'NONE');
#115635=ORIENTED_EDGE ( 'NONE', *, *, #169884, .T. ) ;
#115645=CARTESIAN_POINT ( 'NONE',  ( 11.97929049433705373, 11.37999999999999901, 0.7046979865771783036 ) ) ;
#115646=CARTESIAN_POINT ( 'NONE',  ( -10.82993273518205690, 5.589502548902120616, -6.507125152095314391 ) ) ;
#115664=CARTESIAN_POINT ( 'NONE',  ( 8.991265305961727350, 12.32808046726238516, -7.950307984862021726 ) ) ;
#115672=CARTESIAN_POINT ( 'NONE',  ( 9.281908132336914363, 13.38402037623112939, -6.770111635749896273 ) ) ;
#115684=CARTESIAN_POINT ( 'NONE',  ( 7.127625674359589603, 14.48154076733629303, -9.656946008600062470 ) ) ;
#115718=CARTESIAN_POINT ( 'NONE',  ( -9.497986836791788789, 15.41982400883598459, -7.334206419346871009 ) ) ;
#115728=CYLINDRICAL_SURFACE ( 'NONE', #134307, 0.07999999999999998779 ) ;
#115733=( BOUNDED_SURFACE ( )  B_SPLINE_SURFACE ( 3, 2, ( 
 ( #162753, #80417, #146515 ),
 ( #212534, #64174, #108717 ),
 ( #158470, #81485, #83603 ),
 ( #197354, #150764, #198408 ),
 ( #50052, #183239, #85742 ),
 ( #3399, #16455, #67325 ) ),
 .UNSPECIFIED., .F., .F., .T. ) 
 B_SPLINE_SURFACE_WITH_KNOTS ( ( 4, 2, 4 ),
 ( 3, 3 ),
 ( 0.000000000000000000, 0.0003754689591423961527, 0.0007509379182847923054 ),
 ( 0.000000000000000000, 1.000000000000000000 ),
 .UNSPECIFIED. ) 
 GEOMETRIC_REPRESENTATION_ITEM ( )  RATIONAL_B_SPLINE_SURFACE ( (
 ( 1.000000000000000000, 0.7071067811865551223, 1.000000000000000000),
 ( 1.000000000000000000, 0.7018599272026838642, 1.000000000000000000),
 ( 1.000000000000000000, 0.6927733177256477637, 1.000000000000000000),
 ( 1.000000000000000000, 0.6772007068877506919, 1.000000000000000000),
 ( 1.000000000000000000, 0.6709974581634180479, 1.000000000000000000),
 ( 1.000000000000000000, 0.6711954675835484219, 1.000000000000000000) ) ) 
 REPRESENTATION_ITEM ( '' )  SURFACE ( )  );
#115829=AXIS2_PLACEMENT_3D ( 'NONE', #209952, #127760, #174304 ) ;
#115835=SURFACE_STYLE_FILL_AREA ( #15049 ) ;
#115857=CARTESIAN_POINT ( 'NONE',  ( 11.43195036480943116, 11.15524496285256006, 3.649565797774380727 ) ) ;
#115886=CARTESIAN_POINT ( 'NONE',  ( 8.809690371089210714, 13.28836970969089748, 8.148114100277194183 ) ) ;
#115903=ORIENTED_EDGE ( 'NONE', *, *, #87595, .T. ) ;
#115908=ORIENTED_EDGE ( 'NONE', *, *, #831, .T. ) ;
#115925=CARTESIAN_POINT ( 'NONE',  ( 11.92050416151432835, 9.947946247203756087, -1.381922468431410866 ) ) ;
#115934=CARTESIAN_POINT ( 'NONE',  ( -11.55950211276791428, 12.21999999999998288, 3.221476510067114329 ) ) ;
#115939=ORIENTED_EDGE ( 'NONE', *, *, #60516, .T. ) ;
#115953=FILL_AREA_STYLE_COLOUR ( '', #55822 ) ;
#115961=LINE ( 'NONE', #1053, #53799 ) ;
#116003=CARTESIAN_POINT ( 'NONE',  ( 1.386567914617388375, 8.090296256147718523, -10.72428812184712932 ) ) ;
#116022=AXIS2_PLACEMENT_3D ( 'NONE', #21332, #87438, #71151 ) ;
#116081=CARTESIAN_POINT ( 'NONE',  ( -9.587704862635016312, 4.026159954882873926, 6.671158199369250141 ) ) ;
#116089=EDGE_LOOP ( 'NONE', ( #199034, #149488, #69936, #196119 ) ) ;
#116100=VERTEX_POINT ( 'NONE', #8628 ) ;
#116113=EDGE_CURVE ( 'NONE', #84148, #213513, #67165, .T. ) ;
#116117=AXIS2_PLACEMENT_3D ( 'NONE', #130113, #164659, #144199 ) ;
#116123=B_SPLINE_CURVE_WITH_KNOTS ( 'NONE', 3,
 ( #88844, #174367, #141884, #72561, #40084, #138659 ),
 .UNSPECIFIED., .F., .F.,
 ( 4, 2, 4 ),
 ( 0.000000000000000000, 0.0003778774010236168076, 0.0007557548020472336153 ),
 .UNSPECIFIED. ) ;
#116139=CARTESIAN_POINT ( 'NONE',  ( -10.79323443277434791, 4.699918835924045801, -5.141973237006214781 ) ) ;
#116142=DIRECTION ( 'NONE',  ( 1.000000000000000000, -0.000000000000000000, 1.224646799147353207E-16 ) ) ;
#116144=CARTESIAN_POINT ( 'NONE',  ( 11.81911962874431055, 12.34289426515882759, 1.591749704452489533 ) ) ;
#116165=VERTEX_POINT ( 'NONE', #187380 ) ;
#116172=CARTESIAN_POINT ( 'NONE',  ( -4.778319401024116786, 15.44696626029461939, -10.96850100116969351 ) ) ;
#116224=CARTESIAN_POINT ( 'NONE',  ( 11.35610322553117513, 13.61421628929173266, 3.553412924323500643 ) ) ;
#116236=CARTESIAN_POINT ( 'NONE',  ( 9.710969956560674632, 13.29837910982962690, -8.127984515541683663 ) ) ;
#116247=DIRECTION ( 'NONE',  ( -0.000000000000000000, 1.000000000000000000, 9.023263958591317418E-17 ) ) ;
#116248=VERTEX_POINT ( 'NONE', #95247 ) ;
#116254=CARTESIAN_POINT ( 'NONE',  ( 0.000000000000000000, 18.91999999999999815, 11.09999999999999964 ) ) ;
#116333=CARTESIAN_POINT ( 'NONE',  ( 8.305220197644215929, 14.86737089724833893, -9.585679967850639471 ) ) ;
#116351=CARTESIAN_POINT ( 'NONE',  ( 11.96217875511318063, 13.82854366578976624, -0.9561995067075083066 ) ) ;
#116367=ADVANCED_FACE ( 'NONE', ( #110475 ), #192699, .T. ) ;
#116384=CARTESIAN_POINT ( 'NONE',  ( -9.393996029772727852, 15.45879393270864099, 7.466831081026168881 ) ) ;
#116391=CARTESIAN_POINT ( 'NONE',  ( 9.978696604288037619, 11.55417434068213822, -6.670641654589029912 ) ) ;
#116397=VERTEX_POINT ( 'NONE', #180731 ) ;
#116400=CARTESIAN_POINT ( 'NONE',  ( -10.62873463776380234, 12.29999999999998295, 3.199999999999997957 ) ) ;
#116428=ADVANCED_FACE ( 'NONE', ( #194848 ), #39516, .T. ) ;
#116451=LINE ( 'NONE', #34072, #113008 ) ;
#116467=CARTESIAN_POINT ( 'NONE',  ( -11.97181042169641962, 9.720000000000002416, -0.8318531151397202672 ) ) ;
#116468=DIRECTION ( 'NONE',  ( 1.000000000000000000, -0.000000000000000000, -0.000000000000000000 ) ) ;
#116556=( NAMED_UNIT ( * ) SI_UNIT ( $, .STERADIAN. ) SOLID_ANGLE_UNIT ( ) );
#116584=( NAMED_UNIT ( * ) PLANE_ANGLE_UNIT ( ) SI_UNIT ( $, .RADIAN. ) );
#116617=CARTESIAN_POINT ( 'NONE',  ( -10.88586298614011660, 5.812970821470938354, 6.395187734525825896 ) ) ;
#116647=LINE ( 'NONE', #202063, #158903 ) ;
#116688=MECHANICAL_DESIGN_GEOMETRIC_PRESENTATION_REPRESENTATION('',(#19829),#64679);
#116713=CARTESIAN_POINT ( 'NONE',  ( -9.409940793360268785, 3.999985931113709814, -6.919963696468023784 ) ) ;
#116723=CARTESIAN_POINT ( 'NONE',  ( -10.45911050446410506, 5.175404930453152197, 5.201426885097844455 ) ) ;
#116729=CARTESIAN_POINT ( 'NONE',  ( 10.91919020434494136, 8.223964437691744678, -4.993264204099808090 ) ) ;
#116734=EDGE_LOOP ( 'NONE', ( #14927, #176490, #124387, #193006 ) ) ;
#116742=CARTESIAN_POINT ( 'NONE',  ( 11.05419992680906027, 7.768390597564347466, 1.622890935638873655 ) ) ;
#116753=CARTESIAN_POINT ( 'NONE',  ( 7.695155468110882246, 14.38165973575666179, -9.208594225262938693 ) ) ;
#116755=ORIENTED_EDGE ( 'NONE', *, *, #125943, .F. ) ;
#116768=CARTESIAN_POINT ( 'NONE',  ( -11.86239285000045918, 11.37999999999999901, -1.812080536912752837 ) ) ;
#116854=CIRCLE ( 'NONE', #144525, 0.07999999999999946043 ) ;
#116866=CARTESIAN_POINT ( 'NONE',  ( 11.41126283316774348, 12.34125393091539280, 3.405403429622879230 ) ) ;
#116887=CARTESIAN_POINT ( 'NONE',  ( -11.33772463945037146, 10.89999999999998259, 3.679999999999999272 ) ) ;
#116909=CARTESIAN_POINT ( 'NONE',  ( -9.495441445486415333, 15.17076627066290229, -7.231220947886418671 ) ) ;
#116913=EDGE_LOOP ( 'NONE', ( #86852, #158912, #34659, #206099 ) ) ;
#116945=FACE_OUTER_BOUND ( 'NONE', #103606, .T. ) ;
#116968=CIRCLE ( 'NONE', #137802, 0.07999999999999940492 ) ;
#116972=VERTEX_POINT ( 'NONE', #209403 ) ;
#116990=CARTESIAN_POINT ( 'NONE',  ( 11.84103413958613160, 9.989955215268565780, -1.443924719788771682 ) ) ;
#117004=EDGE_LOOP ( 'NONE', ( #145416, #201101, #72759, #186813 ) ) ;
#117006=CARTESIAN_POINT ( 'NONE',  ( 7.637366960813559480, 15.45595454679949832, 9.257485277755282738 ) ) ;
#117008=CARTESIAN_POINT ( 'NONE',  ( -10.33392256004288079, 4.765625372279607141, 5.445010993851796322 ) ) ;
#117023=CARTESIAN_POINT ( 'NONE',  ( -11.52483635780546578, 11.37999991357544438, 3.345866325258016083 ) ) ;
#117032=DIRECTION ( 'NONE',  ( 0.000000000000000000, 0.000000000000000000, -1.000000000000000000 ) ) ;
#117055=DIRECTION ( 'NONE',  ( 0.000000000000000000, 0.000000000000000000, -1.000000000000000000 ) ) ;
#117065=AXIS2_PLACEMENT_3D ( 'NONE', #109310, #111436, #110373 ) ;
#117068=CARTESIAN_POINT ( 'NONE',  ( 1.499999999999961364, 7.750000000000000000, -10.64483442802188762 ) ) ;
#117071=( GEOMETRIC_REPRESENTATION_CONTEXT ( 3 ) GLOBAL_UNCERTAINTY_ASSIGNED_CONTEXT ( ( #213258 ) ) GLOBAL_UNIT_ASSIGNED_CONTEXT ( ( #16782, #82866, #195571 ) ) REPRESENTATION_CONTEXT ( 'NONE', 'WORKASPACE' ) );
#117081=VERTEX_POINT ( 'NONE', #44825 ) ;
#117094=CARTESIAN_POINT ( 'NONE',  ( -11.55950211276791073, 12.30000000000000071, -3.221476510067115662 ) ) ;
#117102=COLOUR_RGB ( '', 0.72549020, 0.75294118, 0.79215686) ;
#117119=FACE_OUTER_BOUND ( 'NONE', #67896, .T. ) ;
#117185=CARTESIAN_POINT ( 'NONE',  ( -9.437944175038655459, 15.48612576208931735, -7.411204044582823336 ) ) ;
#117214=CARTESIAN_POINT ( 'NONE',  ( 1.469576158976824144E-15, 19.00000000000000000, 12.00000000000000178 ) ) ;
#117248=B_SPLINE_CURVE_WITH_KNOTS ( 'NONE', 3,
 ( #42541, #71780, #174672, #38244, #158401, #170368 ),
 .UNSPECIFIED., .F., .F.,
 ( 4, 2, 4 ),
 ( 0.000000000000000000, 0.0003845013059668467856, 0.0007690026119336935712 ),
 .UNSPECIFIED. ) ;
#117249=EDGE_LOOP ( 'NONE', ( #173220, #204371, #24504, #151828 ) ) ;
#117269=DIRECTION ( 'NONE',  ( 0.000000000000000000, -1.000000000000000000, 0.000000000000000000 ) ) ;
#117271=CARTESIAN_POINT ( 'NONE',  ( 11.41381675112453031, 10.19999999999999929, -3.704697986577182078 ) ) ;
#117274=EDGE_LOOP ( 'NONE', ( #155133, #76149, #60230, #79907 ) ) ;
#117276=ORIENTED_EDGE ( 'NONE', *, *, #2431, .T. ) ;
#117283=AXIS2_PLACEMENT_3D ( 'NONE', #209075, #176609, #11958 ) ;
#117286=ORIENTED_EDGE ( 'NONE', *, *, #178754, .T. ) ;
#117291=CARTESIAN_POINT ( 'NONE',  ( -12.04274103669372309, 7.374159847806027734, 3.963224530603232765 ) ) ;
#117292=CARTESIAN_POINT ( 'NONE',  ( 11.48243876534946217, 13.87999999999998302, 3.199999999999997957 ) ) ;
#117293=CARTESIAN_POINT ( 'NONE',  ( -15.75000000000000000, 12.30000000000000071, -0.7000000000000009548 ) ) ;
#117304=ORIENTED_EDGE ( 'NONE', *, *, #47755, .T. ) ;
#117313=DIRECTION ( 'NONE',  ( 0.000000000000000000, -9.023263958591318651E-17, 1.000000000000000000 ) ) ;
#117319=CARTESIAN_POINT ( 'NONE',  ( -11.86239285000045918, 11.37999999999998302, 1.812080536912751061 ) ) ;
#117333=EDGE_CURVE ( 'NONE', #66261, #59479, #171089, .T. ) ;
#117335=VECTOR ( 'NONE', #127203, 1000.000000000000000 ) ;
#117349=ORIENTED_EDGE ( 'NONE', *, *, #193907, .F. ) ;
#117355=CARTESIAN_POINT ( 'NONE',  ( -9.510997388311002609, 3.006837337344905325, -6.782141846552069531 ) ) ;
#117360=CARTESIAN_POINT ( 'NONE',  ( -11.73399103866650073, 7.418623464565952119, 2.524040681687853560 ) ) ;
#117363=EDGE_CURVE ( 'NONE', #132416, #94694, #178067, .T. ) ;
#117407=CARTESIAN_POINT ( 'NONE',  ( 8.344868292979940705, 13.15147191686607364, -8.540160728547430580 ) ) ;
#117413=ORIENTED_EDGE ( 'NONE', *, *, #53950, .T. ) ;
#117439=CONICAL_SURFACE ( 'NONE', #6651, 10.75000000000000000, 0.5235987755983064762 ) ;
#117459=EDGE_LOOP ( 'NONE', ( #126737, #213397, #36950, #25174 ) ) ;
#117464=CARTESIAN_POINT ( 'NONE',  ( 1.423205080756849483, 7.980384757729337863, -10.65537363484302524 ) ) ;
#117477=ORIENTED_EDGE ( 'NONE', *, *, #154446, .T. ) ;
#117479=AXIS2_PLACEMENT_3D ( 'NONE', #201447, #18449, #5373 ) ;
#117525=SURFACE_STYLE_FILL_AREA ( #184577 ) ;
#117539=LINE ( 'NONE', #165159, #162976 ) ;
#117556=ORIENTED_EDGE ( 'NONE', *, *, #24376, .T. ) ;
#117565=EDGE_CURVE ( 'NONE', #197638, #74053, #140796, .T. ) ;
#117643=DIRECTION ( 'NONE',  ( 0.000000000000000000, -1.000000000000000000, -0.000000000000000000 ) ) ;
#117680=EDGE_CURVE ( 'NONE', #40498, #29327, #5602, .T. ) ;
#117693=CARTESIAN_POINT ( 'NONE',  ( -6.671583288098391407, 15.00000000000335731, -9.747470831326879193 ) ) ;
#117695=CARTESIAN_POINT ( 'NONE',  ( -10.52284260640670688, 5.420240069097000735, -5.071998063130033430 ) ) ;
#117717=ORIENTED_EDGE ( 'NONE', *, *, #37600, .F. ) ;
#117744=TOROIDAL_SURFACE ( 'NONE', #3534, 11.92000000000000171, 0.08000000000000000167 ) ;
#117766=CARTESIAN_POINT ( 'NONE',  ( 11.97178994924802353, 9.720000062027946086, -0.8322011300497146324 ) ) ;
#117790=VERTEX_POINT ( 'NONE', #105302 ) ;
#117795=CARTESIAN_POINT ( 'NONE',  ( -10.48363756508902611, 5.078564944783316548, -7.119907325005036647 ) ) ;
#117813=CARTESIAN_POINT ( 'NONE',  ( 10.92756393739431076, 8.276992061150025393, 4.974981638007045959 ) ) ;
#117825=CARTESIAN_POINT ( 'NONE',  ( 10.27857769538790933, 8.980592535482619709, 4.146738271564137435 ) ) ;
#117834=CARTESIAN_POINT ( 'NONE',  ( 7.602957498476571097, 14.40772565114494341, -9.284908058097229855 ) ) ;
#117835=CARTESIAN_POINT ( 'NONE',  ( -6.748594069003817530, 15.46991018063243928, -9.932583631540687463 ) ) ;
#117836=ORIENTED_EDGE ( 'NONE', *, *, #31880, .T. ) ;
#117837=EDGE_CURVE ( 'NONE', #47238, #59570, #85827, .T. ) ;
#117874=MECHANICAL_DESIGN_GEOMETRIC_PRESENTATION_REPRESENTATION('',(#183515),#69392);
#117905=( LENGTH_UNIT ( ) NAMED_UNIT ( * ) SI_UNIT ( .MILLI., .METRE. ) );
#117940=CIRCLE ( 'NONE', #204429, 0.08000000000000069555 ) ;
#117943=CARTESIAN_POINT ( 'NONE',  ( 11.48243876534946217, 12.29999999999998295, 3.199999999999997957 ) ) ;
#117977=EDGE_CURVE ( 'NONE', #56620, #198793, #89049, .T. ) ;
#117993=FILL_AREA_STYLE ('',( #200222 ) ) ;
#117995=CARTESIAN_POINT ( 'NONE',  ( -11.89942855770814134, 9.799999999999998934, 0.6999999999999992895 ) ) ;
#118001=CARTESIAN_POINT ( 'NONE',  ( -0.008622031262367491067, 15.44736672593548299, 11.95585889282746450 ) ) ;
#118024=CARTESIAN_POINT ( 'NONE',  ( 8.790098660144264997, 13.29414747594432278, 8.101455065885629026 ) ) ;
#118029=COLOUR_RGB ( '', 0.31764706, 0.68627451, 0.89019608) ;
#118044=VERTEX_POINT ( 'NONE', #72766 ) ;
#118065=CARTESIAN_POINT ( 'NONE',  ( 11.84668729410392274, 10.09379487675467146, -1.400000000000001688 ) ) ;
#118080=CARTESIAN_POINT ( 'NONE',  ( 9.175356366548005127, 14.33556514466065757, 7.734832780443797517 ) ) ;
#118082=CARTESIAN_POINT ( 'NONE',  ( -9.911963570431085557, 5.384551446482307213, 6.114068938207696036 ) ) ;
#118093=CIRCLE ( 'NONE', #7450, 11.92000000000000171 ) ;
#118100=CARTESIAN_POINT ( 'NONE',  ( 11.48243876534946217, 12.29999999999998295, 3.199999999999997957 ) ) ;
#118132=DIRECTION ( 'NONE',  ( 1.000000000000000000, 0.000000000000000000, -0.000000000000000000 ) ) ;
#118148=CIRCLE ( 'NONE', #169871, 11.09999999999999964 ) ;
#118159=CARTESIAN_POINT ( 'NONE',  ( -10.91033920341459051, 4.885615726745599297, 4.996448585388897357 ) ) ;
#118162=CARTESIAN_POINT ( 'NONE',  ( -11.84668730067608244, 13.50636224908218885, -1.400000000000002132 ) ) ;
#118166=CARTESIAN_POINT ( 'NONE',  ( -11.44800751629991353, 12.30000000000000071, -3.302956944461114652 ) ) ;
#118190=FILL_AREA_STYLE ('',( #35798 ) ) ;
#118191=CYLINDRICAL_SURFACE ( 'NONE', #132126, 0.3999999999999996336 ) ;
#118224=FACE_OUTER_BOUND ( 'NONE', #48988, .T. ) ;
#118225=CARTESIAN_POINT ( 'NONE',  ( -10.50000000000000355, 10.09158320108480744, -3.600000000000000533 ) ) ;
#118229=UNCERTAINTY_MEASURE_WITH_UNIT (LENGTH_MEASURE( 1.000000000000000082E-05 ), #53637, 'distance_accuracy_value', 'NONE');
#118238=ORIENTED_EDGE ( 'NONE', *, *, #125681, .F. ) ;
#118239=ORIENTED_EDGE ( 'NONE', *, *, #180841, .F. ) ;
#118249=STYLED_ITEM ( 'NONE', ( #166222 ), #47427 ) ;
#118263=DIRECTION ( 'NONE',  ( -0.000000000000000000, -0.000000000000000000, -1.000000000000000000 ) ) ;
#118276=CARTESIAN_POINT ( 'NONE',  ( 11.84668730067608600, 12.69999999999999929, -1.400000000000001910 ) ) ;
#118279=CARTESIAN_POINT ( 'NONE',  ( -15.75000000000000000, 9.799999999999982947, 3.199999999999997957 ) ) ;
#118281=CARTESIAN_POINT ( 'NONE',  ( 10.50000000000000178, 10.19999999999998153, 3.599999999999999201 ) ) ;
#118282=CARTESIAN_POINT ( 'NONE',  ( -11.91826849282518452, 12.69999999999999929, -1.400000000000001465 ) ) ;
#118306=CARTESIAN_POINT ( 'NONE',  ( -9.193915077888615173, 15.44694766967490551, -7.646183055905130921 ) ) ;
#118342=FACE_OUTER_BOUND ( 'NONE', #100430, .T. ) ;
#118346=ORIENTED_EDGE ( 'NONE', *, *, #145457, .T. ) ;
#118348=VERTEX_POINT ( 'NONE', #108546 ) ;
#118353=CARTESIAN_POINT ( 'NONE',  ( -11.92051736251532112, 9.948197562073211486, -1.381800029228967386 ) ) ;
#118360=CARTESIAN_POINT ( 'NONE',  ( -12.04410816989902955, 7.377574010548016759, -3.959763750030863783 ) ) ;
#118382=EDGE_LOOP ( 'NONE', ( #91908, #17183, #115572, #2336, #171811, #160481, #108230, #87915 ) ) ;
#118385=CARTESIAN_POINT ( 'NONE',  ( 11.97297122925974122, 12.30125079326911575, -0.8121202983519294483 ) ) ;
#118389=( GEOMETRIC_REPRESENTATION_CONTEXT ( 3 ) GLOBAL_UNCERTAINTY_ASSIGNED_CONTEXT ( ( #60868 ) ) GLOBAL_UNIT_ASSIGNED_CONTEXT ( ( #184179, #99743, #150644 ) ) REPRESENTATION_CONTEXT ( 'NONE', 'WORKASPACE' ) );
#118424=LINE ( 'NONE', #168178, #157362 ) ;
#118425=CARTESIAN_POINT ( 'NONE',  ( -10.10575425844435138, 4.358269247758318699, 5.859476710806498900 ) ) ;
#118429=CARTESIAN_POINT ( 'NONE',  ( -11.39025776735688211, 6.535114720142842337, -3.782060309780574947 ) ) ;
#118455=COLOUR_RGB ( '', 0.08235294, 0.09019608, 0.10196078) ;
#118474=CARTESIAN_POINT ( 'NONE',  ( 9.167499922608561391, 13.31163428502020452, -9.058864735568997517 ) ) ;
#118529=CARTESIAN_POINT ( 'NONE',  ( 10.40128792240049194, 10.48955026364925835, -5.993062759042677712 ) ) ;
#118533=CARTESIAN_POINT ( 'NONE',  ( 11.88237264505823987, 13.75677038468308844, -0.9087825512663076921 ) ) ;
#118540=DIRECTION ( 'NONE',  ( 0.000000000000000000, 0.4363663406439433068, -0.8997690907966409135 ) ) ;
#118543=CIRCLE ( 'NONE', #63135, 11.09999999999999964 ) ;
#118586=CARTESIAN_POINT ( 'NONE',  ( -10.52211811376582062, 5.354010262649190111, 5.769489279399181214 ) ) ;
#118605=LINE ( 'NONE', #165162, #36175 ) ;
#118676=SURFACE_STYLE_USAGE ( .BOTH. , #52543 ) ;
#118684=CIRCLE ( 'NONE', #104732, 12.00000000000000178 ) ;
#118697=VERTEX_POINT ( 'NONE', #165762 ) ;
#118715=( NAMED_UNIT ( * ) PLANE_ANGLE_UNIT ( ) SI_UNIT ( $, .RADIAN. ) );
#118748=CARTESIAN_POINT ( 'NONE',  ( -1.878313713277967700, 15.99999999999538858, -12.68000002627077905 ) ) ;
#118750=CARTESIAN_POINT ( 'NONE',  ( -10.28816806463375144, 6.680837282875757843, -5.326249955113787848 ) ) ;
#118791=LINE ( 'NONE', #50532, #70133 ) ;
#118820=CARTESIAN_POINT ( 'NONE',  ( 11.89942855770813956, 9.799999999999998934, -0.7000000000000009548 ) ) ;
#118822=CARTESIAN_POINT ( 'NONE',  ( 11.97929049433705373, 9.719999999999998863, 0.7046979865771783036 ) ) ;
#118849=VERTEX_POINT ( 'NONE', #87700 ) ;
#118854=CARTESIAN_POINT ( 'NONE',  ( -10.65086514279933994, 4.118349190211191058, -6.883315229069521202 ) ) ;
#118865=CARTESIAN_POINT ( 'NONE',  ( -10.60630082101195804, 5.715768461961713953, -4.896526734066639186 ) ) ;
#118871=CARTESIAN_POINT ( 'NONE',  ( 11.80022143584854710, 6.865729006526965605, 1.951202288423556919 ) ) ;
#118883=CARTESIAN_POINT ( 'NONE',  ( 10.13617411650462330, 13.69189752474445321, 7.314094131634138130 ) ) ;
#118897=CARTESIAN_POINT ( 'NONE',  ( -7.090402625748199128, 15.44810097730825760, -9.636366487198095854 ) ) ;
#118919=MECHANICAL_DESIGN_GEOMETRIC_PRESENTATION_REPRESENTATION('',(#191040),#63047);
#118930=CARTESIAN_POINT ( 'NONE',  ( -9.439063867296153987, 14.51206345749796256, -7.409881739176208626 ) ) ;
#118942=CARTESIAN_POINT ( 'NONE',  ( -15.75000000000000000, 10.90000000000000036, 0.6999999999999992895 ) ) ;
#118950=CARTESIAN_POINT ( 'NONE',  ( 0.000000000000000000, 19.00000000000000000, 11.92000000000000171 ) ) ;
#118985=EDGE_CURVE ( 'NONE', #122503, #132208, #176825, .T. ) ;
#118996=CIRCLE ( 'NONE', #18578, 0.07999999999999997391 ) ;
#119011=CARTESIAN_POINT ( 'NONE',  ( 11.44779964734710909, 12.60189529870400804, 3.599999963171362616 ) ) ;
#119013=CARTESIAN_POINT ( 'NONE',  ( 11.39743721391019626, 7.463254518212971256, -3.780308495066197594 ) ) ;
#119038=VERTEX_POINT ( 'NONE', #6427 ) ;
#119064=CARTESIAN_POINT ( 'NONE',  ( 11.52469724861193612, 13.87999993351185068, 3.346365485506901827 ) ) ;
#119084=SURFACE_STYLE_USAGE ( .BOTH. , #149388 ) ;
#119089=LINE ( 'NONE', #201311, #102012 ) ;
#119106=ORIENTED_EDGE ( 'NONE', *, *, #170713, .T. ) ;
#119125=EDGE_CURVE ( 'NONE', #49028, #136644, #167697, .T. ) ;
#119142=CARTESIAN_POINT ( 'NONE',  ( -10.95308175811721085, 13.79999999999998295, 1.799999999999999600 ) ) ;
#119153=ORIENTED_EDGE ( 'NONE', *, *, #87324, .T. ) ;
#119174=ORIENTED_EDGE ( 'NONE', *, *, #179202, .T. ) ;
#119180=CARTESIAN_POINT ( 'NONE',  ( 11.92619526913700057, 11.02781666661241644, 1.328859060402684644 ) ) ;
#119185=SURFACE_SIDE_STYLE ('',( #134346 ) ) ;
#119191=( LENGTH_UNIT ( ) NAMED_UNIT ( * ) SI_UNIT ( .MILLI., .METRE. ) );
#119192=CARTESIAN_POINT ( 'NONE',  ( 11.97929049433705373, 9.719999999999998863, -0.7046979865771834106 ) ) ;
#119196=SURFACE_SIDE_STYLE ('',( #137535 ) ) ;
#119210=CARTESIAN_POINT ( 'NONE',  ( -11.94651559118242368, 11.15130655878970956, 1.135242698369626435 ) ) ;
#119212=AXIS2_PLACEMENT_3D ( 'NONE', #31730, #95678, #130365 ) ;
#119228=DIRECTION ( 'NONE',  ( 0.000000000000000000, 1.000000000000000000, 0.000000000000000000 ) ) ;
#119231=ORIENTED_EDGE ( 'NONE', *, *, #131603, .F. ) ;
#119289=CARTESIAN_POINT ( 'NONE',  ( -11.29165584589917870, 5.103824637450834700, 5.764786465619509137 ) ) ;
#119301=ORIENTED_EDGE ( 'NONE', *, *, #50025, .T. ) ;
#119318=EDGE_CURVE ( 'NONE', #121309, #67257, #136639, .T. ) ;
#119319=CARTESIAN_POINT ( 'NONE',  ( 11.89942855770814312, 9.799999999999998934, 0.6999999999999992895 ) ) ;
#119328=ORIENTED_EDGE ( 'NONE', *, *, #28655, .F. ) ;
#119340=ORIENTED_EDGE ( 'NONE', *, *, #195398, .F. ) ;
#119343=CARTESIAN_POINT ( 'NONE',  ( -10.35086068573297524, 3.817517357212610207, -6.072273895623982121 ) ) ;
#119348=CARTESIAN_POINT ( 'NONE',  ( 11.92619525870748021, 12.57377703206318920, 1.328859154005125554 ) ) ;
#119374=CARTESIAN_POINT ( 'NONE',  ( -9.048073855341844052, 15.44705409027664089, -7.818180454737184704 ) ) ;
#119406=CARTESIAN_POINT ( 'NONE',  ( 11.89197415570409611, 11.30000000000000604, 0.8055989572471813354 ) ) ;
#119408=CARTESIAN_POINT ( 'NONE',  ( -9.367496997601300279, 15.00000000000599343, -7.499999999995378808 ) ) ;
#119413=ORIENTED_EDGE ( 'NONE', *, *, #153496, .T. ) ;
#119415=AXIS2_PLACEMENT_3D ( 'NONE', #85776, #18629, #4487 ) ;
#119427=CARTESIAN_POINT ( 'NONE',  ( -10.45911201557330195, 5.175391108250987138, -5.201428006079835242 ) ) ;
#119454=CARTESIAN_POINT ( 'NONE',  ( 11.97929049433705373, 12.22000000000000064, -0.7046979865771821894 ) ) ;
#119480=SURFACE_SIDE_STYLE ('',( #170288 ) ) ;
#119494=TOROIDAL_SURFACE ( 'NONE', #91784, 11.92000000000000171, 0.08000000000000000167 ) ;
#119520=AXIS2_PLACEMENT_3D ( 'NONE', #201714, #37101, #20829 ) ;
#119540=CARTESIAN_POINT ( 'NONE',  ( 9.634427881463707877, 13.63015724552533037, -8.222364378050974310 ) ) ;
#119546=ORIENTED_EDGE ( 'NONE', *, *, #195328, .T. ) ;
#119556=CARTESIAN_POINT ( 'NONE',  ( 11.94105721237522921, 13.52740784401788687, -1.187919463087249605 ) ) ;
#119560=VECTOR ( 'NONE', #45880, 1000.000000000000000 ) ;
#119568=CARTESIAN_POINT ( 'NONE',  ( -10.44369633504468631, 5.112959841837462882, -5.232137017608344820 ) ) ;
#119573=CARTESIAN_POINT ( 'NONE',  ( 8.220249535482631487, 15.16568599130686223, -8.682936656944493237 ) ) ;
#119599=CARTESIAN_POINT ( 'NONE',  ( 9.955160869828317161, 11.52437543985780266, -6.705892285181387358 ) ) ;
#119609=DIRECTION ( 'NONE',  ( 0.000000000000000000, 0.000000000000000000, 1.000000000000000000 ) ) ;
#119670=CARTESIAN_POINT ( 'NONE',  ( 0.000000000000000000, 13.79999999999998295, 0.000000000000000000 ) ) ;
#119683=( BOUNDED_SURFACE ( )  B_SPLINE_SURFACE ( 3, 2, ( 
 ( #75672, #156937, #124509 ),
 ( #176376, #158007, #59414 ),
 ( #73529, #42128, #27982 ),
 ( #91945, #177437, #139631 ),
 ( #44249, #111434, #207786 ),
 ( #107167, #205654, #29054 ) ),
 .UNSPECIFIED., .F., .F., .T. ) 
 B_SPLINE_SURFACE_WITH_KNOTS ( ( 4, 2, 4 ),
 ( 3, 3 ),
 ( 0.000000000000000000, 0.0003766405729503173702, 0.0007532811459006347405 ),
 ( 0.000000000000000000, 1.000000000000000000 ),
 .UNSPECIFIED. ) 
 GEOMETRIC_REPRESENTATION_ITEM ( )  RATIONAL_B_SPLINE_SURFACE ( (
 ( 1.000000000000000000, 0.7071067811865551223, 1.000000000000000000),
 ( 1.000000000000000000, 0.7211294902955875941, 1.000000000000000000),
 ( 1.000000000000000000, 0.7311181975227702967, 1.000000000000000000),
 ( 1.000000000000000000, 0.7429553055063979894, 1.000000000000000000),
 ( 1.000000000000000000, 0.7451698531056455410, 1.000000000000000000),
 ( 1.000000000000000000, 0.7452309222762957264, 1.000000000000000000) ) ) 
 REPRESENTATION_ITEM ( '' )  SURFACE ( )  );
#119712=CARTESIAN_POINT ( 'NONE',  ( -11.98811477081661536, 9.050839079014156852, 0.6170501206370091474 ) ) ;
#119793=STYLED_ITEM ( 'NONE', ( #180337 ), #15900 ) ;
#119821=CARTESIAN_POINT ( 'NONE',  ( 0.7124089920921192753, 16.00000000000000711, -12.66466791154696914 ) ) ;
#119823=CARTESIAN_POINT ( 'NONE',  ( -10.45911201557330195, 5.175391108250987138, -5.201428006079835242 ) ) ;
#119830=AXIS2_PLACEMENT_3D ( 'NONE', #158585, #43791, #90387 ) ;
#119831=CARTESIAN_POINT ( 'NONE',  ( -1.416786528094066577, 7.999640415717689912, -11.00953083556809453 ) ) ;
#119835=ORIENTED_EDGE ( 'NONE', *, *, #205156, .T. ) ;
#119844=CARTESIAN_POINT ( 'NONE',  ( -9.569358774149646862, 4.446947634372958369, 7.167287524840457280 ) ) ;
#119856=SURFACE_SIDE_STYLE ('',( #65673 ) ) ;
#119858=DIRECTION ( 'NONE',  ( -0.9632918427306595976, 0.000000000000000000, -0.2684563758389253985 ) ) ;
#119864=FILL_AREA_STYLE_COLOUR ( '', #115447 ) ;
#119902=CARTESIAN_POINT ( 'NONE',  ( -11.78331023100045627, 12.29999999999998295, 1.799999999999999600 ) ) ;
#119931=CARTESIAN_POINT ( 'NONE',  ( -9.510997388311002609, 3.006837337344905325, -6.782141846552069531 ) ) ;
#119948=CARTESIAN_POINT ( 'NONE',  ( 11.75312296564416847, 6.986206119746739773, -2.433357306325415692 ) ) ;
#119957=ORIENTED_EDGE ( 'NONE', *, *, #201940, .F. ) ;
#119960=CARTESIAN_POINT ( 'NONE',  ( 8.486526397101934904, 12.59978548610894578, -8.445610199728610823 ) ) ;
#119969=CARTESIAN_POINT ( 'NONE',  ( -9.333041836230016486, 15.44694763438214125, 7.472413793098208856 ) ) ;
#119972=CARTESIAN_POINT ( 'NONE',  ( -1.797499070710327107, 15.51994604999343608, -11.89808504883940543 ) ) ;
#119979=CARTESIAN_POINT ( 'NONE',  ( -9.367496997601300279, 15.00000000000599165, 7.679999999987998649 ) ) ;
#119981=AXIS2_PLACEMENT_3D ( 'NONE', #68187, #136433, #117032 ) ;
#119987=LINE ( 'NONE', #19197, #87450 ) ;
#120003=FILL_AREA_STYLE ('',( #69019 ) ) ;
#120015=CARTESIAN_POINT ( 'NONE',  ( 11.88237951145550220, 13.75680652621284317, -0.9087114598430711121 ) ) ;
#120019=CARTESIAN_POINT ( 'NONE',  ( -10.43233925736708301, 5.066585305077033752, -5.254699789447807134 ) ) ;
#120020=AXIS2_PLACEMENT_3D ( 'NONE', #105818, #204306, #73255 ) ;
#120030=AXIS2_PLACEMENT_3D ( 'NONE', #171988, #3047, #136295 ) ;
#120034=CARTESIAN_POINT ( 'NONE',  ( -11.86145016429273191, 19.00000000000000000, 1.179999999999997051 ) ) ;
#120036=DIRECTION ( 'NONE',  ( 0.7806247498251047690, 0.000000000000000000, 0.6249999999683939489 ) ) ;
#120046=DIRECTION ( 'NONE',  ( 0.000000000000000000, 0.000000000000000000, -1.000000000000000000 ) ) ;
#120084=UNCERTAINTY_MEASURE_WITH_UNIT (LENGTH_MEASURE( 1.000000000000000082E-05 ), #114427, 'distance_accuracy_value', 'NONE');
#120085=DIRECTION ( 'NONE',  ( -0.000000000000000000, -1.000000000000000000, -0.000000000000000000 ) ) ;
#120088=CARTESIAN_POINT ( 'NONE',  ( 11.52901446936747298, 12.30574472532411434, 3.330874149801136053 ) ) ;
#120090=LINE ( 'NONE', #152514, #46054 ) ;
#120109=VERTEX_POINT ( 'NONE', #199028 ) ;
#120115=DIRECTION ( 'NONE',  ( 1.000000000000000000, 0.000000000000000000, -0.000000000000000000 ) ) ;
#120123=DIRECTION ( 'NONE',  ( 0.000000000000000000, 0.000000000000000000, -1.000000000000000000 ) ) ;
#120175=AXIS2_PLACEMENT_3D ( 'NONE', #140455, #89179, #57729 ) ;
#120187=STYLED_ITEM ( 'NONE', ( #22522 ), #149381 ) ;
#120218=FACE_OUTER_BOUND ( 'NONE', #110126, .T. ) ;
#120220=EDGE_LOOP ( 'NONE', ( #35959, #208431, #206197, #158473 ) ) ;
#120224=CARTESIAN_POINT ( 'NONE',  ( -10.43230948805442893, 5.066484524551064794, 5.254757398418679060 ) ) ;
#120256=EDGE_LOOP ( 'NONE', ( #43442, #160994, #148447, #10789 ) ) ;
#120263=SURFACE_STYLE_USAGE ( .BOTH. , #139664 ) ;
#120283=EDGE_CURVE ( 'NONE', #102449, #112981, #205879, .T. ) ;
#120289=ADVANCED_FACE ( 'NONE', ( #137285 ), #106571, .T. ) ;
#120319=LINE ( 'NONE', #151693, #7507 ) ;
#120320=DIRECTION ( 'NONE',  ( -0.000000000000000000, -1.000000000000000000, -0.000000000000000000 ) ) ;
#120328=ORIENTED_EDGE ( 'NONE', *, *, #70447, .F. ) ;
#120358=DIRECTION ( 'NONE',  ( 0.000000000000000000, 0.000000000000000000, 1.000000000000000000 ) ) ;
#120361=( LENGTH_UNIT ( ) NAMED_UNIT ( * ) SI_UNIT ( .MILLI., .METRE. ) );
#120370=CARTESIAN_POINT ( 'NONE',  ( -9.956232484441596142, 5.504245459870187318, 6.026037945409589369 ) ) ;
#120371=ORIENTED_EDGE ( 'NONE', *, *, #83347, .F. ) ;
#120374=CARTESIAN_POINT ( 'NONE',  ( -1.349890321011207206, 8.200329036966270024, 10.79298809153610961 ) ) ;
#120383=ORIENTED_EDGE ( 'NONE', *, *, #89670, .F. ) ;
#120399=CARTESIAN_POINT ( 'NONE',  ( -3.594090741707730796, 15.51961551409570994, 11.45768715124896708 ) ) ;
#120407=EDGE_CURVE ( 'NONE', #108500, #79124, #36251, .T. ) ;
#120419=VERTEX_POINT ( 'NONE', #210789 ) ;
#120428=CARTESIAN_POINT ( 'NONE',  ( -11.87828357749937069, 12.29689747259577892, -1.708055325888869325 ) ) ;
#120436=TOROIDAL_SURFACE ( 'NONE', #165347, -0.1799999999926198968, 0.5000000000000013323 ) ;
#120456=LINE ( 'NONE', #88963, #33670 ) ;
#120465=DIRECTION ( 'NONE',  ( 0.000000000000000000, -1.000000000000000000, 0.000000000000000000 ) ) ;
#120472=CYLINDRICAL_SURFACE ( 'NONE', #79440, 11.09999999999999964 ) ;
#120489=DIRECTION ( 'NONE',  ( -0.000000000000000000, 0.000000000000000000, -1.000000000000000000 ) ) ;
#120497=EDGE_CURVE ( 'NONE', #116248, #49891, #118424, .T. ) ;
#120510=CARTESIAN_POINT ( 'NONE',  ( -10.97400665845581536, 4.893988168282350948, 4.351071648605314479 ) ) ;
#120520=CARTESIAN_POINT ( 'NONE',  ( 9.780965096007749437, 12.99495041104594861, 8.039825270927440926 ) ) ;
#120529=CARTESIAN_POINT ( 'NONE',  ( -10.51582573219070227, 13.61290858478269605, 3.554376768052134317 ) ) ;
#120558=EDGE_LOOP ( 'NONE', ( #199507, #86649, #37881, #185894 ) ) ;
#120568=ORIENTED_EDGE ( 'NONE', *, *, #112880, .F. ) ;
#120570=EDGE_CURVE ( 'NONE', #143955, #50054, #25895, .T. ) ;
#120580=DIRECTION ( 'NONE',  ( -0.000000000000000000, -1.000000000000000000, -0.000000000000000000 ) ) ;
#120606=CIRCLE ( 'NONE', #165505, 12.00000000000000178 ) ;
#120624=CARTESIAN_POINT ( 'NONE',  ( 9.664668247050562044, 13.51658191024029243, -8.185676666504042132 ) ) ;
#120630=EDGE_LOOP ( 'NONE', ( #54048, #68869, #197933, #110784 ) ) ;
#120672=CARTESIAN_POINT ( 'NONE',  ( 8.665088397661675046, 14.86833811616255119, 8.238078554563339040 ) ) ;
#120677=PRESENTATION_STYLE_ASSIGNMENT (( #202884 ) ) ;
#120681=EDGE_CURVE ( 'NONE', #59570, #193391, #47797, .T. ) ;
#120792=CARTESIAN_POINT ( 'NONE',  ( -12.00000747045989691, 9.073125656298698161, 0.3084868119113360896 ) ) ;
#120795=EDGE_CURVE ( 'NONE', #33851, #99973, #153653, .T. ) ;
#120837=ORIENTED_EDGE ( 'NONE', *, *, #128643, .F. ) ;
#120846=VECTOR ( 'NONE', #77482, 1000.000000000000000 ) ;
#120854=FILL_AREA_STYLE ('',( #5922 ) ) ;
#120879=UNCERTAINTY_MEASURE_WITH_UNIT (LENGTH_MEASURE( 1.000000000000000082E-05 ), #10082, 'distance_accuracy_value', 'NONE');
#120906=CARTESIAN_POINT ( 'NONE',  ( -10.57232049882948388, 5.599334429189661400, -4.968988939937085014 ) ) ;
#120924=CARTESIAN_POINT ( 'NONE',  ( -11.07790593930098311, 9.799999999999998934, -0.7000000000000009548 ) ) ;
#120939=B_SPLINE_CURVE_WITH_KNOTS ( 'NONE', 3,
 ( #163784, #15363, #81456, #42846, #92662, #10303 ),
 .UNSPECIFIED., .F., .F.,
 ( 4, 2, 4 ),
 ( 0.000000000000000000, 0.0003157158648874029564, 0.0006314317297748059127 ),
 .UNSPECIFIED. ) ;
#120944=AXIS2_PLACEMENT_3D ( 'NONE', #203147, #55852, #74247 ) ;
#120949=DIRECTION ( 'NONE',  ( 0.000000000000000000, 1.000000000000000000, 0.000000000000000000 ) ) ;
#120967=ADVANCED_FACE ( 'NONE', ( #53355 ), #90145, .F. ) ;
#120980=ORIENTED_EDGE ( 'NONE', *, *, #71437, .T. ) ;
#120987=DIRECTION ( 'NONE',  ( 0.8594003466332824637, -0.03762549425793430824, 0.5099170191202098135 ) ) ;
#121019=CARTESIAN_POINT ( 'NONE',  ( -10.68988767858338917, 3.994679225574373493, -4.900161361628223133 ) ) ;
#121030=CARTESIAN_POINT ( 'NONE',  ( -10.44369227015510404, 5.112964020592957404, 5.232143560358708534 ) ) ;
#121036=CARTESIAN_POINT ( 'NONE',  ( 11.84619309640116747, 6.793804897517921049, 1.976512447145533091 ) ) ;
#121060=EDGE_CURVE ( 'NONE', #201490, #64100, #171405, .T. ) ;
#121070=PLANE ( 'NONE',  #201672 ) ;
#121098=TOROIDAL_SURFACE ( 'NONE', #69029, -0.1799999999926198968, 0.5000000000000013323 ) ;
#121100=CYLINDRICAL_SURFACE ( 'NONE', #89308, 0.3999999999999996336 ) ;
#121104=CARTESIAN_POINT ( 'NONE',  ( -10.37923916842784422, 4.890109552615133026, -5.358306740738790097 ) ) ;
#121110=CARTESIAN_POINT ( 'NONE',  ( 11.78331023100045627, 11.37999999999999901, -1.800000000000001155 ) ) ;
#121119=VECTOR ( 'NONE', #38882, 1000.000000000000000 ) ;
#121123=VERTEX_POINT ( 'NONE', #57633 ) ;
#121129=EDGE_CURVE ( 'NONE', #77503, #146971, #195085, .T. ) ;
#121171=COLOUR_RGB ( '', 0.66274510, 0.83137255, 0.94901961) ;
#121185=CARTESIAN_POINT ( 'NONE',  ( -11.88235317400313917, 13.75664239773029784, -0.9089793033029951452 ) ) ;
#121190=ORIENTED_EDGE ( 'NONE', *, *, #150613, .F. ) ;
#121193=CYLINDRICAL_SURFACE ( 'NONE', #21198, 0.3999999999999997446 ) ;
#121197=CARTESIAN_POINT ( 'NONE',  ( 11.97181073603049484, 13.88000000000000256, 0.8318477717169565633 ) ) ;
#121220=PRESENTATION_STYLE_ASSIGNMENT (( #169870 ) ) ;
#121224=CARTESIAN_POINT ( 'NONE',  ( 11.55950211276791251, 13.79999999999998472, 3.221476510067111665 ) ) ;
#121239=CARTESIAN_POINT ( 'NONE',  ( 9.681502816803464029, 4.134754161804807815, -7.090028435276412466 ) ) ;
#121242=DIRECTION ( 'NONE',  ( 0.8164965809277274778, -1.132850316508781087E-13, -0.5773502691896237327 ) ) ;
#121281=CARTESIAN_POINT ( 'NONE',  ( -11.84668729410370602, 10.09379487675469633, 1.399999999999998357 ) ) ;
#121298=CARTESIAN_POINT ( 'NONE',  ( -11.94105721237523277, 13.40000000000000036, 1.187919463087245386 ) ) ;
#121299=CARTESIAN_POINT ( 'NONE',  ( -10.81012925547440773, 5.523932969818027949, 6.547168141744070802 ) ) ;
#121307=EDGE_CURVE ( 'NONE', #200740, #37563, #105732, .T. ) ;
#121309=VERTEX_POINT ( 'NONE', #169537 ) ;
#121310=AXIS2_PLACEMENT_3D ( 'NONE', #4784, #73012, #8013 ) ;
#121328=CARTESIAN_POINT ( 'NONE',  ( -4.379728251965876673, 15.51893462891072595, -11.18122699412752397 ) ) ;
#121337=( NAMED_UNIT ( * ) PLANE_ANGLE_UNIT ( ) SI_UNIT ( $, .RADIAN. ) );
#121375=ADVANCED_FACE ( 'NONE', ( #153287 ), #599, .F. ) ;
#121376=CARTESIAN_POINT ( 'NONE',  ( 0.000000000000000000, 8.500000000000000000, 0.000000000000000000 ) ) ;
#121397=CARTESIAN_POINT ( 'NONE',  ( -1.748073236337231107, 15.51991758800158117, 11.90628676210878822 ) ) ;
#121410=CARTESIAN_POINT ( 'NONE',  ( 0.000000000000000000, 7.000000000000000000, 0.000000000000000000 ) ) ;
#121416=CARTESIAN_POINT ( 'NONE',  ( 11.86239285000045740, 12.21999999999998288, 1.812080536912751061 ) ) ;
#121431=B_SPLINE_CURVE_WITH_KNOTS ( 'NONE', 3,
 ( #7581, #109444, #175451, #27035, #76857, #72588 ),
 .UNSPECIFIED., .F., .F.,
 ( 4, 2, 4 ),
 ( 0.000000000000000000, 0.0003844267940947831432, 0.0007688535881895662864 ),
 .UNSPECIFIED. ) ;
#121447=CARTESIAN_POINT ( 'NONE',  ( -10.32184838934336213, 3.007359993651753438, 7.367400555339857604 ) ) ;
#121462=DIRECTION ( 'NONE',  ( 1.000000000000000000, -0.000000000000000000, -0.000000000000000000 ) ) ;
#121484=ORIENTED_EDGE ( 'NONE', *, *, #68124, .F. ) ;
#121488=CARTESIAN_POINT ( 'NONE',  ( 11.94980361058169116, 13.39999999999999858, 1.099999999999994982 ) ) ;
#121497=CARTESIAN_POINT ( 'NONE',  ( -9.604686356149274573, 3.530925729795075796, -7.193747284969078670 ) ) ;
#121502=CARTESIAN_POINT ( 'NONE',  ( 11.88172094500853859, 12.22000005601592321, 1.685553348215818925 ) ) ;
#121519=EDGE_CURVE ( 'NONE', #130695, #95488, #40106, .T. ) ;
#121529=ADVANCED_FACE ( 'NONE', ( #154361 ), #156104, .F. ) ;
#121531=CARTESIAN_POINT ( 'NONE',  ( -15.75000000000000000, 12.29999999999998295, 1.799999999999999600 ) ) ;
#121570=VERTEX_POINT ( 'NONE', #8807 ) ;
#121580=FILL_AREA_STYLE ('',( #8803 ) ) ;
#121581=CARTESIAN_POINT ( 'NONE',  ( -11.82816107619417778, 7.167718870070345361, 1.885585305228718589 ) ) ;
#121582=TOROIDAL_SURFACE ( 'NONE', #97386, 11.92000000000000171, 0.08000000000000000167 ) ;
#121607=CIRCLE ( 'NONE', #149185, 0.07999999999999998779 ) ;
#121609=CARTESIAN_POINT ( 'NONE',  ( 11.86145016429273191, 12.69999999999999929, -1.100000000000000533 ) ) ;
#121612=ADVANCED_FACE ( 'NONE', ( #209120 ), #83959, .T. ) ;
#121644=ORIENTED_EDGE ( 'NONE', *, *, #105829, .T. ) ;
#121648=DIRECTION ( 'NONE',  ( -0.000000000000000000, -1.000000000000000000, -0.000000000000000000 ) ) ;
#121705=ADVANCED_FACE ( 'NONE', ( #66051 ), #145256, .T. ) ;
#121746=CARTESIAN_POINT ( 'NONE',  ( 9.100815109899395239, 14.29680943629558776, 7.752531514792824652 ) ) ;
#121752=CARTESIAN_POINT ( 'NONE',  ( -11.52114515671133610, 8.081606464056415362, 2.192706985476595261 ) ) ;
#121757=CARTESIAN_POINT ( 'NONE',  ( -3.543593105830169065, 14.52998843158304254, -11.47354445632842257 ) ) ;
#121811=CARTESIAN_POINT ( 'NONE',  ( -9.333041836230696831, 14.55305236563169302, -7.472413793098840351 ) ) ;
#121815=STYLED_ITEM ( 'NONE', ( #34728 ), #61220 ) ;
#121817=VERTEX_POINT ( 'NONE', #63957 ) ;
#121841=CARTESIAN_POINT ( 'NONE',  ( -11.52901446936791352, 9.805744725324480271, -3.330874149801263506 ) ) ;
#121852=COLOUR_RGB ( '', 0.31764706, 0.68627451, 0.89019608) ;
#121853=CARTESIAN_POINT ( 'NONE',  ( 9.445304453185899618, 4.469082159062008230, -7.402818517570769252 ) ) ;
#121856=CYLINDRICAL_SURFACE ( 'NONE', #194242, 0.07999999999999998779 ) ;
#121863=CARTESIAN_POINT ( 'NONE',  ( -11.32514615057358043, 7.707209080198650142, -3.974810102870973694 ) ) ;
#121870=AXIS2_PLACEMENT_3D ( 'NONE', #97966, #180265, #15599 ) ;
#121896=MECHANICAL_DESIGN_GEOMETRIC_PRESENTATION_REPRESENTATION('',(#25028),#111526);
#121920=EDGE_CURVE ( 'NONE', #169596, #124, #16659, .T. ) ;
#121936=CARTESIAN_POINT ( 'NONE',  ( 10.20550892794189579, 9.995811918519301287, 6.492953855302722843 ) ) ;
#121943=CARTESIAN_POINT ( 'NONE',  ( 8.057215556046470439, 15.94308538975788281, 9.795211633567449283 ) ) ;
#121965=AXIS2_PLACEMENT_3D ( 'NONE', #137633, #152797, #85659 ) ;
#121978=CARTESIAN_POINT ( 'NONE',  ( -11.30309668167796922, 5.150585336095397260, -5.742054036728555744 ) ) ;
#122007=ORIENTED_EDGE ( 'NONE', *, *, #131977, .F. ) ;
#122019=( NAMED_UNIT ( * ) PLANE_ANGLE_UNIT ( ) SI_UNIT ( $, .RADIAN. ) );
#122038=DIRECTION ( 'NONE',  ( 0.9982742078614211811, 0.000000000000000000, 0.05872483221476467591 ) ) ;
#122043=DIRECTION ( 'NONE',  ( 1.000000000000000000, -0.000000000000000000, -0.000000000000000000 ) ) ;
#122049=EDGE_LOOP ( 'NONE', ( #22885, #102693, #51599, #174725 ) ) ;
#122088=CARTESIAN_POINT ( 'NONE',  ( -11.69084473744764097, 4.401359152538248054, -5.144113628910231384 ) ) ;
#122097=CARTESIAN_POINT ( 'NONE',  ( -10.05286969158539812, 5.876479340494690895, 5.831501649199077875 ) ) ;
#122101=ORIENTED_EDGE ( 'NONE', *, *, #66969, .T. ) ;
#122103=CARTESIAN_POINT ( 'NONE',  ( 8.880228351732188941, 12.81718488518845156, 8.003373899717370676 ) ) ;
#122113=EDGE_LOOP ( 'NONE', ( #109921, #190876, #68911, #81309 ) ) ;
#122132=CARTESIAN_POINT ( 'NONE',  ( -11.94105721237523099, 13.40000000000000036, -1.187919463087249827 ) ) ;
#122169=FILL_AREA_STYLE_COLOUR ( '', #179436 ) ;
#122174=CARTESIAN_POINT ( 'NONE',  ( -10.14891672641957499, 5.000029895416906456, -7.601366607803407227 ) ) ;
#122184=DIRECTION ( 'NONE',  ( 0.05872483221476459958, 0.000000000000000000, 0.9982742078614211811 ) ) ;
#122191=( GEOMETRIC_REPRESENTATION_CONTEXT ( 3 ) GLOBAL_UNCERTAINTY_ASSIGNED_CONTEXT ( ( #148541 ) ) GLOBAL_UNIT_ASSIGNED_CONTEXT ( ( #53701, #152271, #7053 ) ) REPRESENTATION_CONTEXT ( 'NONE', 'WORKASPACE' ) );
#122245=CARTESIAN_POINT ( 'NONE',  ( 11.80247861663003484, 13.79999999999999716, -1.695431928471867966 ) ) ;
#122257=B_SPLINE_CURVE_WITH_KNOTS ( 'NONE', 3,
 ( #53244, #118306, #119374, #34842, #185361, #54315, #103066, #169122, #170182, #86810, #152876, #116172, #84675, #4454, #70524, #33788, #1265, #136641, #67324, #133468, #199471, #51113 ),
 .UNSPECIFIED., .F., .F.,
 ( 4, 2, 2, 2, 2, 2, 2, 2, 2, 2, 4 ),
 ( -5.999999999670954957E-08, 0.0006677484337924339576, 0.001335556867584864740, 0.002671173735169722618, 0.004006790602754580280, 0.005342407470339437942, 0.006678024337924295603, 0.008013641205509153265, 0.009349258073094010926, 0.01001706650688643715, 0.01068487494067886685 ),
 .UNSPECIFIED. ) ;
#122278=SURFACE_SIDE_STYLE ('',( #136313 ) ) ;
#122286=TOROIDAL_SURFACE ( 'NONE', #11474, 11.92000000000000171, 0.08000000000000000167 ) ;
#122296=CARTESIAN_POINT ( 'NONE',  ( 0.000000000000000000, 11.37999999999998302, 0.000000000000000000 ) ) ;
#122301=CARTESIAN_POINT ( 'NONE',  ( 11.33772467203841572, 13.50732847981847939, 3.599999999999999201 ) ) ;
#122307=SURFACE_SIDE_STYLE ('',( #123375 ) ) ;
#122361=CARTESIAN_POINT ( 'NONE',  ( 11.55950211276791251, 13.88000000000000078, -3.221476510067114329 ) ) ;
#122377=ORIENTED_EDGE ( 'NONE', *, *, #197814, .F. ) ;
#122381=CARTESIAN_POINT ( 'NONE',  ( -9.811677024507259759, 4.107325997343203028, 6.339424533126782002 ) ) ;
#122400=CARTESIAN_POINT ( 'NONE',  ( 1.469576158976824144E-15, 18.91999999999999815, 12.00000000000000178 ) ) ;
#122407=DIRECTION ( 'NONE',  ( 0.000000000000000000, -1.000000000000000000, 0.000000000000000000 ) ) ;
#122415=CARTESIAN_POINT ( 'NONE',  ( 10.62873463776380056, 9.799999999999998934, -3.200000000000001510 ) ) ;
#122419=CARTESIAN_POINT ( 'NONE',  ( 0.000000000000000000, 9.799999999999982947, 0.000000000000000000 ) ) ;
#122420=CARTESIAN_POINT ( 'NONE',  ( -11.84668730067608600, 10.89999999999998259, 1.399999999999998579 ) ) ;
#122426=ORIENTED_EDGE ( 'NONE', *, *, #102711, .F. ) ;
#122427=PLANE ( 'NONE',  #15410 ) ;
#122428=DIRECTION ( 'NONE',  ( 0.000000000000000000, 0.000000000000000000, -1.000000000000000000 ) ) ;
#122431=MECHANICAL_DESIGN_GEOMETRIC_PRESENTATION_REPRESENTATION('',(#94684),#28961);
#122445=AXIS2_PLACEMENT_3D ( 'NONE', #163206, #180509, #32129 ) ;
#122460=ADVANCED_FACE ( 'NONE', ( #140301 ), #2343, .T. ) ;
#122476=CARTESIAN_POINT ( 'NONE',  ( -5.973748133451506348, 15.46936577441865168, 10.41719235512011998 ) ) ;
#122486=CARTESIAN_POINT ( 'NONE',  ( -10.95308175811721085, 11.29999999999998117, 1.799999999999999600 ) ) ;
#122491=CARTESIAN_POINT ( 'NONE',  ( 11.46886997981669509, 8.378336224489386197, 3.378633107758532095 ) ) ;
#122495=EDGE_CURVE ( 'NONE', #20303, #50054, #147298, .T. ) ;
#122503=VERTEX_POINT ( 'NONE', #106751 ) ;
#122514=PLANE ( 'NONE',  #161246 ) ;
#122524=CARTESIAN_POINT ( 'NONE',  ( -11.73082749631449140, 4.534045925630191931, 5.066687987500840151 ) ) ;
#122528=UNCERTAINTY_MEASURE_WITH_UNIT (LENGTH_MEASURE( 1.000000000000000082E-05 ), #55190, 'distance_accuracy_value', 'NONE');
#122534=VERTEX_POINT ( 'NONE', #10254 ) ;
#122539=ORIENTED_EDGE ( 'NONE', *, *, #49979, .F. ) ;
#122575=CARTESIAN_POINT ( 'NONE',  ( -11.04536101718726293, 12.59409062111168609, -1.100000000000000311 ) ) ;
#122588=CARTESIAN_POINT ( 'NONE',  ( 11.86145016429273191, 13.40000000000000036, 1.099999999999996758 ) ) ;
#122608=MECHANICAL_DESIGN_GEOMETRIC_PRESENTATION_REPRESENTATION('',(#67119),#23408);
#122610=EDGE_LOOP ( 'NONE', ( #32374, #49383, #200713, #72257 ) ) ;
#122646=ORIENTED_EDGE ( 'NONE', *, *, #192009, .T. ) ;
#122660=DIRECTION ( 'NONE',  ( 1.000000000000000000, -0.000000000000000000, -0.000000000000000000 ) ) ;
#122661=CARTESIAN_POINT ( 'NONE',  ( -11.19364298753552411, 5.612864353363596237, -3.868560769348357464 ) ) ;
#122663=CARTESIAN_POINT ( 'NONE',  ( -11.44779965693287416, 10.10313923201287700, 3.599999932275866676 ) ) ;
#122666=AXIS2_PLACEMENT_3D ( 'NONE', #92230, #75947, #155070 ) ;
#122669=CARTESIAN_POINT ( 'NONE',  ( 11.86145016429273369, 12.59412591486744759, -1.100000000000002087 ) ) ;
#122675=CARTESIAN_POINT ( 'NONE',  ( 11.96212011828584387, 12.27187554950052295, 0.9569185076417748848 ) ) ;
#122689=ORIENTED_EDGE ( 'NONE', *, *, #71412, .F. ) ;
#122691=FACE_OUTER_BOUND ( 'NONE', #21253, .T. ) ;
#122694=CARTESIAN_POINT ( 'NONE',  ( 0.000000000000000000, 12.21999999999998288, 0.000000000000000000 ) ) ;
#122728=( NAMED_UNIT ( * ) SI_UNIT ( $, .STERADIAN. ) SOLID_ANGLE_UNIT ( ) );
#122733=( NAMED_UNIT ( * ) SI_UNIT ( $, .STERADIAN. ) SOLID_ANGLE_UNIT ( ) );
#122779=CARTESIAN_POINT ( 'NONE',  ( -11.89197369110780045, 12.30000000000000604, -0.8056055387119882560 ) ) ;
#122782=LINE ( 'NONE', #155189, #94482 ) ;
#122784=ORIENTED_EDGE ( 'NONE', *, *, #64259, .F. ) ;
#122832=ORIENTED_EDGE ( 'NONE', *, *, #142608, .F. ) ;
#122836=LINE ( 'NONE', #23071, #21096 ) ;
#122841=CARTESIAN_POINT ( 'NONE',  ( -5.601541066505636657, 14.53093293999984681, -10.62175398270116489 ) ) ;
#122880=PLANE ( 'NONE',  #55929 ) ;
#122914=DIRECTION ( 'NONE',  ( 0.000000000000000000, 1.000000000000000000, 0.000000000000000000 ) ) ;
#122926=CARTESIAN_POINT ( 'NONE',  ( -11.55950211276791251, 9.719999999999998863, -3.221476510067115662 ) ) ;
#122928=EDGE_CURVE ( 'NONE', #30243, #64100, #65357, .T. ) ;
#122941=FACE_OUTER_BOUND ( 'NONE', #93460, .T. ) ;
#122948=CARTESIAN_POINT ( 'NONE',  ( -11.40750169882514520, 7.888053100162446540, 3.733381924586108624 ) ) ;
#122950=DIRECTION ( 'NONE',  ( -0.000000000000000000, 1.000000000000000000, -0.000000000000000000 ) ) ;
#122960=AXIS2_PLACEMENT_3D ( 'NONE', #56031, #122184, #141590 ) ;
#123004=PRESENTATION_STYLE_ASSIGNMENT (( #104528 ) ) ;
#123014=CARTESIAN_POINT ( 'NONE',  ( -11.48243876534946217, 11.29999999999998117, 3.199999999999997957 ) ) ;
#123017=( LENGTH_UNIT ( ) NAMED_UNIT ( * ) SI_UNIT ( .MILLI., .METRE. ) );
#123026=CARTESIAN_POINT ( 'NONE',  ( 0.000000000000000000, 15.00000000000000000, 0.000000000000000000 ) ) ;
#123033=CARTESIAN_POINT ( 'NONE',  ( 7.947120472790364154, 14.95225098152464582, 9.881210053433072460 ) ) ;
#123041=UNCERTAINTY_MEASURE_WITH_UNIT (LENGTH_MEASURE( 1.000000000000000082E-05 ), #21195, 'distance_accuracy_value', 'NONE');
#123067=CARTESIAN_POINT ( 'NONE',  ( -11.77618483200234500, 4.711409542047888976, 4.977076041189349098 ) ) ;
#123069=MECHANICAL_DESIGN_GEOMETRIC_PRESENTATION_REPRESENTATION('',(#1856),#209365);
#123090=LINE ( 'NONE', #170661, #211493 ) ;
#123131=FILL_AREA_STYLE ('',( #210391 ) ) ;
#123133=ADVANCED_FACE ( 'NONE', ( #51299 ), #207566, .T. ) ;
#123146=DIRECTION ( 'NONE',  ( -1.000000000000000000, -8.267061968666011278E-31, 1.224646799147343593E-16 ) ) ;
#123149=CARTESIAN_POINT ( 'NONE',  ( -10.99777869561574661, 5.379318780083400142, 4.807744692366845207 ) ) ;
#123168=EDGE_CURVE ( 'NONE', #177320, #156205, #202316, .T. ) ;
#123175=STYLED_ITEM ( 'NONE', ( #191132 ), #140161 ) ;
#123181=CARTESIAN_POINT ( 'NONE',  ( -10.50659947519749693, 5.359800460605414152, -5.105385958519358169 ) ) ;
#123196=VERTEX_POINT ( 'NONE', #82721 ) ;
#123209=CARTESIAN_POINT ( 'NONE',  ( -11.84668730067608600, 13.39999999999998259, 1.399999999999998579 ) ) ;
#123251=CARTESIAN_POINT ( 'NONE',  ( -9.645406396194509568, 4.042443384815813445, -6.587269312116742270 ) ) ;
#123262=EDGE_CURVE ( 'NONE', #140594, #114917, #109597, .T. ) ;
#123279=( NAMED_UNIT ( * ) PLANE_ANGLE_UNIT ( ) SI_UNIT ( $, .RADIAN. ) );
#123315=CARTESIAN_POINT ( 'NONE',  ( 11.53271246284126406, 7.258204413557574064, -3.348426109308498155 ) ) ;
#123335=VERTEX_POINT ( 'NONE', #187681 ) ;
#123341=DIRECTION ( 'NONE',  ( 0.9982742078614211811, 0.000000000000000000, -0.05872483221476467591 ) ) ;
#123342=CARTESIAN_POINT ( 'NONE',  ( 11.94654170777226376, 13.65174326158935791, 1.134972293687618539 ) ) ;
#123363=CARTESIAN_POINT ( 'NONE',  ( 9.398334472548928176, 13.71816428308574842, -7.461477588779884762 ) ) ;
#123364=DIRECTION ( 'NONE',  ( 0.000000000000000000, 1.000000000000000000, 0.000000000000000000 ) ) ;
#123375=SURFACE_STYLE_FILL_AREA ( #204496 ) ;
#123377=EDGE_CURVE ( 'NONE', #157191, #33058, #108644, .T. ) ;
#123419=SURFACE_STYLE_FILL_AREA ( #57258 ) ;
#123420=AXIS2_PLACEMENT_3D ( 'NONE', #62154, #113101, #30729 ) ;
#123444=VERTEX_POINT ( 'NONE', #141124 ) ;
#123447=CARTESIAN_POINT ( 'NONE',  ( -11.95360554405576359, 13.60444996502587500, 1.059413164304729538 ) ) ;
#123448=CARTESIAN_POINT ( 'NONE',  ( -11.27970626620888517, 5.059847508428347851, 5.788342990380983544 ) ) ;
#123458=EDGE_LOOP ( 'NONE', ( #169688, #168594, #120371, #178895 ) ) ;
#123459=COLOUR_RGB ( '', 0.09019608, 0.27058824, 0.51372549) ;
#123471=CIRCLE ( 'NONE', #151067, 0.08000000000000040412 ) ;
#123478=CARTESIAN_POINT ( 'NONE',  ( 1.466069532605751007E-15, 14.48154074412737558, 12.00000000000000178 ) ) ;
#123486=CARTESIAN_POINT ( 'NONE',  ( 10.50000000000000178, 10.09159113040219502, -3.600000000000000977 ) ) ;
#123494=EDGE_LOOP ( 'NONE', ( #58317, #124950, #199642, #39194 ) ) ;
#123512=( NAMED_UNIT ( * ) PLANE_ANGLE_UNIT ( ) SI_UNIT ( $, .RADIAN. ) );
#123557=CARTESIAN_POINT ( 'NONE',  ( 11.83077207345802506, 7.766074702148943132, -1.743650018162308912 ) ) ;
#123558=CARTESIAN_POINT ( 'NONE',  ( -1.448815997565382929, 7.903552007303741966, 10.65195286442484424 ) ) ;
#123562=CIRCLE ( 'NONE', #185610, 11.92000000000000171 ) ;
#123587=CARTESIAN_POINT ( 'NONE',  ( -0.04160626335162843220, 15.48012587866529444, 11.99061301703373772 ) ) ;
#123588=CARTESIAN_POINT ( 'NONE',  ( -9.669761313225400556, 3.035266360176858136, 6.558537842936834394 ) ) ;
#123640=CARTESIAN_POINT ( 'NONE',  ( -11.07131242353766254, 12.30000000000000249, -0.8043462106219255725 ) ) ;
#123652=FACE_OUTER_BOUND ( 'NONE', #144440, .T. ) ;
#123675=DIRECTION ( 'NONE',  ( 0.000000000000000000, 1.000000000000000000, 0.000000000000000000 ) ) ;
#123692=AXIS2_PLACEMENT_3D ( 'NONE', #20600, #33665, #52061 ) ;
#123695=CARTESIAN_POINT ( 'NONE',  ( 1.613391111044842492E-15, 14.84205778326404612, 11.68011747745297590 ) ) ;
#123724=CARTESIAN_POINT ( 'NONE',  ( -10.93365108933372198, 4.740440605563193799, -4.433365903526399698 ) ) ;
#123725=AXIS2_PLACEMENT_3D ( 'NONE', #161234, #193721, #45364 ) ;
#123727=CARTESIAN_POINT ( 'NONE',  ( 8.961696533999443659, 14.59015583931033611, 8.974872064516899783 ) ) ;
#123739=DIRECTION ( 'NONE',  ( -0.7806247498001170904, 4.926614671774123060E-13, 0.6249999999996038724 ) ) ;
#123758=AXIS2_PLACEMENT_3D ( 'NONE', #175213, #156824, #6263 ) ;
#123771=CARTESIAN_POINT ( 'NONE',  ( 11.86239285000045740, 13.87999999999998302, 1.812080536912751061 ) ) ;
#123784=ORIENTED_EDGE ( 'NONE', *, *, #141919, .F. ) ;
#123787=EDGE_LOOP ( 'NONE', ( #51638, #195042, #78130, #130282, #54355, #145308, #42936, #60741 ) ) ;
#123796=CARTESIAN_POINT ( 'NONE',  ( 11.41176686791169281, 9.840491965131443308, 3.404018756831826309 ) ) ;
#123797=FILL_AREA_STYLE ('',( #152998 ) ) ;
#123817=EDGE_CURVE ( 'NONE', #3699, #129981, #117248, .T. ) ;
#123836=EDGE_CURVE ( 'NONE', #83914, #181742, #40146, .T. ) ;
#123837=CARTESIAN_POINT ( 'NONE',  ( -11.01135777277262129, 10.90000000000000036, -1.400000000000001910 ) ) ;
#123872=VECTOR ( 'NONE', #113720, 1000.000000000000000 ) ;
#123881=LINE ( 'NONE', #108669, #174992 ) ;
#123898=CARTESIAN_POINT ( 'NONE',  ( -7.120083641305332556, 14.52987117624244284, -9.669683711067579068 ) ) ;
#123905=DIRECTION ( 'NONE',  ( 1.000000000000000000, -0.000000000000000000, -0.000000000000000000 ) ) ;
#123908=B_SPLINE_CURVE_WITH_KNOTS ( 'NONE', 3,
 ( #167768, #138483, #19365, #152580, #203436, #121239, #21480, #18296, #150469, #38838 ),
 .UNSPECIFIED., .F., .F.,
 ( 4, 2, 2, 2, 4 ),
 ( 1.323043618166807713E-09, 0.0004044078111608055909, 0.0008088142992779929433, 0.001213220787395179103, 0.001617627275512365263 ),
 .UNSPECIFIED. ) ;
#123918=AXIS2_PLACEMENT_3D ( 'NONE', #181934, #162524, #146292 ) ;
#123970=CARTESIAN_POINT ( 'NONE',  ( -11.45842088241054668, 13.59306470877032424, 3.566211699757681597 ) ) ;
#123981=CARTESIAN_POINT ( 'NONE',  ( 10.75342306851627328, 8.382369863076769789, 4.797975732338054300 ) ) ;
#123985=CARTESIAN_POINT ( 'NONE',  ( -11.49978884755372555, 9.857291788371918884, -3.429452816445187402 ) ) ;
#123989=ORIENTED_EDGE ( 'NONE', *, *, #143956, .T. ) ;
#124000=DIRECTION ( 'NONE',  ( 0.000000000000000000, 0.000000000000000000, -1.000000000000000000 ) ) ;
#124003=CIRCLE ( 'NONE', #175882, 10.75000000000000000 ) ;
#124035=CARTESIAN_POINT ( 'NONE',  ( -15.75000000000000000, 10.90000000000000036, -3.600000000000002309 ) ) ;
#124038=CYLINDRICAL_SURFACE ( 'NONE', #126567, 0.07999999999999998779 ) ;
#124045=ADVANCED_FACE ( 'NONE', ( #14541 ), #59545, .T. ) ;
#124062=DIRECTION ( 'NONE',  ( 0.000000000000000000, 0.000000000000000000, -1.000000000000000000 ) ) ;
#124080=EDGE_CURVE ( 'NONE', #37826, #96984, #127642, .T. ) ;
#124082=CARTESIAN_POINT ( 'NONE',  ( 7.874658059456543846, 14.91651369936353433, 9.071118931273595365 ) ) ;
#124089=CARTESIAN_POINT ( 'NONE',  ( 9.680359324772703999, 13.43752487939449836, 8.167046318416048223 ) ) ;
#124123=CARTESIAN_POINT ( 'NONE',  ( -11.58085191697663241, 6.132731128919016506, 5.153920277027906671 ) ) ;
#124124=ORIENTED_EDGE ( 'NONE', *, *, #189834, .F. ) ;
#124129=FILL_AREA_STYLE_COLOUR ( '', #180996 ) ;
#124149=CARTESIAN_POINT ( 'NONE',  ( 9.977656983550911463, 11.55331835374545513, 6.672210388449995477 ) ) ;
#124206=CARTESIAN_POINT ( 'NONE',  ( 10.50000000000000178, 10.90000000000000036, -3.600000000000002309 ) ) ;
#124215=EDGE_LOOP ( 'NONE', ( #168297, #85213, #149687, #99800 ) ) ;
#124237=CARTESIAN_POINT ( 'NONE',  ( -10.88586298614011660, 5.812970821470938354, 6.395187734525825896 ) ) ;
#124242=SURFACE_STYLE_USAGE ( .BOTH. , #58080 ) ;
#124287=ORIENTED_EDGE ( 'NONE', *, *, #62427, .T. ) ;
#124305=CARTESIAN_POINT ( 'NONE',  ( 1.250000000000037526, 8.500000000000000000, 11.02939254900286237 ) ) ;
#124311=CARTESIAN_POINT ( 'NONE',  ( -10.21576913194658864, 4.000029896383376027, -7.512182378973799146 ) ) ;
#124373=CARTESIAN_POINT ( 'NONE',  ( 11.33772463945043718, 12.69999999999997264, 3.600000000000075140 ) ) ;
#124382=( LENGTH_UNIT ( ) NAMED_UNIT ( * ) SI_UNIT ( .MILLI., .METRE. ) );
#124387=ORIENTED_EDGE ( 'NONE', *, *, #143394, .T. ) ;
#124402=ORIENTED_EDGE ( 'NONE', *, *, #167734, .F. ) ;
#124411=CARTESIAN_POINT ( 'NONE',  ( -10.79363438595513891, 4.456531630721114468, -5.247043704664541508 ) ) ;
#124414=CARTESIAN_POINT ( 'NONE',  ( -9.372156330827838389, 14.58101807628380264, -7.405769076522356720 ) ) ;
#124417=ORIENTED_EDGE ( 'NONE', *, *, #84764, .F. ) ;
#124429=CARTESIAN_POINT ( 'NONE',  ( 11.44791656467458552, 12.30000000000000071, -3.303228920649581291 ) ) ;
#124480=FACE_OUTER_BOUND ( 'NONE', #138227, .T. ) ;
#124504=CARTESIAN_POINT ( 'NONE',  ( -9.510677803526956353, 3.006766436585398772, 6.782528980676592489 ) ) ;
#124509=CARTESIAN_POINT ( 'NONE',  ( -11.86239285000045918, 11.37999999999999901, -1.812080536912753059 ) ) ;
#124513=VERTEX_POINT ( 'NONE', #91882 ) ;
#124533=CARTESIAN_POINT ( 'NONE',  ( -4.795850251199142988, 15.51848109270388854, -11.00904932811271486 ) ) ;
#124546=CARTESIAN_POINT ( 'NONE',  ( 11.94105721237523277, 10.90000000000000036, -1.187919463087249827 ) ) ;
#124553=CARTESIAN_POINT ( 'NONE',  ( 0.000000000000000000, 4.000000000000002665, 0.000000000000000000 ) ) ;
#124559=CARTESIAN_POINT ( 'NONE',  ( 1.734723475976807094E-15, 14.55305236562695193, 11.95586206896570580 ) ) ;
#124564=FILL_AREA_STYLE_COLOUR ( '', #16262 ) ;
#124582=CARTESIAN_POINT ( 'NONE',  ( 1.446532937691837683E-15, 15.15766726230651606, 11.68000000000000504 ) ) ;
#124601=CARTESIAN_POINT ( 'NONE',  ( -11.33772463945037146, 10.19999999999998153, 3.679999999999999272 ) ) ;
#124604=( BOUNDED_SURFACE ( )  B_SPLINE_SURFACE ( 3, 2, ( 
 ( #136416, #206719, #24765 ),
 ( #138544, #89809, #153722 ),
 ( #106084, #73521, #58347 ),
 ( #72443, #123447, #189409 ),
 ( #158000, #155854, #90867 ),
 ( #107160, #41051, #121298 ) ),
 .UNSPECIFIED., .F., .F., .F. ) 
 B_SPLINE_SURFACE_WITH_KNOTS ( ( 4, 2, 4 ),
 ( 3, 3 ),
 ( 0.000000000000000000, 0.0003754689591423960443, 0.0007509379182847920886 ),
 ( 0.000000000000000000, 1.000000000000000000 ),
 .UNSPECIFIED. ) 
 GEOMETRIC_REPRESENTATION_ITEM ( )  RATIONAL_B_SPLINE_SURFACE ( (
 ( 1.000000000000000000, 0.7071067811865399122, 1.000000000000000000),
 ( 1.000000000000000000, 0.7018599272026960767, 1.000000000000000000),
 ( 1.000000000000000000, 0.6927733177256535368, 1.000000000000000000),
 ( 1.000000000000000000, 0.6772007068877564651, 1.000000000000000000),
 ( 1.000000000000000000, 0.6709974581634203794, 1.000000000000000000),
 ( 1.000000000000000000, 0.6711954675835395401, 1.000000000000000000) ) ) 
 REPRESENTATION_ITEM ( '' )  SURFACE ( )  );
#124616=DIRECTION ( 'NONE',  ( -0.000000000000000000, -1.000000000000000000, -0.000000000000000000 ) ) ;
#124653=UNCERTAINTY_MEASURE_WITH_UNIT (LENGTH_MEASURE( 1.000000000000000082E-05 ), #205548, 'distance_accuracy_value', 'NONE');
#124667=ORIENTED_EDGE ( 'NONE', *, *, #6610, .T. ) ;
#124675=VECTOR ( 'NONE', #95541, 1000.000000000000000 ) ;
#124684=DIRECTION ( 'NONE',  ( 0.000000000000000000, 1.000000000000000000, 0.000000000000000000 ) ) ;
#124696=CARTESIAN_POINT ( 'NONE',  ( -5.540667111194848893, 14.48160243150212523, 10.65389079987404486 ) ) ;
#124710=CARTESIAN_POINT ( 'NONE',  ( 11.88235317400313917, 13.75664239773029962, 0.9089793033029933689 ) ) ;
#124732=CARTESIAN_POINT ( 'NONE',  ( 10.50000000000000355, 13.50718427492792983, 3.599999999999998312 ) ) ;
#124743=DIRECTION ( 'NONE',  ( 0.9632918427306595976, 0.000000000000000000, -0.2684563758389253985 ) ) ;
#124764=CARTESIAN_POINT ( 'NONE',  ( 10.50000000000000178, 13.40000000000000036, -3.600000000000002309 ) ) ;
#124765=CARTESIAN_POINT ( 'NONE',  ( -11.84101807917483740, 9.989784997391225829, -1.444039656437080099 ) ) ;
#124767=CARTESIAN_POINT ( 'NONE',  ( -11.92050416151432835, 13.65205375279624356, -1.381922468431411088 ) ) ;
#124791=CARTESIAN_POINT ( 'NONE',  ( -11.86145017031081217, 10.09418046486151077, -1.100000000000000533 ) ) ;
#124800=ORIENTED_EDGE ( 'NONE', *, *, #120795, .T. ) ;
#124804=DIRECTION ( 'NONE',  ( 0.2684563758389304500, -5.821219718043054220E-15, -0.9632918427306581544 ) ) ;
#124826=SURFACE_STYLE_USAGE ( .BOTH. , #29383 ) ;
#124843=CARTESIAN_POINT ( 'NONE',  ( -11.94654170777226021, 12.44825673841064173, 1.134972293687618539 ) ) ;
#124853=AXIS2_PLACEMENT_3D ( 'NONE', #109596, #62891, #175602 ) ;
#124865=VERTEX_POINT ( 'NONE', #93489 ) ;
#124871=MECHANICAL_DESIGN_GEOMETRIC_PRESENTATION_REPRESENTATION('',(#190472),#93734);
#124882=ORIENTED_EDGE ( 'NONE', *, *, #187512, .F. ) ;
#124891=DIRECTION ( 'NONE',  ( 0.000000000000000000, 1.485208455459594811E-16, -1.000000000000000000 ) ) ;
#124892=ORIENTED_EDGE ( 'NONE', *, *, #13749, .F. ) ;
#124908=CARTESIAN_POINT ( 'NONE',  ( -9.898321827453750998, 15.00000000001253753, -7.924999999985899990 ) ) ;
#124924=AXIS2_PLACEMENT_3D ( 'NONE', #180564, #3912, #49500 ) ;
#124933=EDGE_LOOP ( 'NONE', ( #170736, #119328, #103640, #27761 ) ) ;
#124950=ORIENTED_EDGE ( 'NONE', *, *, #12835, .T. ) ;
#124954=CARTESIAN_POINT ( 'NONE',  ( -10.44369633504468631, 5.112959841837461994, -5.232137017608345708 ) ) ;
#124966=VERTEX_POINT ( 'NONE', #143324 ) ;
#124971=LINE ( 'NONE', #207192, #35433 ) ;
#125021=ORIENTED_EDGE ( 'NONE', *, *, #110409, .T. ) ;
#125033=CARTESIAN_POINT ( 'NONE',  ( -11.44779963594995564, 13.39999999999999147, 3.600000000000075140 ) ) ;
#125046=CARTESIAN_POINT ( 'NONE',  ( 8.994968294694656308, 12.46332533355852590, 7.469580661692561740 ) ) ;
#125052=ORIENTED_EDGE ( 'NONE', *, *, #60132, .T. ) ;
#125062=CARTESIAN_POINT ( 'NONE',  ( 9.367496997597591246, 3.530917816115240360, -7.500000000000005329 ) ) ;
#125090=CARTESIAN_POINT ( 'NONE',  ( 11.92619526913699879, 12.69999999999999929, -1.328859060402686199 ) ) ;
#125103=CARTESIAN_POINT ( 'NONE',  ( -3.501245407925490216, 15.00000000000010658, 11.28115623562641900 ) ) ;
#125144=CARTESIAN_POINT ( 'NONE',  ( 11.88429252019798632, 7.170827761689094970, -1.886747465692856451 ) ) ;
#125150=CARTESIAN_POINT ( 'NONE',  ( 9.504385499323440456, 15.23678955516845868, 8.235007229972609366 ) ) ;
#125168=CARTESIAN_POINT ( 'NONE',  ( 11.94980361490430099, 10.09667875264134551, 1.099999952233555955 ) ) ;
#125180=CARTESIAN_POINT ( 'NONE',  ( -12.15057777967900243, 9.234859088329544718, 2.778757836088345812 ) ) ;
#125256=CARTESIAN_POINT ( 'NONE',  ( -9.361942704757909794, 14.57097479506862037, -7.422992708136343154 ) ) ;
#125263=CARTESIAN_POINT ( 'NONE',  ( 0.05083690440159209512, 14.51152975025495806, 11.99422659986761808 ) ) ;
#125264=CARTESIAN_POINT ( 'NONE',  ( 11.97181073603049484, 11.38000000000000078, 0.8318477717169575625 ) ) ;
#125270=PRESENTATION_STYLE_ASSIGNMENT (( #206423 ) ) ;
#125280=ORIENTED_EDGE ( 'NONE', *, *, #119318, .F. ) ;
#125283=VECTOR ( 'NONE', #162957, 1000.000000000000000 ) ;
#125287=FILL_AREA_STYLE ('',( #59129 ) ) ;
#125288=ADVANCED_FACE ( 'NONE', ( #163814, #115113 ), #16454, .F. ) ;
#125297=CARTESIAN_POINT ( 'NONE',  ( -11.03396297008821847, 6.349565552376400746, 6.086320354413141231 ) ) ;
#125301=( NAMED_UNIT ( * ) SI_UNIT ( $, .STERADIAN. ) SOLID_ANGLE_UNIT ( ) );
#125311=ORIENTED_EDGE ( 'NONE', *, *, #168278, .T. ) ;
#125323=VERTEX_POINT ( 'NONE', #162751 ) ;
#125365=CARTESIAN_POINT ( 'NONE',  ( -9.949604414185204249, 5.483733089116166859, -6.039292150722699759 ) ) ;
#125439=TOROIDAL_SURFACE ( 'NONE', #4246, 12.17999999982603399, 0.5000000000000008882 ) ;
#125442=FILL_AREA_STYLE_COLOUR ( '', #33971 ) ;
#125468=CARTESIAN_POINT ( 'NONE',  ( 9.281668279142875733, 11.48512158433666386, 7.535354720287775088 ) ) ;
#125477=CARTESIAN_POINT ( 'NONE',  ( -5.633484485803696096, 15.51846582102598227, 10.60471134310094321 ) ) ;
#125563=CARTESIAN_POINT ( 'NONE',  ( 9.703911172298809618, 13.32558040432908619, 8.137536601084995880 ) ) ;
#125565=CARTESIAN_POINT ( 'NONE',  ( -10.83017591827266557, 4.360326817186668258, 4.636531744782178777 ) ) ;
#125581=LINE ( 'NONE', #88746, #92277 ) ;
#125608=B_SPLINE_CURVE_WITH_KNOTS ( 'NONE', 3,
 ( #27336, #68347, #115059, #184239, #198354, #119319 ),
 .UNSPECIFIED., .F., .F.,
 ( 4, 2, 4 ),
 ( 0.000000000000000000, 0.0003157158648874033901, 0.0006314317297748067801 ),
 .UNSPECIFIED. ) ;
#125619=CARTESIAN_POINT ( 'NONE',  ( -0.8965205372419083885, 14.55264382554858038, 11.93046248445855007 ) ) ;
#125621=EDGE_CURVE ( 'NONE', #149864, #144610, #122257, .T. ) ;
#125626=CARTESIAN_POINT ( 'NONE',  ( 9.574755873860459232, 4.231292704880496025, 7.158835545600457095 ) ) ;
#125668=ORIENTED_EDGE ( 'NONE', *, *, #136122, .T. ) ;
#125673=CARTESIAN_POINT ( 'NONE',  ( -9.569358774149646862, 4.446947634372958369, 7.167287524840457280 ) ) ;
#125674=LINE ( 'NONE', #7553, #56021 ) ;
#125681=EDGE_CURVE ( 'NONE', #10371, #83814, #147450, .T. ) ;
#125687=VERTEX_POINT ( 'NONE', #157161 ) ;
#125697=CARTESIAN_POINT ( 'NONE',  ( 11.84668730067608244, 10.90000000000000036, -1.320000000000001616 ) ) ;
#125708=CARTESIAN_POINT ( 'NONE',  ( -10.10575425844435138, 4.358269247758318699, 5.859476710806498900 ) ) ;
#125728=EDGE_LOOP ( 'NONE', ( #76003, #131636, #81408, #32621 ) ) ;
#125755=EDGE_CURVE ( 'NONE', #213959, #150697, #134824, .T. ) ;
#125760=CARTESIAN_POINT ( 'NONE',  ( -3.448037578273754011, 14.48027471475642081, 11.50286700577156651 ) ) ;
#125772=SURFACE_STYLE_USAGE ( .BOTH. , #91077 ) ;
#125781=CARTESIAN_POINT ( 'NONE',  ( -11.84668730067608600, 10.89999999999998259, 1.319999999999998286 ) ) ;
#125796=CARTESIAN_POINT ( 'NONE',  ( 0.000000000000000000, 11.37999999999999901, 0.000000000000000000 ) ) ;
#125808=CARTESIAN_POINT ( 'NONE',  ( -11.52463353791760348, 11.38000000000000078, -3.346594096177641475 ) ) ;
#125832=CARTESIAN_POINT ( 'NONE',  ( -11.91292854676703605, 13.61481529673005397, -1.446370920797322102 ) ) ;
#125837=AXIS2_PLACEMENT_3D ( 'NONE', #192243, #12428, #208490 ) ;
#125846=PRESENTATION_STYLE_ASSIGNMENT (( #5570 ) ) ;
#125847=CARTESIAN_POINT ( 'NONE',  ( -9.868259782058050433, 3.553064995558723904, -6.768212174838916795 ) ) ;
#125853=FACE_OUTER_BOUND ( 'NONE', #138672, .T. ) ;
#125894=AXIS2_PLACEMENT_3D ( 'NONE', #8053, #74142, #155382 ) ;
#125897=CARTESIAN_POINT ( 'NONE',  ( 8.767237390769398786, 13.41519500316246116, 8.126379486628986015 ) ) ;
#125943=EDGE_CURVE ( 'NONE', #22427, #108500, #43716, .T. ) ;
#125958=CARTESIAN_POINT ( 'NONE',  ( 9.338271064545565991, 13.87258202181963362, 7.537100060026529214 ) ) ;
#125961=SURFACE_STYLE_USAGE ( .BOTH. , #157324 ) ;
#125962=EDGE_CURVE ( 'NONE', #21587, #28791, #73757, .T. ) ;
#126008=CARTESIAN_POINT ( 'NONE',  ( 11.44779965693276225, 10.99686076798702317, 3.599999932275867121 ) ) ;
#126023=CARTESIAN_POINT ( 'NONE',  ( 0.000000000000000000, 15.00000000000000000, 0.000000000000000000 ) ) ;
#126026=DIRECTION ( 'NONE',  ( 2.078337502098293044E-13, 0.000000000000000000, -1.000000000000000000 ) ) ;
#126058=FILL_AREA_STYLE_COLOUR ( '', #93998 ) ;
#126088=CARTESIAN_POINT ( 'NONE',  ( 11.28392429091624649, 8.882752594160487902, 4.087434772561983287 ) ) ;
#126107=CARTESIAN_POINT ( 'NONE',  ( 8.368688605668825886, 13.06099974637745298, -8.528945119623642768 ) ) ;
#126121=LINE ( 'NONE', #45879, #14810 ) ;
#126165=CARTESIAN_POINT ( 'NONE',  ( 1.000000047849772367, 16.00000000000000711, 11.64874984998672325 ) ) ;
#126170=DIRECTION ( 'NONE',  ( 1.000000000000000000, -0.000000000000000000, -0.000000000000000000 ) ) ;
#126185=( NAMED_UNIT ( * ) PLANE_ANGLE_UNIT ( ) SI_UNIT ( $, .RADIAN. ) );
#126194=FILL_AREA_STYLE ('',( #60041 ) ) ;
#126197=CIRCLE ( 'NONE', #171095, 0.07999999999999933553 ) ;
#126207=CARTESIAN_POINT ( 'NONE',  ( -10.09116860393517534, 4.085811977184856225, -6.504559477715052829 ) ) ;
#126214=CARTESIAN_POINT ( 'NONE',  ( 7.319456789301566957, 16.00157973104908393, 10.35127506063409264 ) ) ;
#126250=CARTESIAN_POINT ( 'NONE',  ( -11.34342368903357290, 5.311043228906556557, 5.661199053045820051 ) ) ;
#126259=EDGE_CURVE ( 'NONE', #116165, #14896, #113035, .T. ) ;
#126264=SURFACE_STYLE_USAGE ( .BOTH. , #129469 ) ;
#126276=CARTESIAN_POINT ( 'NONE',  ( 11.33572747117623791, 8.723673349139550837, 3.942066673117861519 ) ) ;
#126321=CARTESIAN_POINT ( 'NONE',  ( -11.13909472336046136, 5.782604485667383720, 4.477913003530919589 ) ) ;
#126323=EDGE_CURVE ( 'NONE', #37173, #4671, #140671, .T. ) ;
#126348=COLOUR_RGB ( '', 0.09019608, 0.27058824, 0.51372549) ;
#126363=CARTESIAN_POINT ( 'NONE',  ( -9.979842676043658045, 5.589819607760295739, 5.978770845575332338 ) ) ;
#126366=ORIENTED_EDGE ( 'NONE', *, *, #19563, .T. ) ;
#126386=AXIS2_PLACEMENT_3D ( 'NONE', #68435, #167034, #183269 ) ;
#126407=STYLED_ITEM ( 'NONE', ( #111738 ), #135185 ) ;
#126412=ORIENTED_EDGE ( 'NONE', *, *, #144259, .T. ) ;
#126429=SURFACE_STYLE_FILL_AREA ( #128571 ) ;
#126434=CARTESIAN_POINT ( 'NONE',  ( -10.14898710519052649, 3.000029897349846930, -7.601419320309957151 ) ) ;
#126450=DIRECTION ( 'NONE',  ( -0.000000000000000000, -1.000000000000000000, -0.000000000000000000 ) ) ;
#126474=CARTESIAN_POINT ( 'NONE',  ( 11.97929049433705373, 12.22000000000000064, 0.7046979865771783036 ) ) ;
#126501=CARTESIAN_POINT ( 'NONE',  ( 11.70084472423419797, 7.007359388644037068, -2.672842359620002384 ) ) ;
#126503=STYLED_ITEM ( 'NONE', ( #52587 ), #121375 ) ;
#126508=MECHANICAL_DESIGN_GEOMETRIC_PRESENTATION_REPRESENTATION('',(#212833),#150555);
#126509=EDGE_CURVE ( 'NONE', #211752, #19657, #189173, .T. ) ;
#126539=DIRECTION ( 'NONE',  ( -0.5773502691896091887, 0.000000000000000000, 0.8164965809277375808 ) ) ;
#126554=CARTESIAN_POINT ( 'NONE',  ( 8.927850118614284014, 14.71571904887444049, -8.019635469902768321 ) ) ;
#126556=CARTESIAN_POINT ( 'NONE',  ( 11.33772463945036968, 12.59097530385349728, -3.600000000000000977 ) ) ;
#126567=AXIS2_PLACEMENT_3D ( 'NONE', #156459, #40577, #155375 ) ;
#126576=DIRECTION ( 'NONE',  ( 1.598721155460225418E-14, 0.000000000000000000, 1.000000000000000000 ) ) ;
#126620=CARTESIAN_POINT ( 'NONE',  ( 11.91826849282518630, 13.39999999999998259, 1.399999999999996581 ) ) ;
#126625=CARTESIAN_POINT ( 'NONE',  ( 9.808998241650231265, 12.88675894182173387, 8.003755498086194464 ) ) ;
#126655=CARTESIAN_POINT ( 'NONE',  ( -10.33433454857960321, 4.766519530047388820, -5.444264161973041638 ) ) ;
#126669=CARTESIAN_POINT ( 'NONE',  ( 11.94105721237522921, 11.02740784401788865, -1.187919463087249605 ) ) ;
#126670=FILL_AREA_STYLE_COLOUR ( '', #26264 ) ;
#126683=CARTESIAN_POINT ( 'NONE',  ( -7.093286029333435216, 14.55189876998235832, 9.634085594043046541 ) ) ;
#126690=CARTESIAN_POINT ( 'NONE',  ( 9.476364169157013961, 3.602179700984872390, 7.289721614627932667 ) ) ;
#126737=ORIENTED_EDGE ( 'NONE', *, *, #148914, .F. ) ;
#126753=ORIENTED_EDGE ( 'NONE', *, *, #128643, .T. ) ;
#126765=EDGE_CURVE ( 'NONE', #116972, #72298, #88851, .T. ) ;
#126768=DIRECTION ( 'NONE',  ( 1.000000000000000000, -0.000000000000000000, -0.000000000000000000 ) ) ;
#126831=DIRECTION ( 'NONE',  ( 0.9982742078614211811, 0.000000000000000000, -0.05872483221476467591 ) ) ;
#126850=CARTESIAN_POINT ( 'NONE',  ( 11.94105721237523277, 19.00000000000000000, 1.187919463087248273 ) ) ;
#126866=ORIENTED_EDGE ( 'NONE', *, *, #114896, .F. ) ;
#126900=CARTESIAN_POINT ( 'NONE',  ( -11.88156762547253997, 13.87999991545968292, -1.686557021358706443 ) ) ;
#126919=CARTESIAN_POINT ( 'NONE',  ( -11.33772463945037146, 10.19999999999998153, 3.599999999999999201 ) ) ;
#126932=CARTESIAN_POINT ( 'NONE',  ( 11.94105721839851952, 12.57301656658866662, 1.187919402540718927 ) ) ;
#126942=CARTESIAN_POINT ( 'NONE',  ( -11.44779965693221335, 13.49686076798708889, -3.599999932276612746 ) ) ;
#126966=DIRECTION ( 'NONE',  ( -0.000000000000000000, -1.000000000000000000, -0.000000000000000000 ) ) ;
#126979=ADVANCED_FACE ( 'NONE', ( #31893 ), #5734, .T. ) ;
#126995=CARTESIAN_POINT ( 'NONE',  ( 11.84668729035180590, 11.00518580017410386, -1.400000000000001688 ) ) ;
#127007=ORIENTED_EDGE ( 'NONE', *, *, #147272, .F. ) ;
#127020=VERTEX_POINT ( 'NONE', #69682 ) ;
#127030=CARTESIAN_POINT ( 'NONE',  ( 8.347919278768385354, 15.09740922415466358, 8.560103915482137893 ) ) ;
#127052=ORIENTED_EDGE ( 'NONE', *, *, #58359, .T. ) ;
#127053=ORIENTED_EDGE ( 'NONE', *, *, #161821, .T. ) ;
#127099=CARTESIAN_POINT ( 'NONE',  ( -11.33772463945036968, 13.40000000000000036, -3.600000000000002309 ) ) ;
#127113=SURFACE_STYLE_USAGE ( .BOTH. , #130305 ) ;
#127159=FACE_OUTER_BOUND ( 'NONE', #76685, .T. ) ;
#127162=CARTESIAN_POINT ( 'NONE',  ( 9.502358067502351346, 13.11573065610559574, -7.329361613111205820 ) ) ;
#127165=EDGE_CURVE ( 'NONE', #18470, #19630, #9210, .T. ) ;
#127184=EDGE_CURVE ( 'NONE', #72298, #197365, #73030, .T. ) ;
#127185=CARTESIAN_POINT ( 'NONE',  ( 9.231638989588612176, 10.65826171540251366, -7.829156132265964629 ) ) ;
#127188=VERTEX_POINT ( 'NONE', #104353 ) ;
#127190=ORIENTED_EDGE ( 'NONE', *, *, #113810, .F. ) ;
#127203=DIRECTION ( 'NONE',  ( 1.000000000000000000, -0.000000000000000000, -0.000000000000000000 ) ) ;
#127243=CARTESIAN_POINT ( 'NONE',  ( 0.6674790882334069586, 14.00000000000000533, 11.66566053519463786 ) ) ;
#127244=CARTESIAN_POINT ( 'NONE',  ( -11.86145016429273191, 19.00000000000000000, 1.179999999999997051 ) ) ;
#127254=CIRCLE ( 'NONE', #182493, 0.07999999999999998779 ) ;
#127263=LINE ( 'NONE', #76283, #1092 ) ;
#127288=CARTESIAN_POINT ( 'NONE',  ( 7.861136941706560854, 14.80574585066181825, 8.642037812201863289 ) ) ;
#127312=CARTESIAN_POINT ( 'NONE',  ( -9.410012541129075814, 4.000000000000001776, 6.919867902370715917 ) ) ;
#127313=( NAMED_UNIT ( * ) PLANE_ANGLE_UNIT ( ) SI_UNIT ( $, .RADIAN. ) );
#127323=CARTESIAN_POINT ( 'NONE',  ( -12.26673246283585961, 6.254089313302478637, -3.851195297204758727 ) ) ;
#127340=CARTESIAN_POINT ( 'NONE',  ( -9.367496997601303832, 14.53091781611831479, 7.499999999995374367 ) ) ;
#127348=CARTESIAN_POINT ( 'NONE',  ( 11.80555752044661944, 7.909119009004187184, 2.191159464515625821 ) ) ;
#127404=CARTESIAN_POINT ( 'NONE',  ( -11.95482478513894087, 9.001061590107186206, -0.6098180090666859288 ) ) ;
#127426=CIRCLE ( 'NONE', #175747, 12.00000000000000178 ) ;
#127428=DIRECTION ( 'NONE',  ( 0.000000000000000000, 0.000000000000000000, -1.000000000000000000 ) ) ;
#127439=CARTESIAN_POINT ( 'NONE',  ( -12.93484866278744150, 7.732355869717920882, 1.092763313629060873 ) ) ;
#127459=DIRECTION ( 'NONE',  ( -0.000000000000000000, -0.000000000000000000, -1.000000000000000000 ) ) ;
#127491=ORIENTED_EDGE ( 'NONE', *, *, #93697, .T. ) ;
#127497=DIRECTION ( 'NONE',  ( 1.000000000000000000, -0.000000000000000000, -0.000000000000000000 ) ) ;
#127506=( GEOMETRIC_REPRESENTATION_CONTEXT ( 3 ) GLOBAL_UNCERTAINTY_ASSIGNED_CONTEXT ( ( #168477 ) ) GLOBAL_UNIT_ASSIGNED_CONTEXT ( ( #97201, #1774, #129766 ) ) REPRESENTATION_CONTEXT ( 'NONE', 'WORKASPACE' ) );
#127522=( NAMED_UNIT ( * ) SI_UNIT ( $, .STERADIAN. ) SOLID_ANGLE_UNIT ( ) );
#127570=ORIENTED_EDGE ( 'NONE', *, *, #76439, .T. ) ;
#127595=FACE_OUTER_BOUND ( 'NONE', #190694, .T. ) ;
#127611=DIRECTION ( 'NONE',  ( 0.000000000000000000, -1.000000000000000000, 0.000000000000000000 ) ) ;
#127613=CARTESIAN_POINT ( 'NONE',  ( 11.48899393572690997, 7.332171132234710065, 3.320533030897445670 ) ) ;
#127616=( GEOMETRIC_REPRESENTATION_CONTEXT ( 3 ) GLOBAL_UNCERTAINTY_ASSIGNED_CONTEXT ( ( #84021 ) ) GLOBAL_UNIT_ASSIGNED_CONTEXT ( ( #70164, #51822, #132032 ) ) REPRESENTATION_CONTEXT ( 'NONE', 'WORKASPACE' ) );
#127620=CARTESIAN_POINT ( 'NONE',  ( -9.438511317522861432, 14.67479611868992606, -7.309645042966809392 ) ) ;
#127640=CARTESIAN_POINT ( 'NONE',  ( 11.44779964734710909, 10.10189529870395830, 3.599999963171363060 ) ) ;
#127642=B_SPLINE_CURVE_WITH_KNOTS ( 'NONE', 3,
 ( #168275, #70743, #104354, #102210, #4670, #37206 ),
 .UNSPECIFIED., .F., .F.,
 ( 4, 2, 4 ),
 ( 0.000000000000000000, 0.0003778774010236168619, 0.0007557548020472337237 ),
 .UNSPECIFIED. ) ;
#127652=CARTESIAN_POINT ( 'NONE',  ( 7.471610726854514439, 15.41851326508443165, -9.339756462365158995 ) ) ;
#127669=COLOUR_RGB ( '', 0.66274510, 0.83137255, 0.94901961) ;
#127672=ORIENTED_EDGE ( 'NONE', *, *, #156042, .F. ) ;
#127684=EDGE_CURVE ( 'NONE', #154122, #191521, #98761, .T. ) ;
#127689=CARTESIAN_POINT ( 'NONE',  ( -11.48243876534946217, 9.799999999999982947, 3.199999999999997957 ) ) ;
#127699=CARTESIAN_POINT ( 'NONE',  ( 11.89317557362561217, 13.76275843837575152, 1.599935658895948576 ) ) ;
#127704=CARTESIAN_POINT ( 'NONE',  ( 10.20276969027985992, 13.21904656514576004, -7.144040684766732596 ) ) ;
#127714=SURFACE_SIDE_STYLE ('',( #129834 ) ) ;
#127750=CARTESIAN_POINT ( 'NONE',  ( -9.608224290795256195, 15.11803043437814331, -7.189021211466465999 ) ) ;
#127753=B_SPLINE_CURVE_WITH_KNOTS ( 'NONE', 3,
 ( #171545, #208303, #179038, #75126, #159572, #42648, #26357, #145508, #160640, #28507, #92473, #126088, #144438, #30657, #58870, #11170, #193134, #128238, #12240, #158512, #10111, #143363, #61005, #207244, #43712, #63143, #27432, #76184, #45847, #157457, #142292, #161724, #44782, #78314, #174782, #209360, #127162, #59933 ),
 .UNSPECIFIED., .F., .F.,
 ( 4, 2, 2, 2, 2, 2, 2, 2, 2, 2, 2, 2, 2, 2, 2, 2, 2, 2, 4 ),
 ( 1.734723475976806517E-18, 0.001334241201257017244, 0.002668482402514032754, 0.004002723603771048480, 0.005336964805028063773, 0.006004085405656572720, 0.006671206006285081667, 0.008005447207542100430, 0.009339688408799118324, 0.01067392961005613622, 0.01134105021068464170, 0.01200817081131315064, 0.01334241201257016854, 0.01467665321382718990, 0.01601089441508420780, 0.01734513561634122916, 0.01867937681759824706, 0.02001361801885526842, 0.02134785922011228632 ),
 .UNSPECIFIED. ) ;
#127758=VERTEX_POINT ( 'NONE', #140821 ) ;
#127760=DIRECTION ( 'NONE',  ( 0.000000000000000000, 1.000000000000000000, 0.000000000000000000 ) ) ;
#127772=CARTESIAN_POINT ( 'NONE',  ( 9.348761378620915607, 13.52553930298125096, -7.449808453853658641 ) ) ;
#127778=( NAMED_UNIT ( * ) PLANE_ANGLE_UNIT ( ) SI_UNIT ( $, .RADIAN. ) );
#127781=CARTESIAN_POINT ( 'NONE',  ( -10.79203373075640116, 4.452925688118183345, 5.250250085790691301 ) ) ;
#127823=( NAMED_UNIT ( * ) PLANE_ANGLE_UNIT ( ) SI_UNIT ( $, .RADIAN. ) );
#127849=CARTESIAN_POINT ( 'NONE',  ( -9.386220699155614966, 14.48154074412966175, 7.476614104249496684 ) ) ;
#127857=CARTESIAN_POINT ( 'NONE',  ( 0.004084906056917469129, 14.55754942065380320, 11.94689476429229202 ) ) ;
#127914=CARTESIAN_POINT ( 'NONE',  ( 0.000000000000000000, 12.30000000000000071, 0.000000000000000000 ) ) ;
#127917=FACE_OUTER_BOUND ( 'NONE', #140775, .T. ) ;
#127919=ORIENTED_EDGE ( 'NONE', *, *, #171659, .F. ) ;
#127920=EDGE_CURVE ( 'NONE', #18446, #158767, #123562, .T. ) ;
#127924=AXIS2_PLACEMENT_3D ( 'NONE', #75062, #7906, #88113 ) ;
#127945=CARTESIAN_POINT ( 'NONE',  ( 11.91292854676714974, 11.11481529673021207, 1.446370920797324100 ) ) ;
#127947=DIRECTION ( 'NONE',  ( 0.000000000000000000, 0.000000000000000000, -1.000000000000000000 ) ) ;
#127961=( NAMED_UNIT ( * ) PLANE_ANGLE_UNIT ( ) SI_UNIT ( $, .RADIAN. ) );
#127977=CARTESIAN_POINT ( 'NONE',  ( 10.97030574691034843, 12.29999999999998472, 1.695191245859930307 ) ) ;
#127981=DIRECTION ( 'NONE',  ( 0.000000000000000000, 1.000000000000000000, 0.000000000000000000 ) ) ;
#128003=CARTESIAN_POINT ( 'NONE',  ( -11.86145016429273014, 12.69999999999999929, 1.179999999999997051 ) ) ;
#128005=SURFACE_STYLE_USAGE ( .BOTH. , #80214 ) ;
#128020=CARTESIAN_POINT ( 'NONE',  ( 0.000000000000000000, 9.719999999999982876, 0.000000000000000000 ) ) ;
#128040=CARTESIAN_POINT ( 'NONE',  ( 8.445188405616965710, 14.00107259802710047, 8.462322735403144947 ) ) ;
#128049=FACE_OUTER_BOUND ( 'NONE', #164340, .T. ) ;
#128067=AXIS2_PLACEMENT_3D ( 'NONE', #205036, #55607, #72909 ) ;
#128071=CARTESIAN_POINT ( 'NONE',  ( -11.33772463945037146, 12.69999999999998153, 3.599999999999999201 ) ) ;
#128101=UNCERTAINTY_MEASURE_WITH_UNIT (LENGTH_MEASURE( 1.000000000000000082E-05 ), #8072, 'distance_accuracy_value', 'NONE');
#128138=EDGE_CURVE ( 'NONE', #102037, #105543, #141889, .T. ) ;
#128140=CIRCLE ( 'NONE', #121310, 12.00000000000000178 ) ;
#128178=AXIS2_PLACEMENT_3D ( 'NONE', #143483, #211619, #158631 ) ;
#128187=SURFACE_STYLE_FILL_AREA ( #123131 ) ;
#128190=ORIENTED_EDGE ( 'NONE', *, *, #112880, .T. ) ;
#128238=CARTESIAN_POINT ( 'NONE',  ( 11.97505132285663443, 7.681807955339387206, 0.8856721426690242760 ) ) ;
#128244=CARTESIAN_POINT ( 'NONE',  ( -11.78331023100045627, 9.719999999999982876, 1.799999999999999600 ) ) ;
#128246=FACE_OUTER_BOUND ( 'NONE', #106790, .T. ) ;
#128249=ORIENTED_EDGE ( 'NONE', *, *, #82633, .F. ) ;
#128259=CARTESIAN_POINT ( 'NONE',  ( 8.414596756380271714, 12.86228968013755747, 8.493303441398989406 ) ) ;
#128275=CIRCLE ( 'NONE', #124853, 11.92000000000000171 ) ;
#128316=CARTESIAN_POINT ( 'NONE',  ( -1.878313713275644226, 13.99999999999692513, 12.68000002627077905 ) ) ;
#128317=DIRECTION ( 'NONE',  ( 0.000000000000000000, 1.000000000000000000, 0.000000000000000000 ) ) ;
#128344=CARTESIAN_POINT ( 'NONE',  ( -11.89942855770814134, 13.88000000000000078, 0.6999999999999992895 ) ) ;
#128357=CARTESIAN_POINT ( 'NONE',  ( 8.806171940766564177, 13.38206018750110182, -7.684638306840279043 ) ) ;
#128360=CARTESIAN_POINT ( 'NONE',  ( 7.740615115470229846, 13.97676715014342008, 10.04400721814316810 ) ) ;
#128380=CARTESIAN_POINT ( 'NONE',  ( -10.41468459643390254, 5.042717479376880974, -5.872073626459179962 ) ) ;
#128393=CARTESIAN_POINT ( 'NONE',  ( -11.77619280525687451, 4.711391180887883223, -4.977117663154129623 ) ) ;
#128405=( NAMED_UNIT ( * ) SI_UNIT ( $, .STERADIAN. ) SOLID_ANGLE_UNIT ( ) );
#128408=EDGE_CURVE ( 'NONE', #101488, #137788, #15851, .T. ) ;
#128411=CARTESIAN_POINT ( 'NONE',  ( -9.585855168520197367, 15.23438424536737656, 7.219146574778744885 ) ) ;
#128418=CARTESIAN_POINT ( 'NONE',  ( 11.08203335251971744, 9.254633050982178588, 4.606539154764891286 ) ) ;
#128466=CARTESIAN_POINT ( 'NONE',  ( 11.33772463945036790, 10.90000000000000036, -3.600000000000002309 ) ) ;
#128467=CARTESIAN_POINT ( 'NONE',  ( -11.86286653539476177, 7.770451347058147995, 1.827103009650931753 ) ) ;
#128475=CARTESIAN_POINT ( 'NONE',  ( -11.06911165594924462, 7.103609171308002956, -4.638933421456848727 ) ) ;
#128490=ORIENTED_EDGE ( 'NONE', *, *, #105724, .T. ) ;
#128500=EDGE_CURVE ( 'NONE', #53115, #39641, #118791, .T. ) ;
#128506=CARTESIAN_POINT ( 'NONE',  ( -11.33523815116046229, 5.279172990141937305, 5.677742996778201601 ) ) ;
#128509=PRESENTATION_STYLE_ASSIGNMENT (( #213893 ) ) ;
#128513=ORIENTED_EDGE ( 'NONE', *, *, #200040, .T. ) ;
#128526=CARTESIAN_POINT ( 'NONE',  ( 11.52483635780546933, 13.87999991357535201, -3.345866325258015639 ) ) ;
#128538=CIRCLE ( 'NONE', #156144, 0.07999999999999977962 ) ;
#128571=FILL_AREA_STYLE ('',( #208640 ) ) ;
#128576=CARTESIAN_POINT ( 'NONE',  ( -10.83049189199067719, 4.361170120774730208, -4.636001201543571426 ) ) ;
#128616=B_SPLINE_CURVE_WITH_KNOTS ( 'NONE', 3,
 ( #156548, #105683, #70984, #136027, #137097, #186887 ),
 .UNSPECIFIED., .F., .F.,
 ( 4, 2, 4 ),
 ( 0.0006258038130483376113, 0.0009388807108837884767, 0.001251957608719239451 ),
 .UNSPECIFIED. ) ;
#128617=CARTESIAN_POINT ( 'NONE',  ( 11.04536101718726293, 10.90000000000000036, 1.099999999999996758 ) ) ;
#128632=COLOUR_RGB ( '', 0.66274510, 0.83137255, 0.94901961) ;
#128641=CARTESIAN_POINT ( 'NONE',  ( -11.33772463945037146, 19.00000000000000000, 3.679999999999999272 ) ) ;
#128643=EDGE_CURVE ( 'NONE', #51477, #164408, #177465, .T. ) ;
#128671=CARTESIAN_POINT ( 'NONE',  ( 0.000000000000000000, 15.00041888085534758, 0.000000000000000000 ) ) ;
#128673=CARTESIAN_POINT ( 'NONE',  ( 9.070174955424544549, 12.14068019893067429, 7.786856565648018424 ) ) ;
#128691=AXIS2_PLACEMENT_3D ( 'NONE', #186294, #99729, #149548 ) ;
#128699=DIRECTION ( 'NONE',  ( 0.000000000000000000, -0.000000000000000000, 1.000000000000000000 ) ) ;
#128706=( NAMED_UNIT ( * ) PLANE_ANGLE_UNIT ( ) SI_UNIT ( $, .RADIAN. ) );
#128709=CARTESIAN_POINT ( 'NONE',  ( 6.928203230275522984, 15.46908218388476008, -9.797958971132700867 ) ) ;
#128729=COLOUR_RGB ( '', 0.66274510, 0.83137255, 0.94901961) ;
#128733=CARTESIAN_POINT ( 'NONE',  ( -9.949604414185204249, 5.483733089116166859, -6.039292150722699759 ) ) ;
#128741=CARTESIAN_POINT ( 'NONE',  ( -11.94654170777226376, 13.65174326158935969, -1.134972293687621647 ) ) ;
#128747=CARTESIAN_POINT ( 'NONE',  ( 10.38156701084615108, 9.116244165890112328, -6.071958079708653422 ) ) ;
#128748=ADVANCED_FACE ( 'NONE', ( #51612 ), #19081, .F. ) ;
#128757=CARTESIAN_POINT ( 'NONE',  ( 11.96247689755394639, 8.209949295921704859, 0.8094914028917779003 ) ) ;
#128769=CARTESIAN_POINT ( 'NONE',  ( -11.04536101718726293, 13.40000000000000036, 1.099999999999996758 ) ) ;
#128787=ORIENTED_EDGE ( 'NONE', *, *, #208559, .F. ) ;
#128820=AXIS2_PLACEMENT_3D ( 'NONE', #61175, #193305, #194372 ) ;
#128866=SURFACE_STYLE_FILL_AREA ( #193776 ) ;
#128901=DIRECTION ( 'NONE',  ( 0.000000000000000000, 1.000000000000000000, 0.000000000000000000 ) ) ;
#128904=DIRECTION ( 'NONE',  ( 0.000000000000000000, 1.000000000000000000, 0.000000000000000000 ) ) ;
#128927=AXIS2_PLACEMENT_3D ( 'NONE', #42964, #175088, #26676 ) ;
#128965=CARTESIAN_POINT ( 'NONE',  ( 1.500000000000065503, 6.071532165918824830E-15, 10.99818166789400742 ) ) ;
#128967=EDGE_LOOP ( 'NONE', ( #61000, #111316, #20756, #43601 ) ) ;
#128985=VERTEX_POINT ( 'NONE', #104629 ) ;
#128993=AXIS2_PLACEMENT_3D ( 'NONE', #187257, #38884, #58332 ) ;
#128995=AXIS2_PLACEMENT_3D ( 'NONE', #9651, #90932, #41119 ) ;
#129004=ORIENTED_EDGE ( 'NONE', *, *, #60154, .T. ) ;
#129010=AXIS2_PLACEMENT_3D ( 'NONE', #32599, #164730, #16319 ) ;
#129032=CARTESIAN_POINT ( 'NONE',  ( -11.84668729410359411, 13.50620512324532818, -1.400000000000001688 ) ) ;
#129043=FILL_AREA_STYLE ('',( #115953 ) ) ;
#129046=ORIENTED_EDGE ( 'NONE', *, *, #128138, .T. ) ;
#129084=DIRECTION ( 'NONE',  ( -0.000000000000000000, -1.000000000000000000, -0.000000000000000000 ) ) ;
#129092=CIRCLE ( 'NONE', #35591, 0.07999999999999998779 ) ;
#129110=CARTESIAN_POINT ( 'NONE',  ( -9.703135535010517287, 4.518467101586145063, -7.062303484189693670 ) ) ;
#129132=CARTESIAN_POINT ( 'NONE',  ( -11.94650005372637835, 13.65102700337638275, -1.135399707157295435 ) ) ;
#129145=EDGE_CURVE ( 'NONE', #4671, #80885, #111452, .T. ) ;
#129172=COLOUR_RGB ( '', 0.31764706, 0.68627451, 0.89019608) ;
#129231=EDGE_LOOP ( 'NONE', ( #80186, #154470, #198935, #157613 ) ) ;
#129232=( BOUNDED_SURFACE ( )  B_SPLINE_SURFACE ( 3, 2, ( 
 ( #106907, #172932, #140457 ),
 ( #28802, #162014, #48272 ),
 ( #49324, #212861, #47208 ),
 ( #94886, #13603, #14661 ),
 ( #97025, #132724, #148942 ),
 ( #179330, #163079, #80753 ) ),
 .UNSPECIFIED., .F., .F., .T. ) 
 B_SPLINE_SURFACE_WITH_KNOTS ( ( 4, 2, 4 ),
 ( 3, 3 ),
 ( 0.000000000000000000, 0.0003766405729503176413, 0.0007532811459006352826 ),
 ( 0.000000000000000000, 1.000000000000000000 ),
 .UNSPECIFIED. ) 
 GEOMETRIC_REPRESENTATION_ITEM ( )  RATIONAL_B_SPLINE_SURFACE ( (
 ( 1.000000000000000000, 0.7071067811865551223, 1.000000000000000000),
 ( 1.000000000000000000, 0.7211294902953119257, 1.000000000000000000),
 ( 1.000000000000000000, 0.7311181975231312302, 1.000000000000000000),
 ( 1.000000000000000000, 0.7429553055060466038, 1.000000000000000000),
 ( 1.000000000000000000, 0.7451698531059031128, 1.000000000000000000),
 ( 1.000000000000000000, 0.7452309222763021657, 1.000000000000000000) ) ) 
 REPRESENTATION_ITEM ( '' )  SURFACE ( )  );
#129240=CARTESIAN_POINT ( 'NONE',  ( -1.499999999999930278, -6.071532165918824830E-15, 10.99818166789402696 ) ) ;
#129297=EDGE_LOOP ( 'NONE', ( #55009, #10941 ) ) ;
#129310=TOROIDAL_SURFACE ( 'NONE', #125894, 11.92000000000000171, 0.08000000000000000167 ) ;
#129314=( NAMED_UNIT ( * ) SI_UNIT ( $, .STERADIAN. ) SOLID_ANGLE_UNIT ( ) );
#129325=CARTESIAN_POINT ( 'NONE',  ( 9.416996651545288088, 12.55534501603134778, -8.859730546806567020 ) ) ;
#129352=CARTESIAN_POINT ( 'NONE',  ( -11.97297122925984958, 11.29874920673088390, -0.8121202983519461016 ) ) ;
#129374=CARTESIAN_POINT ( 'NONE',  ( -11.55950211276791428, 9.719999999999998863, -3.221476510067114329 ) ) ;
#129377=CARTESIAN_POINT ( 'NONE',  ( 0.3263184169966897308, 15.00000000000058265, 11.67999999558625213 ) ) ;
#129415=EDGE_CURVE ( 'NONE', #120109, #125687, #14798, .T. ) ;
#129417=CARTESIAN_POINT ( 'NONE',  ( -11.99928154390922330, 8.498563086969809888, 1.147813104201464540 ) ) ;
#129421=CARTESIAN_POINT ( 'NONE',  ( 6.743451144134844810, 14.00000000000000000, -9.536680065235829673 ) ) ;
#129424=CARTESIAN_POINT ( 'NONE',  ( 8.350859280846282928, 13.12796858787615584, 8.536646826506956387 ) ) ;
#129456=CARTESIAN_POINT ( 'NONE',  ( -10.99878419127389684, 6.872217442641685103, 3.961452310287494338 ) ) ;
#129469=SURFACE_SIDE_STYLE ('',( #26532 ) ) ;
#129475=CARTESIAN_POINT ( 'NONE',  ( -9.342754679287263997, 14.55305246464195434, 7.460282140107980631 ) ) ;
#129481=EDGE_LOOP ( 'NONE', ( #196368, #188299, #23427, #77058 ) ) ;
#129483=CARTESIAN_POINT ( 'NONE',  ( 11.51809730133723697, 8.398897926204437425, 3.388883170576209913 ) ) ;
#129531=CARTESIAN_POINT ( 'NONE',  ( -11.82159334412768104, 7.677341743419558107, 2.075736564397430151 ) ) ;
#129539=CARTESIAN_POINT ( 'NONE',  ( -10.50059885609812937, 5.377696206510352184, -5.808392519734754345 ) ) ;
#129544=VERTEX_POINT ( 'NONE', #192943 ) ;
#129556=DIRECTION ( 'NONE',  ( 1.776356839400250465E-14, 0.000000000000000000, -1.000000000000000000 ) ) ;
#129566=CARTESIAN_POINT ( 'NONE',  ( -11.78041000490145862, 4.728159582424554586, -4.968671142906706528 ) ) ;
#129573=VERTEX_POINT ( 'NONE', #196165 ) ;
#129583=EDGE_CURVE ( 'NONE', #191009, #173974, #101021, .T. ) ;
#129595=CARTESIAN_POINT ( 'NONE',  ( -7.095284314752811738, 15.44810195178240342, 9.632597271208634737 ) ) ;
#129608=CARTESIAN_POINT ( 'NONE',  ( 9.333041836227135235, 4.446947634373625391, 7.472413793103378943 ) ) ;
#129632=CARTESIAN_POINT ( 'NONE',  ( -11.86145016429273014, 10.19999999999999929, 1.179999999999997051 ) ) ;
#129638=CARTESIAN_POINT ( 'NONE',  ( -10.40063108925089885, 3.507138841238251370, -5.415724211249433040 ) ) ;
#129645=ORIENTED_EDGE ( 'NONE', *, *, #95824, .F. ) ;
#129648=FILL_AREA_STYLE_COLOUR ( '', #112563 ) ;
#129666=AXIS2_PLACEMENT_3D ( 'NONE', #94858, #196606, #31981 ) ;
#129722=ORIENTED_EDGE ( 'NONE', *, *, #425, .F. ) ;
#129732=ORIENTED_EDGE ( 'NONE', *, *, #97488, .F. ) ;
#129738=CARTESIAN_POINT ( 'NONE',  ( 8.837199670533893325, 13.05657914357218274, -8.050043542826816889 ) ) ;
#129741=CARTESIAN_POINT ( 'NONE',  ( 9.348381460497192208, 13.52536904890506797, 7.450314784081282227 ) ) ;
#129757=EDGE_CURVE ( 'NONE', #33851, #81409, #146272, .T. ) ;
#129766=( NAMED_UNIT ( * ) SI_UNIT ( $, .STERADIAN. ) SOLID_ANGLE_UNIT ( ) );
#129817=CARTESIAN_POINT ( 'NONE',  ( 10.88976023856472075, 8.285890218793616313, -4.933575180849306463 ) ) ;
#129826=CARTESIAN_POINT ( 'NONE',  ( 10.14644687988836047, 13.59653676117442878, -7.280050914245562055 ) ) ;
#129827=CARTESIAN_POINT ( 'NONE',  ( -10.37901820579008039, 4.889546506944066451, 5.358714317323078014 ) ) ;
#129834=SURFACE_STYLE_FILL_AREA ( #192597 ) ;
#129857=ADVANCED_FACE ( 'NONE', ( #202520 ), #88668, .T. ) ;
#129861=ORIENTED_EDGE ( 'NONE', *, *, #77449, .F. ) ;
#129868=( LENGTH_UNIT ( ) NAMED_UNIT ( * ) SI_UNIT ( .MILLI., .METRE. ) );
#129909=DIRECTION ( 'NONE',  ( -0.000000000000000000, -1.000000000000000000, -0.000000000000000000 ) ) ;
#129948=CARTESIAN_POINT ( 'NONE',  ( -11.94105721237523277, 19.00000000000000000, 1.187919463087248273 ) ) ;
#129952=AXIS2_PLACEMENT_3D ( 'NONE', #83122, #18112, #84198 ) ;
#129970=CARTESIAN_POINT ( 'NONE',  ( -15.75000000000000000, 10.19999999999998153, 1.799999999999999600 ) ) ;
#129979=DIRECTION ( 'NONE',  ( 0.000000000000000000, 0.000000000000000000, 1.000000000000000000 ) ) ;
#129980=CARTESIAN_POINT ( 'NONE',  ( 11.01135777277261951, 12.59499145469730763, -1.400000000000001243 ) ) ;
#129981=VERTEX_POINT ( 'NONE', #18453 ) ;
#129984=EDGE_CURVE ( 'NONE', #48908, #130487, #204177, .T. ) ;
#130002=DIRECTION ( 'NONE',  ( -0.000000000000000000, 1.000000000000000000, -0.000000000000000000 ) ) ;
#130032=CARTESIAN_POINT ( 'NONE',  ( -15.75000000000000000, 9.799999999999998934, 0.6999999999999992895 ) ) ;
#130086=PRESENTATION_STYLE_ASSIGNMENT (( #43446 ) ) ;
#130088=CARTESIAN_POINT ( 'NONE',  ( -9.333041836230020039, 14.55305236562984383, 7.472413793098202639 ) ) ;
#130096=AXIS2_PLACEMENT_3D ( 'NONE', #141700, #207712, #189330 ) ;
#130101=( LENGTH_UNIT ( ) NAMED_UNIT ( * ) SI_UNIT ( .MILLI., .METRE. ) );
#130113=CARTESIAN_POINT ( 'NONE',  ( 11.86145016429273191, 19.00000000000000000, 1.179999999999997051 ) ) ;
#130131=EDGE_LOOP ( 'NONE', ( #30396, #147073, #168630, #207790, #19667, #65519, #160029, #132721 ) ) ;
#130138=DIRECTION ( 'NONE',  ( -0.9885327375000381167, 0.000000000000000000, -0.1510067114093955609 ) ) ;
#130144=DIRECTION ( 'NONE',  ( 0.000000000000000000, 0.000000000000000000, -1.000000000000000000 ) ) ;
#130164=CARTESIAN_POINT ( 'NONE',  ( -10.44468290228067353, 5.054123846477016180, -5.910681132699941998 ) ) ;
#130166=ORIENTED_EDGE ( 'NONE', *, *, #195119, .F. ) ;
#130184=CARTESIAN_POINT ( 'NONE',  ( -11.52469724861192901, 12.22000006648766934, 3.346365485506925808 ) ) ;
#130195=CARTESIAN_POINT ( 'NONE',  ( -10.51568781791557328, 9.987432697960841210, 3.554797817682051164 ) ) ;
#130200=LINE ( 'NONE', #12097, #554 ) ;
#130204=( BOUNDED_SURFACE ( )  B_SPLINE_SURFACE ( 3, 2, ( 
 ( #22686, #68238, #20563 ),
 ( #38970, #72517, #54154 ),
 ( #69301, #135414, #138613 ),
 ( #86646, #155925, #119210 ),
 ( #201435, #137551, #71439 ),
 ( #70367, #4296, #172178 ) ),
 .UNSPECIFIED., .F., .F., .T. ) 
 B_SPLINE_SURFACE_WITH_KNOTS ( ( 4, 2, 4 ),
 ( 3, 3 ),
 ( 0.000000000000000000, 0.0003754689591423960443, 0.0007509379182847920886 ),
 ( 0.000000000000000000, 1.000000000000000000 ),
 .UNSPECIFIED. ) 
 GEOMETRIC_REPRESENTATION_ITEM ( )  RATIONAL_B_SPLINE_SURFACE ( (
 ( 1.000000000000000000, 0.7071067811865475727, 1.000000000000000000),
 ( 1.000000000000000000, 0.7018599272024074187, 1.000000000000000000),
 ( 1.000000000000000000, 0.6927733177260235742, 1.000000000000000000),
 ( 1.000000000000000000, 0.6772007068873748814, 1.000000000000000000),
 ( 1.000000000000000000, 0.6709974581637080382, 1.000000000000000000),
 ( 1.000000000000000000, 0.6711954675835395401, 1.000000000000000000) ) ) 
 REPRESENTATION_ITEM ( '' )  SURFACE ( )  );
#130220=CARTESIAN_POINT ( 'NONE',  ( 11.89942855770814312, 12.30000000000000071, 0.6999999999999992895 ) ) ;
#130231=EDGE_CURVE ( 'NONE', #187025, #175932, #32138, .T. ) ;
#130241=ORIENTED_EDGE ( 'NONE', *, *, #212713, .F. ) ;
#130282=ORIENTED_EDGE ( 'NONE', *, *, #165199, .T. ) ;
#130288=DIRECTION ( 'NONE',  ( -0.5994789404140892231, 4.843714549364036058E-15, -0.8003905296791067325 ) ) ;
#130305=SURFACE_SIDE_STYLE ('',( #31668 ) ) ;
#130365=DIRECTION ( 'NONE',  ( 1.000000000000000000, 0.000000000000000000, -0.000000000000000000 ) ) ;
#130376=CARTESIAN_POINT ( 'NONE',  ( 9.413505227241941498, 12.55540351140892597, 8.860593473029982903 ) ) ;
#130392=CARTESIAN_POINT ( 'NONE',  ( -11.92619526913699524, 11.02780024161488193, 1.328859060402684866 ) ) ;
#130407=CARTESIAN_POINT ( 'NONE',  ( -11.89197816957260478, 11.29999999999999893, -0.8055420615339585755 ) ) ;
#130424=ADVANCED_FACE ( 'NONE', ( #61 ), #8300, .T. ) ;
#130431=CARTESIAN_POINT ( 'NONE',  ( -11.52460864928265138, 9.719999999999998863, -3.346683403123526190 ) ) ;
#130474=CARTESIAN_POINT ( 'NONE',  ( 7.845839667831243425, 15.84947785439367074, -8.676411862874921610 ) ) ;
#130477=CARTESIAN_POINT ( 'NONE',  ( 8.399612633245173043, 14.34265028463549108, 8.120044275143325052 ) ) ;
#130487=VERTEX_POINT ( 'NONE', #95507 ) ;
#130489=ADVANCED_FACE ( 'NONE', ( #176725 ), #184150, .T. ) ;
#130511=CARTESIAN_POINT ( 'NONE',  ( -11.79409034920973021, 4.782243044590097192, -4.941202808084400822 ) ) ;
#130527=CARTESIAN_POINT ( 'NONE',  ( -9.372067988369742864, 14.58092609327329292, 7.405912380423360197 ) ) ;
#130535=CARTESIAN_POINT ( 'NONE',  ( 11.22634050851384657, 8.811580666534183592, -4.110909495814070169 ) ) ;
#130547=CARTESIAN_POINT ( 'NONE',  ( 11.84668730067608244, 10.09363775091781079, -1.400000000000002132 ) ) ;
#130570=DIRECTION ( 'NONE',  ( -0.000000000000000000, -1.000000000000000000, -0.000000000000000000 ) ) ;
#130573=CARTESIAN_POINT ( 'NONE',  ( -5.580797839525510007, 14.55306906467030181, -10.58276376127103013 ) ) ;
#130584=CARTESIAN_POINT ( 'NONE',  ( -11.86145016429273191, 10.90000000000000036, 1.099999999999996758 ) ) ;
#130585=CARTESIAN_POINT ( 'NONE',  ( -11.82588180490283492, 7.634079919984739782, -2.050956402321635785 ) ) ;
#130589=EDGE_CURVE ( 'NONE', #48908, #209385, #18350, .T. ) ;
#130594=CARTESIAN_POINT ( 'NONE',  ( -10.83006501599620641, 6.402595425522297212, -5.185414522284083283 ) ) ;
#130597=DIRECTION ( 'NONE',  ( 0.000000000000000000, 1.000000000000000000, 0.000000000000000000 ) ) ;
#130614=DIRECTION ( 'NONE',  ( 0.000000000000000000, 0.000000000000000000, 1.000000000000000000 ) ) ;
#130636=ORIENTED_EDGE ( 'NONE', *, *, #131120, .F. ) ;
#130643=B_SPLINE_CURVE_WITH_KNOTS ( 'NONE', 3,
 ( #139674, #25880, #191574, #140755, #187323, #171072 ),
 .UNSPECIFIED., .F., .F.,
 ( 4, 2, 4 ),
 ( 0.0006258038130483376113, 0.0009388807108837884767, 0.001251957608719239451 ),
 .UNSPECIFIED. ) ;
#130649=( NAMED_UNIT ( * ) SI_UNIT ( $, .STERADIAN. ) SOLID_ANGLE_UNIT ( ) );
#130663=EDGE_CURVE ( 'NONE', #133272, #187716, #59807, .T. ) ;
#130672=ORIENTED_EDGE ( 'NONE', *, *, #103048, .F. ) ;
#130695=VERTEX_POINT ( 'NONE', #199338 ) ;
#130700=VECTOR ( 'NONE', #153099, 1000.000000000000000 ) ;
#130711=CARTESIAN_POINT ( 'NONE',  ( -11.92619526913699879, 13.39999999999998259, 1.328859060402682868 ) ) ;
#130761=CARTESIAN_POINT ( 'NONE',  ( -11.07790593930098311, 12.30000000000000071, -0.7000000000000009548 ) ) ;
#130801=EDGE_CURVE ( 'NONE', #29604, #158693, #42667, .T. ) ;
#130808=AXIS2_PLACEMENT_3D ( 'NONE', #166256, #97029, #15726 ) ;
#130815=CARTESIAN_POINT ( 'NONE',  ( 11.92619526913699879, 10.90000000000000036, -1.328859060402686199 ) ) ;
#130824=CARTESIAN_POINT ( 'NONE',  ( 11.86145016429272836, 10.19999999999999929, -1.100000000000000311 ) ) ;
#130847=CARTESIAN_POINT ( 'NONE',  ( 9.534401699824593734, 3.538070456466941849, 7.287265385874707846 ) ) ;
#130868=MECHANICAL_DESIGN_GEOMETRIC_PRESENTATION_REPRESENTATION('',(#96360),#92803);
#130869=PRESENTATION_STYLE_ASSIGNMENT (( #64726 ) ) ;
#130870=CARTESIAN_POINT ( 'NONE',  ( 10.25278263059461636, 12.94063552693930497, 7.030852149930005623 ) ) ;
#130875=ORIENTED_EDGE ( 'NONE', *, *, #50048, .T. ) ;
#130882=CARTESIAN_POINT ( 'NONE',  ( 7.947034306432539275, 14.34752413088959422, -8.932881469798775953 ) ) ;
#130902=ADVANCED_FACE ( 'NONE', ( #85606 ), #170250, .T. ) ;
#130906=CARTESIAN_POINT ( 'NONE',  ( -9.406910906341044765, 14.61725638504506364, 7.349368793364711827 ) ) ;
#130972=EDGE_CURVE ( 'NONE', #4829, #131029, #80684, .T. ) ;
#130986=VERTEX_POINT ( 'NONE', #25932 ) ;
#130996=AXIS2_PLACEMENT_3D ( 'NONE', #113323, #66582, #45074 ) ;
#131028=SURFACE_SIDE_STYLE ('',( #115835 ) ) ;
#131029=VERTEX_POINT ( 'NONE', #172207 ) ;
#131048=AXIS2_PLACEMENT_3D ( 'NONE', #35895, #104113, #188548 ) ;
#131070=ADVANCED_FACE ( 'NONE', ( #9685 ), #189506, .T. ) ;
#131082=CARTESIAN_POINT ( 'NONE',  ( 7.301865417239311817, 14.53770032347495800, 9.470102474007479287 ) ) ;
#131102=CARTESIAN_POINT ( 'NONE',  ( 11.43195036480942051, 12.44475503714742182, -3.649565797774410036 ) ) ;
#131106=DIRECTION ( 'NONE',  ( 0.3162277660168376636, 0.9486832980505138790, 0.000000000000000000 ) ) ;
#131120=EDGE_CURVE ( 'NONE', #183827, #70986, #24863, .T. ) ;
#131122=CARTESIAN_POINT ( 'NONE',  ( 11.92619526913699701, 10.19999999999999929, -1.328859060402686199 ) ) ;
#131158=DIRECTION ( 'NONE',  ( 0.2684563758389304500, 5.821219718043054220E-15, 0.9632918427306581544 ) ) ;
#131163=CARTESIAN_POINT ( 'NONE',  ( -11.04635347860243932, 7.050416898779586106, 4.576031291579900184 ) ) ;
#131174=VERTEX_POINT ( 'NONE', #109405 ) ;
#131176=ORIENTED_EDGE ( 'NONE', *, *, #86952, .F. ) ;
#131206=CARTESIAN_POINT ( 'NONE',  ( 11.94105721237523277, 19.00000000000000000, -1.187919463087249827 ) ) ;
#131208=ORIENTED_EDGE ( 'NONE', *, *, #57012, .T. ) ;
#131214=CARTESIAN_POINT ( 'NONE',  ( -9.976780902586998678, 4.600322429387547984, -6.670003923370737553 ) ) ;
#131223=CARTESIAN_POINT ( 'NONE',  ( 11.41381675112460847, 12.56983264508522602, 3.704697986577264235 ) ) ;
#131233=CARTESIAN_POINT ( 'NONE',  ( -11.97929049433705373, 13.88000000000000078, -0.7046979865771821894 ) ) ;
#131242=ORIENTED_EDGE ( 'NONE', *, *, #19314, .T. ) ;
#131246=SURFACE_STYLE_USAGE ( .BOTH. , #180989 ) ;
#131282=UNCERTAINTY_MEASURE_WITH_UNIT (LENGTH_MEASURE( 1.000000000000000082E-05 ), #177501, 'distance_accuracy_value', 'NONE');
#131287=EDGE_LOOP ( 'NONE', ( #58344, #135804, #133400, #26968 ) ) ;
#131308=EDGE_CURVE ( 'NONE', #84713, #125323, #63362, .T. ) ;
#131309=AXIS2_PLACEMENT_3D ( 'NONE', #14076, #162506, #80166 ) ;
#131333=CARTESIAN_POINT ( 'NONE',  ( 11.45842088241064793, 11.09306470877039885, -3.566211699757709574 ) ) ;
#131338=DIRECTION ( 'NONE',  ( 0.000000000000000000, 0.000000000000000000, 1.000000000000000000 ) ) ;
#131398=CARTESIAN_POINT ( 'NONE',  ( -11.92619526913699879, 10.19999999999999929, -1.328859060402686199 ) ) ;
#131414=CARTESIAN_POINT ( 'NONE',  ( 9.898415338264832997, 12.56653357618227318, -7.886274193477667893 ) ) ;
#131415=ORIENTED_EDGE ( 'NONE', *, *, #54909, .T. ) ;
#131426=ORIENTED_EDGE ( 'NONE', *, *, #27605, .T. ) ;
#131429=CARTESIAN_POINT ( 'NONE',  ( 11.07124251632621537, 12.30000000000000071, -0.8054525327832628978 ) ) ;
#131453=CARTESIAN_POINT ( 'NONE',  ( 11.44791656467458552, 9.800000000000002487, -3.303228920649581291 ) ) ;
#131464=CARTESIAN_POINT ( 'NONE',  ( -11.45681933918879380, 6.923721555720867116, -3.421067468575024417 ) ) ;
#131468=DIRECTION ( 'NONE',  ( 0.000000000000000000, 0.000000000000000000, -1.000000000000000000 ) ) ;
#131496=CARTESIAN_POINT ( 'NONE',  ( -15.75000000000000000, 9.799999999999998934, -1.800000000000001155 ) ) ;
#131510=CARTESIAN_POINT ( 'NONE',  ( 9.998113830209401698, 14.27718261535635058, -7.519171174559423854 ) ) ;
#131542=CARTESIAN_POINT ( 'NONE',  ( -10.91675076000969113, 4.673595418013491987, -4.467283485442433921 ) ) ;
#131555=ADVANCED_FACE ( 'NONE', ( #111529 ), #132952, .T. ) ;
#131564=CARTESIAN_POINT ( 'NONE',  ( -9.417646481151111360, 14.63844056099971347, 7.338279069377040997 ) ) ;
#131565=VERTEX_POINT ( 'NONE', #167678 ) ;
#131603=EDGE_CURVE ( 'NONE', #1299, #31691, #121431, .T. ) ;
#131623=CARTESIAN_POINT ( 'NONE',  ( -11.56423468642480401, 7.060487068201201311, -3.212550277156387857 ) ) ;
#131631=CARTESIAN_POINT ( 'NONE',  ( -11.29536259237624485, 7.646265759024179154, -3.923153468842301983 ) ) ;
#131636=ORIENTED_EDGE ( 'NONE', *, *, #138826, .T. ) ;
#131661=DIRECTION ( 'NONE',  ( 0.000000000000000000, -0.000000000000000000, 1.000000000000000000 ) ) ;
#131664=EDGE_LOOP ( 'NONE', ( #11171, #81544, #69267, #38679 ) ) ;
#131674=ORIENTED_EDGE ( 'NONE', *, *, #63108, .F. ) ;
#131677=SURFACE_STYLE_FILL_AREA ( #160939 ) ;
#131679=CARTESIAN_POINT ( 'NONE',  ( -10.50000000000000000, 12.69999999999998153, 3.599999999999999201 ) ) ;
#131680=CARTESIAN_POINT ( 'NONE',  ( 11.41126283316785361, 13.75874606908454822, -3.405403429622925415 ) ) ;
#131699=EDGE_CURVE ( 'NONE', #49891, #7711, #174095, .T. ) ;
#131727=ORIENTED_EDGE ( 'NONE', *, *, #208458, .F. ) ;
#131773=AXIS2_PLACEMENT_3D ( 'NONE', #8241, #7157, #42912 ) ;
#131793=CARTESIAN_POINT ( 'NONE',  ( -10.44369227015510404, 5.112964020592957404, 5.232143560358708534 ) ) ;
#131813=ORIENTED_EDGE ( 'NONE', *, *, #116113, .T. ) ;
#131858=CARTESIAN_POINT ( 'NONE',  ( 11.97929049433705551, 9.799999999999998934, -0.7046979865771820783 ) ) ;
#131886=CARTESIAN_POINT ( 'NONE',  ( -10.97030176249251276, 11.29999999999998117, 1.695215491223428739 ) ) ;
#131887=CARTESIAN_POINT ( 'NONE',  ( -10.19200560444942560, 4.477620260464512114, -5.707107691925500603 ) ) ;
#131902=CARTESIAN_POINT ( 'NONE',  ( 8.628029272663843230, 13.71747347301596598, -8.342125298644845088 ) ) ;
#131910=CARTESIAN_POINT ( 'NONE',  ( 11.05511614931255160, 7.767163931695388435, -1.611817371847934943 ) ) ;
#131917=B_SPLINE_CURVE_WITH_KNOTS ( 'NONE', 3,
 ( #57741, #142224, #191982, #109764, #107623, #173654 ),
 .UNSPECIFIED., .F., .F.,
 ( 4, 2, 4 ),
 ( 0.000000000000000000, 0.0003157158648874024685, 0.0006314317297748052622 ),
 .UNSPECIFIED. ) ;
#131921=CARTESIAN_POINT ( 'NONE',  ( 8.207694362149334566, 14.14762995341124707, -8.754715811281320370 ) ) ;
#131929=CARTESIAN_POINT ( 'NONE',  ( -11.04536101718726293, 13.50581159806359643, -1.100000000000000311 ) ) ;
#131953=SURFACE_STYLE_USAGE ( .BOTH. , #180659 ) ;
#131969=CARTESIAN_POINT ( 'NONE',  ( 11.07131242353766254, 11.29999999999999893, -0.8043462106219256835 ) ) ;
#131977=EDGE_CURVE ( 'NONE', #175932, #210028, #201496, .T. ) ;
#132002=DIRECTION ( 'NONE',  ( 0.000000000000000000, 0.000000000000000000, 1.000000000000000000 ) ) ;
#132020=CARTESIAN_POINT ( 'NONE',  ( -11.88234649872613602, 9.843392170832489185, 0.9090484974825225883 ) ) ;
#132032=( NAMED_UNIT ( * ) SI_UNIT ( $, .STERADIAN. ) SOLID_ANGLE_UNIT ( ) );
#132068=CARTESIAN_POINT ( 'NONE',  ( 11.01135777277262306, 12.69999999999999929, -1.400000000000001910 ) ) ;
#132126=AXIS2_PLACEMENT_3D ( 'NONE', #36861, #2205, #102945 ) ;
#132131=STYLED_ITEM ( 'NONE', ( #125846 ), #48566 ) ;
#132188=ORIENTED_EDGE ( 'NONE', *, *, #168648, .F. ) ;
#132193=VECTOR ( 'NONE', #130002, 1000.000000000000000 ) ;
#132201=CARTESIAN_POINT ( 'NONE',  ( -11.86145016429273014, 10.19999999999999929, -1.100000000000000533 ) ) ;
#132208=VERTEX_POINT ( 'NONE', #120924 ) ;
#132209=DIRECTION ( 'NONE',  ( -0.000000000000000000, 1.000000000000000000, -0.000000000000000000 ) ) ;
#132210=EDGE_LOOP ( 'NONE', ( #143260, #131242, #92187, #160284 ) ) ;
#132229=CARTESIAN_POINT ( 'NONE',  ( -11.97929049433705373, 13.88000000000000078, 0.7046979865771783036 ) ) ;
#132243=ORIENTED_EDGE ( 'NONE', *, *, #120497, .T. ) ;
#132248=SURFACE_SIDE_STYLE ('',( #36827 ) ) ;
#132268=CARTESIAN_POINT ( 'NONE',  ( -11.94105722165071093, 13.52582762082958823, -1.187919369849417484 ) ) ;
#132276=EDGE_LOOP ( 'NONE', ( #199, #178059, #85880, #134118 ) ) ;
#132287=SURFACE_STYLE_USAGE ( .BOTH. , #185244 ) ;
#132306=EDGE_CURVE ( 'NONE', #99531, #18446, #55841, .T. ) ;
#132320=CARTESIAN_POINT ( 'NONE',  ( 11.84668730067608600, 10.19999999999998153, 1.399999999999998579 ) ) ;
#132326=COLOUR_RGB ( '', 0.72549020, 0.75294118, 0.79215686) ;
#132352=AXIS2_PLACEMENT_3D ( 'NONE', #181149, #113028, #14365 ) ;
#132358=EDGE_CURVE ( 'NONE', #20115, #73634, #163720, .T. ) ;
#132375=LINE ( 'NONE', #118279, #18169 ) ;
#132378=CARTESIAN_POINT ( 'NONE',  ( 11.84104725192634966, 12.49016462548580542, 1.443823348526939165 ) ) ;
#132382=AXIS2_PLACEMENT_3D ( 'NONE', #182038, #81362, #179937 ) ;
#132384=CARTESIAN_POINT ( 'NONE',  ( 1.500000000000065503, 7.750000000000000000, -10.99818166789400919 ) ) ;
#132398=ORIENTED_EDGE ( 'NONE', *, *, #168226, .T. ) ;
#132406=DIRECTION ( 'NONE',  ( -0.000000000000000000, -1.000000000000000000, -0.000000000000000000 ) ) ;
#132416=VERTEX_POINT ( 'NONE', #71328 ) ;
#132417=ORIENTED_EDGE ( 'NONE', *, *, #143084, .T. ) ;
#132428=DIRECTION ( 'NONE',  ( 0.05872483221476467591, -7.952201780260630618E-17, -0.9982742078614211811 ) ) ;
#132436=FACE_OUTER_BOUND ( 'NONE', #4385, .T. ) ;
#132442=DIRECTION ( 'NONE',  ( 1.000000000000000000, -0.000000000000000000, -0.000000000000000000 ) ) ;
#132458=CARTESIAN_POINT ( 'NONE',  ( 0.000000000000000000, 19.00000000000000000, 0.000000000000000000 ) ) ;
#132468=CARTESIAN_POINT ( 'NONE',  ( 8.366200769982176766, 13.06116137083107098, 8.526426475962127327 ) ) ;
#132525=CARTESIAN_POINT ( 'NONE',  ( 11.94105721237523277, 12.69999999999999929, -1.187919463087249827 ) ) ;
#132530=DIRECTION ( 'NONE',  ( -0.5994789404140901112, 2.055006554627987857E-15, 0.8003905296791060664 ) ) ;
#132564=CARTESIAN_POINT ( 'NONE',  ( 7.296230878984865775, 15.96627503840708329, -9.125506818615267690 ) ) ;
#132582=CARTESIAN_POINT ( 'NONE',  ( -10.04321860110356468, 4.586749146271848154, -6.488091244683950265 ) ) ;
#132612=CARTESIAN_POINT ( 'NONE',  ( -9.342889097980298985, 15.44694756379904099, 7.460114341897615908 ) ) ;
#132618=CARTESIAN_POINT ( 'NONE',  ( 1.499999999999961364, 7.750000000000000000, -10.64483442802188762 ) ) ;
#132623=CARTESIAN_POINT ( 'NONE',  ( 11.95360554405587195, 13.60444996502594428, -1.059413164304662924 ) ) ;
#132631=ORIENTED_EDGE ( 'NONE', *, *, #123168, .T. ) ;
#132633=CARTESIAN_POINT ( 'NONE',  ( 11.92619526248524586, 12.57255386085826032, -1.328859120100568170 ) ) ;
#132646=VECTOR ( 'NONE', #126170, 1000.000000000000000 ) ;
#132669=CARTESIAN_POINT ( 'NONE',  ( -11.94980361058168938, 12.70000000000000107, -1.100000000000000311 ) ) ;
#132671=CARTESIAN_POINT ( 'NONE',  ( -11.38926526437179731, 6.532335583446259086, -3.785035105474102934 ) ) ;
#132679=DIRECTION ( 'NONE',  ( -0.9885327375000381167, 0.000000000000000000, 0.1510067114093955609 ) ) ;
#132683=EDGE_CURVE ( 'NONE', #185122, #149864, #30824, .T. ) ;
#132713=EDGE_LOOP ( 'NONE', ( #152801, #149344, #28519, #132871 ) ) ;
#132721=ORIENTED_EDGE ( 'NONE', *, *, #134279, .T. ) ;
#132724=CARTESIAN_POINT ( 'NONE',  ( -11.91826848676304529, 12.59166292761251782, 1.400000051402190637 ) ) ;
#132726=CIRCLE ( 'NONE', #39312, 0.07999999999999998779 ) ;
#132727=CARTESIAN_POINT ( 'NONE',  ( -10.62873463776380056, 13.79999999999999893, -3.200000000000001510 ) ) ;
#132731=MECHANICAL_DESIGN_GEOMETRIC_PRESENTATION_REPRESENTATION('',(#170729),#84300);
#132755=ORIENTED_EDGE ( 'NONE', *, *, #131699, .T. ) ;
#132774=DIRECTION ( 'NONE',  ( -0.000000000000000000, 1.000000000000000000, -0.000000000000000000 ) ) ;
#132843=CARTESIAN_POINT ( 'NONE',  ( 1.050790385994986309, 16.00000000000000711, -12.64745918785790835 ) ) ;
#132845=CARTESIAN_POINT ( 'NONE',  ( -11.21412923722849619, 8.995494058042485364, 2.499828665724475485 ) ) ;
#132859=ORIENTED_EDGE ( 'NONE', *, *, #57116, .T. ) ;
#132865=ORIENTED_EDGE ( 'NONE', *, *, #59183, .T. ) ;
#132871=ORIENTED_EDGE ( 'NONE', *, *, #123262, .F. ) ;
#132880=CARTESIAN_POINT ( 'NONE',  ( 10.50000000000000000, 12.59290055818100562, 3.599999999999996536 ) ) ;
#132891=CYLINDRICAL_SURFACE ( 'NONE', #171914, 0.08000000000000020983 ) ;
#132902=SURFACE_STYLE_FILL_AREA ( #50552 ) ;
#132932=ORIENTED_EDGE ( 'NONE', *, *, #13361, .T. ) ;
#132935=AXIS2_PLACEMENT_3D ( 'NONE', #28086, #44353, #62705 ) ;
#132941=CIRCLE ( 'NONE', #122666, 0.07999999999999946043 ) ;
#132952=( BOUNDED_SURFACE ( )  B_SPLINE_SURFACE ( 3, 2, ( 
 ( #12871, #180722, #152497 ),
 ( #66939, #68008, #182851 ),
 ( #4080, #34470, #134148 ),
 ( #132020, #99483, #135203 ),
 ( #51810, #183922, #35534 ),
 ( #101610, #133081, #50725 ) ),
 .UNSPECIFIED., .F., .F., .F. ) 
 B_SPLINE_SURFACE_WITH_KNOTS ( ( 4, 2, 4 ),
 ( 3, 3 ),
 ( 0.000000000000000000, 0.0003754691837024765901, 0.0007509383674049531802 ),
 ( 0.000000000000000000, 1.000000000000000000 ),
 .UNSPECIFIED. ) 
 GEOMETRIC_REPRESENTATION_ITEM ( )  RATIONAL_B_SPLINE_SURFACE ( (
 ( 1.000000000000000000, 0.6711954675835484219, 1.000000000000000000),
 ( 1.000000000000000000, 0.6709646295267468474, 1.000000000000000000),
 ( 1.000000000000000000, 0.6771840716659200954, 1.000000000000000000),
 ( 1.000000000000000000, 0.6927481755867312962, 1.000000000000000000),
 ( 1.000000000000000000, 0.7017972101310004929, 1.000000000000000000),
 ( 1.000000000000000000, 0.7071067811865475727, 1.000000000000000000) ) ) 
 REPRESENTATION_ITEM ( '' )  SURFACE ( )  );
#132958=CARTESIAN_POINT ( 'NONE',  ( 10.39592987943500724, 9.162555348756470153, 6.046252475528372194 ) ) ;
#132967=VERTEX_POINT ( 'NONE', #141232 ) ;
#132970=CARTESIAN_POINT ( 'NONE',  ( 11.15299978643949252, 7.622798436847911141, 0.8142573934770976907 ) ) ;
#132980=CARTESIAN_POINT ( 'NONE',  ( 7.884034871045744630, 14.36475460829932516, -9.047442571381882459 ) ) ;
#132987=CARTESIAN_POINT ( 'NONE',  ( -11.06298660227979802, 13.75680399625266759, -0.9087478855431304625 ) ) ;
#132995=PRESENTATION_STYLE_ASSIGNMENT (( #165455 ) ) ;
#133034=EDGE_CURVE ( 'NONE', #52465, #31723, #194931, .T. ) ;
#133035=ORIENTED_EDGE ( 'NONE', *, *, #113819, .T. ) ;
#133060=ADVANCED_FACE ( 'NONE', ( #127159 ), #44779, .T. ) ;
#133062=EDGE_LOOP ( 'NONE', ( #227, #26178, #70461, #188347 ) ) ;
#133074=B_SPLINE_CURVE_WITH_KNOTS ( 'NONE', 3,
 ( #183358, #48066, #17634, #51236, #83719, #81595, #147680, #149809, #117360, #114178, #34963, #150882, #18710, #84794, #2445, #180172, #16571, #68519, #213697, #134646, #151939, #49113, #52300, #118429, #102114, #168183, #85864, #196421 ),
 .UNSPECIFIED., .F., .F.,
 ( 4, 2, 2, 2, 2, 2, 2, 2, 2, 2, 2, 2, 2, 4 ),
 ( 8.673617379884039324E-19, 0.001589606426660063751, 0.002384409639990094001, 0.003179212853320124467, 0.003974016066650155367, 0.004768819279980185399, 0.006358425706640248067, 0.007153228919970278966, 0.007948032133300312468, 0.008742835346630343368, 0.009537638559960374268, 0.01033244177329040690, 0.01112724498662043780, 0.01271685141328049613 ),
 .UNSPECIFIED. ) ;
#133081=CARTESIAN_POINT ( 'NONE',  ( -11.97929049433705551, 9.799999999999998934, 0.7046979865771804130 ) ) ;
#133096=CARTESIAN_POINT ( 'NONE',  ( 11.55950211276791428, 12.21999999999998288, 3.221476510067112109 ) ) ;
#133100=AXIS2_PLACEMENT_3D ( 'NONE', #82618, #199558, #31765 ) ;
#133108=STYLED_ITEM ( 'NONE', ( #213630 ), #186082 ) ;
#133109=CARTESIAN_POINT ( 'NONE',  ( -10.56519166458664039, 11.25908454800986647, -3.404836274859124323 ) ) ;
#133116=DIRECTION ( 'NONE',  ( -0.000000000000000000, -1.000000000000000000, 0.000000000000000000 ) ) ;
#133123=( GEOMETRIC_REPRESENTATION_CONTEXT ( 3 ) GLOBAL_UNCERTAINTY_ASSIGNED_CONTEXT ( ( #35321 ) ) GLOBAL_UNIT_ASSIGNED_CONTEXT ( ( #119191, #203546, #7490 ) ) REPRESENTATION_CONTEXT ( 'NONE', 'WORKASPACE' ) );
#133148=( LENGTH_UNIT ( ) NAMED_UNIT ( * ) SI_UNIT ( .MILLI., .METRE. ) );
#133150=STYLED_ITEM ( 'NONE', ( #43323 ), #86239 ) ;
#133173=DIRECTION ( 'NONE',  ( 0.000000000000000000, 0.000000000000000000, 1.000000000000000000 ) ) ;
#133215=CARTESIAN_POINT ( 'NONE',  ( 11.92619526248524586, 10.07255386085825677, -1.328859120100568170 ) ) ;
#133232=CARTESIAN_POINT ( 'NONE',  ( 9.354067518987882579, 13.88574871644472708, 7.517258212044111154 ) ) ;
#133234=CARTESIAN_POINT ( 'NONE',  ( -9.410012541129075814, 4.000000000000001776, 6.919867902370715917 ) ) ;
#133272=VERTEX_POINT ( 'NONE', #114103 ) ;
#133279=FACE_OUTER_BOUND ( 'NONE', #143061, .T. ) ;
#133288=ADVANCED_FACE ( 'NONE', ( #47987 ), #197995, .F. ) ;
#133293=CARTESIAN_POINT ( 'NONE',  ( 1.292128843000315053, 8.373613470998938269, -10.90074592850030655 ) ) ;
#133299=DIRECTION ( 'NONE',  ( 1.224646799147343346E-16, 0.000000000000000000, -1.000000000000000000 ) ) ;
#133311=ADVANCED_FACE ( 'NONE', ( #164901 ), #35349, .T. ) ;
#133334=CARTESIAN_POINT ( 'NONE',  ( -8.158842082463221956, 15.47018964179058287, 8.845107385697343005 ) ) ;
#133378=FILL_AREA_STYLE_COLOUR ( '', #174788 ) ;
#133400=ORIENTED_EDGE ( 'NONE', *, *, #162616, .T. ) ;
#133412=CARTESIAN_POINT ( 'NONE',  ( -9.386185638452808178, 15.51845904014325406, -7.476657895053266500 ) ) ;
#133420=CARTESIAN_POINT ( 'NONE',  ( -11.94105721237522921, 10.07259609010266388, 1.187919463087244720 ) ) ;
#133440=CARTESIAN_POINT ( 'NONE',  ( -11.86239285000045918, 12.22000000000000064, -1.812080536912753059 ) ) ;
#133468=CARTESIAN_POINT ( 'NONE',  ( -0.4486072944944382579, 15.44705570208638967, -11.94951239051067482 ) ) ;
#133479=( GEOMETRIC_REPRESENTATION_CONTEXT ( 3 ) GLOBAL_UNCERTAINTY_ASSIGNED_CONTEXT ( ( #152796 ) ) GLOBAL_UNIT_ASSIGNED_CONTEXT ( ( #142440, #127313, #177043 ) ) REPRESENTATION_CONTEXT ( 'NONE', 'WORKASPACE' ) );
#133498=CARTESIAN_POINT ( 'NONE',  ( 0.000000000000000000, 15.51845925587262798, 0.000000000000000000 ) ) ;
#133512=CARTESIAN_POINT ( 'NONE',  ( -11.91294103507069480, 9.985399100436019637, -1.446263142085563169 ) ) ;
#133518=CARTESIAN_POINT ( 'NONE',  ( -11.30310531956832776, 5.150576456239970291, 5.742040133384030298 ) ) ;
#133520=SURFACE_STYLE_USAGE ( .BOTH. , #67379 ) ;
#133545=CARTESIAN_POINT ( 'NONE',  ( 11.94105722165070560, 12.57417237917041142, -1.187919369849492757 ) ) ;
#133574=CARTESIAN_POINT ( 'NONE',  ( -11.78331023100045627, 13.88000000000000078, -1.800000000000001155 ) ) ;
#133584=CARTESIAN_POINT ( 'NONE',  ( -10.87107728089202752, 4.495199002972934288, -4.557510466808897043 ) ) ;
#133612=FILL_AREA_STYLE_COLOUR ( '', #104215 ) ;
#133634=CARTESIAN_POINT ( 'NONE',  ( 7.440075190158704110, 14.00000000000000000, -10.26883734974634166 ) ) ;
#133677=ORIENTED_EDGE ( 'NONE', *, *, #173872, .F. ) ;
#133681=DIRECTION ( 'NONE',  ( -1.000000000000000000, 0.000000000000000000, 1.224646799147353207E-16 ) ) ;
#133682=CARTESIAN_POINT ( 'NONE',  ( -9.417400626923768669, 15.36186642319061413, 7.338645109549106316 ) ) ;
#133683=ORIENTED_EDGE ( 'NONE', *, *, #52222, .F. ) ;
#133689=( GEOMETRIC_REPRESENTATION_CONTEXT ( 3 ) GLOBAL_UNCERTAINTY_ASSIGNED_CONTEXT ( ( #164225 ) ) GLOBAL_UNIT_ASSIGNED_CONTEXT ( ( #31959, #15678, #65485 ) ) REPRESENTATION_CONTEXT ( 'NONE', 'WORKASPACE' ) );
#133702=ORIENTED_EDGE ( 'NONE', *, *, #193910, .F. ) ;
#133704=CARTESIAN_POINT ( 'NONE',  ( 11.84668730067608600, 10.19999999999998153, 1.399999999999998579 ) ) ;
#133737=SURFACE_STYLE_USAGE ( .BOTH. , #115382 ) ;
#133749=CARTESIAN_POINT ( 'NONE',  ( -10.63162544082345917, 5.889931872887933295, 5.474679228419857324 ) ) ;
#133752=CIRCLE ( 'NONE', #57497, 0.5000000000000013323 ) ;
#133760=MECHANICAL_DESIGN_GEOMETRIC_PRESENTATION_REPRESENTATION('',(#19612),#36927);
#133795=CARTESIAN_POINT ( 'NONE',  ( -0.07968943112122245376, 15.51761980755981973, 11.99973206010910864 ) ) ;
#133821=VERTEX_POINT ( 'NONE', #191013 ) ;
#133836=( NAMED_UNIT ( * ) SI_UNIT ( $, .STERADIAN. ) SOLID_ANGLE_UNIT ( ) );
#133868=CARTESIAN_POINT ( 'NONE',  ( -11.01135777277262129, 13.40000000000000036, -1.400000000000001910 ) ) ;
#133888=UNCERTAINTY_MEASURE_WITH_UNIT (LENGTH_MEASURE( 1.000000000000000082E-05 ), #81990, 'distance_accuracy_value', 'NONE');
#133917=CARTESIAN_POINT ( 'NONE',  ( -10.71026998871754721, 6.055660674263378951, 4.667787751035539223 ) ) ;
#133929=COLOUR_RGB ( '', 0.31764706, 0.68627451, 0.89019608) ;
#133939=EDGE_LOOP ( 'NONE', ( #167985, #69695, #121644, #115903, #185832, #17908, #60357, #23850 ) ) ;
#133945=ORIENTED_EDGE ( 'NONE', *, *, #81658, .T. ) ;
#133947=LINE ( 'NONE', #68877, #23903 ) ;
#133956=CARTESIAN_POINT ( 'NONE',  ( -11.89942855770814134, 9.799999999999998934, 0.6999999999999992895 ) ) ;
#133986=CARTESIAN_POINT ( 'NONE',  ( 11.88234649872613602, 9.843392170832489185, -0.9090484974825243647 ) ) ;
#134010=ORIENTED_EDGE ( 'NONE', *, *, #20246, .T. ) ;
#134015=CARTESIAN_POINT ( 'NONE',  ( -10.33433454857960321, 4.766519530047388820, -5.444264161973041638 ) ) ;
#134025=SURFACE_STYLE_FILL_AREA ( #5019 ) ;
#134032=CARTESIAN_POINT ( 'NONE',  ( 10.00007831732923691, 9.861607340972970093, 6.659929834790830228 ) ) ;
#134036=EDGE_LOOP ( 'NONE', ( #185814, #105206, #124892, #14967 ) ) ;
#134043=CARTESIAN_POINT ( 'NONE',  ( 9.350297026732835803, 12.83744219491209293, 6.612079693597346264 ) ) ;
#134061=CARTESIAN_POINT ( 'NONE',  ( 10.62873463776380056, 9.799999999999982947, 3.199999999999997957 ) ) ;
#134068=( NAMED_UNIT ( * ) SI_UNIT ( $, .STERADIAN. ) SOLID_ANGLE_UNIT ( ) );
#134095=DIRECTION ( 'NONE',  ( 0.000000000000000000, 0.000000000000000000, -1.000000000000000000 ) ) ;
#134118=ORIENTED_EDGE ( 'NONE', *, *, #193079, .T. ) ;
#134148=CARTESIAN_POINT ( 'NONE',  ( -11.94650005372637835, 9.948972996623616893, 1.135399707157293658 ) ) ;
#134164=CARTESIAN_POINT ( 'NONE',  ( -11.55950211276791428, 12.21999999999998288, 3.221476510067114329 ) ) ;
#134187=CARTESIAN_POINT ( 'NONE',  ( 1.469576158976824144E-15, 0.08000000000000020983, 12.00000000000000178 ) ) ;
#134243=CARTESIAN_POINT ( 'NONE',  ( 8.142236001222203257, 14.23929044818452994, 8.815766320197676365 ) ) ;
#134279=EDGE_CURVE ( 'NONE', #73634, #139957, #211871, .T. ) ;
#134299=SURFACE_SIDE_STYLE ('',( #164635 ) ) ;
#134307=AXIS2_PLACEMENT_3D ( 'NONE', #150324, #101557, #134095 ) ;
#134314=ORIENTED_EDGE ( 'NONE', *, *, #127920, .F. ) ;
#134346=SURFACE_STYLE_FILL_AREA ( #3208 ) ;
#134398=CARTESIAN_POINT ( 'NONE',  ( 11.78331023100045627, 11.29999999999999893, -1.800000000000001155 ) ) ;
#134449=CARTESIAN_POINT ( 'NONE',  ( -9.348561386651960348, 5.000000000000002665, 7.001914024036568485 ) ) ;
#134450=ORIENTED_EDGE ( 'NONE', *, *, #194571, .F. ) ;
#134482=VECTOR ( 'NONE', #152466, 1000.000000000000000 ) ;
#134499=VERTEX_POINT ( 'NONE', #2396 ) ;
#134506=CARTESIAN_POINT ( 'NONE',  ( -10.29780748029859616, 4.862821740736285925, -6.167739988275216412 ) ) ;
#134517=LINE ( 'NONE', #4441, #25874 ) ;
#134538=EDGE_CURVE ( 'NONE', #148656, #167726, #172744, .T. ) ;
#134552=CARTESIAN_POINT ( 'NONE',  ( 11.48243876534946217, 11.37999999999998302, 3.199999999999997957 ) ) ;
#134572=ORIENTED_EDGE ( 'NONE', *, *, #126259, .T. ) ;
#134584=CARTESIAN_POINT ( 'NONE',  ( -10.83922355283164229, 5.627439893072521571, -6.488667358217314884 ) ) ;
#134586=LINE ( 'NONE', #117293, #112050 ) ;
#134595=CARTESIAN_POINT ( 'NONE',  ( 9.962237412473150755, 12.35880645891234408, 7.801823201411741238 ) ) ;
#134646=CARTESIAN_POINT ( 'NONE',  ( -11.73494313955695745, 7.421333685592205853, -2.519709837933482355 ) ) ;
#134668=EDGE_CURVE ( 'NONE', #33058, #36899, #191109, .T. ) ;
#134672=ADVANCED_FACE ( 'NONE', ( #143149 ), #30470, .T. ) ;
#134688=DIRECTION ( 'NONE',  ( 0.000000000000000000, 0.000000000000000000, 1.000000000000000000 ) ) ;
#134691=CARTESIAN_POINT ( 'NONE',  ( 9.228631970132592954, 13.18394157654138610, -9.019657609914000673 ) ) ;
#134744=CARTESIAN_POINT ( 'NONE',  ( 9.348761378620913831, 13.52553930298124918, -7.449808453853659529 ) ) ;
#134748=CARTESIAN_POINT ( 'NONE',  ( 11.96535697748077709, 13.75262667064441935, -0.9148528286455174241 ) ) ;
#134755=ADVANCED_FACE ( 'NONE', ( #156167 ), #125439, .F. ) ;
#134759=CARTESIAN_POINT ( 'NONE',  ( -11.84104725192634966, 11.10983537451415870, 1.443823348526939165 ) ) ;
#134782=EDGE_CURVE ( 'NONE', #173974, #77951, #109615, .T. ) ;
#134792=FILL_AREA_STYLE_COLOUR ( '', #195445 ) ;
#134804=CARTESIAN_POINT ( 'NONE',  ( -10.82839673812366321, 6.397356466741112690, 5.188991974343044156 ) ) ;
#134807=( LENGTH_UNIT ( ) NAMED_UNIT ( * ) SI_UNIT ( .MILLI., .METRE. ) );
#134809=ORIENTED_EDGE ( 'NONE', *, *, #205068, .F. ) ;
#134815=MECHANICAL_DESIGN_GEOMETRIC_PRESENTATION_REPRESENTATION('',(#68896),#207298);
#134819=DIRECTION ( 'NONE',  ( 0.000000000000000000, 0.000000000000000000, 1.000000000000000000 ) ) ;
#134824=B_SPLINE_CURVE_WITH_KNOTS ( 'NONE', 3,
 ( #140933, #158225, #108465, #43412, #124732, #206947 ),
 .UNSPECIFIED., .F., .F.,
 ( 4, 2, 4 ),
 ( 0.0006378314054480060599, 0.0009584618939205532184, 0.001279092382393100377 ),
 .UNSPECIFIED. ) ;
#134844=EDGE_LOOP ( 'NONE', ( #174673, #129645, #190536, #119231 ) ) ;
#134900=ORIENTED_EDGE ( 'NONE', *, *, #202203, .F. ) ;
#134966=CARTESIAN_POINT ( 'NONE',  ( -10.61989522411177944, 7.619981102720494448, -4.513857952992439415 ) ) ;
#134997=DIRECTION ( 'NONE',  ( 1.000000000000000000, -0.000000000000000000, -0.000000000000000000 ) ) ;
#135005=CARTESIAN_POINT ( 'NONE',  ( -11.86686399458719343, 9.990712702246623778, 1.056461745586970480 ) ) ;
#135013=MECHANICAL_DESIGN_GEOMETRIC_PRESENTATION_REPRESENTATION('',(#180002),#183379);
#135053=CIRCLE ( 'NONE', #65727, 12.00000000000000178 ) ;
#135067=CARTESIAN_POINT ( 'NONE',  ( -10.40063108925089885, 3.507138841238251370, -5.415724211249433040 ) ) ;
#135077=CARTESIAN_POINT ( 'NONE',  ( -11.52570357830391323, 8.091488070261075194, -2.173620758456770830 ) ) ;
#135083=CARTESIAN_POINT ( 'NONE',  ( 11.95102697937679359, 6.645246171022539450, 0.4972084260056497951 ) ) ;
#135087=ORIENTED_EDGE ( 'NONE', *, *, #30633, .F. ) ;
#135094=DIRECTION ( 'NONE',  ( 0.000000000000000000, 0.000000000000000000, -1.000000000000000000 ) ) ;
#135095=CARTESIAN_POINT ( 'NONE',  ( 9.280150959925951071, 13.43437406861168704, 6.783356236849154008 ) ) ;
#135106=CARTESIAN_POINT ( 'NONE',  ( 8.361471489411563596, 14.02767860296625813, -8.607966671085261368 ) ) ;
#135120=DIRECTION ( 'NONE',  ( 0.000000000000000000, 0.000000000000000000, -1.000000000000000000 ) ) ;
#135185=ADVANCED_FACE ( 'NONE', ( #133279 ), #198226, .F. ) ;
#135203=CARTESIAN_POINT ( 'NONE',  ( -11.96209379583854293, 9.772070594057634452, 0.9572398070798600056 ) ) ;
#135217=UNCERTAINTY_MEASURE_WITH_UNIT (LENGTH_MEASURE( 1.000000000000000082E-05 ), #89600, 'distance_accuracy_value', 'NONE');
#135218=VECTOR ( 'NONE', #123905, 1000.000000000000000 ) ;
#135238=PRESENTATION_STYLE_ASSIGNMENT (( #38783 ) ) ;
#135251=VERTEX_POINT ( 'NONE', #66075 ) ;
#135270=CIRCLE ( 'NONE', #166317, 0.5000000000000004441 ) ;
#135274=CARTESIAN_POINT ( 'NONE',  ( 11.43195036480941340, 13.65524496285255829, 3.649565797774438458 ) ) ;
#135307=( BOUNDED_SURFACE ( )  B_SPLINE_SURFACE ( 3, 2, ( 
 ( #157767, #89574, #14680 ),
 ( #12550, #196652, #80777 ),
 ( #146865, #195593, #160960 ),
 ( #99158, #194511, #15744 ),
 ( #177210, #163100, #180403 ),
 ( #45098, #178286, #162033 ),
 ( #210761, #181453, #46159 ),
 ( #147912, #65550, #32022 ),
 ( #94910, #213927, #78625 ),
 ( #47227, #112272, #129608 ) ),
 .UNSPECIFIED., .F., .F., .T. ) 
 B_SPLINE_SURFACE_WITH_KNOTS ( ( 4, 2, 2, 2, 4 ),
 ( 3, 3 ),
 ( 2.466559942404522587E-18, 0.0004030251014121731448, 0.0008060502028243437958, 0.001209075304236514447, 0.001612100405648685206 ),
 ( 0.000000000000000000, 1.000000000000000000 ),
 .UNSPECIFIED. ) 
 GEOMETRIC_REPRESENTATION_ITEM ( )  RATIONAL_B_SPLINE_SURFACE ( (
 ( 1.000000000000000000, 0.8509629433967630385, 1.000000000000000000),
 ( 1.000000000000000000, 0.8510310118808805946, 1.000000000000000000),
 ( 1.000000000000000000, 0.8495812529563545601, 1.000000000000000000),
 ( 1.000000000000000000, 0.8465918360525764852, 1.000000000000000000),
 ( 1.000000000000000000, 0.8452340365386274978, 1.000000000000000000),
 ( 1.000000000000000000, 0.8452309425927184705, 1.000000000000000000),
 ( 1.000000000000000000, 0.8465710739603050650, 1.000000000000000000),
 ( 1.000000000000000000, 0.8495952187152687740, 1.000000000000000000),
 ( 1.000000000000000000, 0.8510135196387145218, 1.000000000000000000),
 ( 1.000000000000000000, 0.8509629433966235945, 1.000000000000000000) ) ) 
 REPRESENTATION_ITEM ( '' )  SURFACE ( )  );
#135316=ORIENTED_EDGE ( 'NONE', *, *, #63078, .F. ) ;
#135362=CARTESIAN_POINT ( 'NONE',  ( -11.44800751630026880, 11.29999999999998117, 3.302956944461236777 ) ) ;
#135390=DIRECTION ( 'NONE',  ( -1.000000000000000000, 0.000000000000000000, 0.000000000000000000 ) ) ;
#135395=EDGE_LOOP ( 'NONE', ( #157090, #74492, #155181, #120383, #130241, #60205 ) ) ;
#135408=ADVANCED_FACE ( 'NONE', ( #14138, #153760, #5330, #137523, #69276, #138587, #166816 ), #54129, .T. ) ;
#135414=CARTESIAN_POINT ( 'NONE',  ( -11.96535697748077887, 11.25262667064452948, 0.9148528286454729042 ) ) ;
#135417=ORIENTED_EDGE ( 'NONE', *, *, #77449, .T. ) ;
#135422=CARTESIAN_POINT ( 'NONE',  ( -10.62336932346880936, 4.106376894962319390, 5.581641476743597785 ) ) ;
#135456=DIRECTION ( 'NONE',  ( -0.5773502691896166272, 0.000000000000000000, -0.8164965809277325848 ) ) ;
#135490=CARTESIAN_POINT ( 'NONE',  ( -11.75337143377970328, 4.618255228540592228, 5.022398747751031678 ) ) ;
#135491=EDGE_LOOP ( 'NONE', ( #203530, #202669, #146030, #144366 ) ) ;
#135507=ORIENTED_EDGE ( 'NONE', *, *, #108416, .F. ) ;
#135521=CARTESIAN_POINT ( 'NONE',  ( -9.367496997601206132, 15.51845925588232333, -7.499999999995496047 ) ) ;
#135541=CARTESIAN_POINT ( 'NONE',  ( -10.51720842395916300, 3.993285388006064807, -5.782618101111140163 ) ) ;
#135546=EDGE_CURVE ( 'NONE', #144017, #147946, #102057, .T. ) ;
#135559=CARTESIAN_POINT ( 'NONE',  ( -1.249999999999964695, 8.500000000000000000, -12.00100000000000122 ) ) ;
#135577=B_SPLINE_CURVE_WITH_KNOTS ( 'NONE', 3,
 ( #82464, #120, #4387, #136574, #184224, #70458 ),
 .UNSPECIFIED., .F., .F.,
 ( 4, 2, 4 ),
 ( 0.000000000000000000, 0.0003202408338303456550, 0.0006404816676606913100 ),
 .UNSPECIFIED. ) ;
#135615=ORIENTED_EDGE ( 'NONE', *, *, #98658, .T. ) ;
#135626=CARTESIAN_POINT ( 'NONE',  ( -11.13230441903222534, 5.430351611223322550, 4.009938051813186632 ) ) ;
#135638=CARTESIAN_POINT ( 'NONE',  ( 12.55138299807035551, 7.397854759914610057, -0.9335798560614338992 ) ) ;
#135649=VERTEX_POINT ( 'NONE', #154829 ) ;
#135657=CARTESIAN_POINT ( 'NONE',  ( 11.04536101718726293, 0.000000000000000000, 1.099999999999996758 ) ) ;
#135678=CYLINDRICAL_SURFACE ( 'NONE', #98151, 0.3999999999999997446 ) ;
#135680=CARTESIAN_POINT ( 'NONE',  ( 9.508009452425755015, 4.000007913748543587, -7.612499999891275237 ) ) ;
#135693=CARTESIAN_POINT ( 'NONE',  ( 11.48243876534946217, 9.799999999999982947, 3.199999999999997957 ) ) ;
#135698=CARTESIAN_POINT ( 'NONE',  ( -9.748756651352278979, 4.000007913748506283, -7.301653494139321410 ) ) ;
#135717=( LENGTH_UNIT ( ) NAMED_UNIT ( * ) SI_UNIT ( .MILLI., .METRE. ) );
#135739=CARTESIAN_POINT ( 'NONE',  ( 9.483953901554681210, 14.00935217397140953, -8.399901643884886582 ) ) ;
#135756=CARTESIAN_POINT ( 'NONE',  ( 11.97181042169641962, 13.88000000000000611, -0.8318531151397201562 ) ) ;
#135786=CARTESIAN_POINT ( 'NONE',  ( 8.336750050606532625, 15.10367673868402605, 8.570998589250198307 ) ) ;
#135787=CARTESIAN_POINT ( 'NONE',  ( -9.472340320762523191, 15.37246691557686873, 7.367375266019397628 ) ) ;
#135791=LINE ( 'NONE', #53460, #130700 ) ;
#135793=CARTESIAN_POINT ( 'NONE',  ( 10.26659657359305733, 10.85725357443524786, -6.218427518227997552 ) ) ;
#135801=CARTESIAN_POINT ( 'NONE',  ( 8.790438134619869004, 13.29428800202395955, -8.101059483297389008 ) ) ;
#135804=ORIENTED_EDGE ( 'NONE', *, *, #39389, .T. ) ;
#135807=CARTESIAN_POINT ( 'NONE',  ( 11.84668730067608777, 10.09365272245202938, 1.399999999999998579 ) ) ;
#135824=SHAPE_REPRESENTATION ( 'chamber', ( #200407 ), #110829 ) ;
#135833=CARTESIAN_POINT ( 'NONE',  ( 11.48243876534946217, 11.29999999999999893, -3.200000000000001510 ) ) ;
#135849=MECHANICAL_DESIGN_GEOMETRIC_PRESENTATION_REPRESENTATION('',(#208338),#142682);
#135852=CARTESIAN_POINT ( 'NONE',  ( -11.13121356413584095, 7.259994163161730185, 4.367082668627133124 ) ) ;
#135855=FILL_AREA_STYLE_COLOUR ( '', #81701 ) ;
#135873=ORIENTED_EDGE ( 'NONE', *, *, #57116, .F. ) ;
#135900=DIRECTION ( 'NONE',  ( -0.000000000000000000, -1.000000000000000000, -0.000000000000000000 ) ) ;
#135941=EDGE_CURVE ( 'NONE', #152913, #16328, #164353, .T. ) ;
#135944=AXIS2_PLACEMENT_3D ( 'NONE', #54045, #106044, #89771 ) ;
#135958=FILL_AREA_STYLE_COLOUR ( '', #184331 ) ;
#135967=EDGE_CURVE ( 'NONE', #172406, #187025, #60448, .T. ) ;
#135982=SURFACE_STYLE_USAGE ( .BOTH. , #151170 ) ;
#135990=UNCERTAINTY_MEASURE_WITH_UNIT (LENGTH_MEASURE( 1.000000000000000082E-05 ), #89847, 'distance_accuracy_value', 'NONE');
#135991=CARTESIAN_POINT ( 'NONE',  ( -10.59765138761703085, 11.29999999999998295, 3.303242380465396977 ) ) ;
#136016=CARTESIAN_POINT ( 'NONE',  ( -8.065673753978270355, 13.99999996918362832, -8.613976771946813216 ) ) ;
#136018=CARTESIAN_POINT ( 'NONE',  ( -10.78227258717170578, 6.269840026405313793, 4.500979083849748541 ) ) ;
#136027=CARTESIAN_POINT ( 'NONE',  ( -11.04978080397792972, 9.991554750122867645, 1.057339094031728211 ) ) ;
#136039=VECTOR ( 'NONE', #174952, 1000.000000000000000 ) ;
#136060=SURFACE_STYLE_FILL_AREA ( #139264 ) ;
#136086=VERTEX_POINT ( 'NONE', #60508 ) ;
#136111=AXIS2_PLACEMENT_3D ( 'NONE', #24402, #102481, #204209 ) ;
#136112=ORIENTED_EDGE ( 'NONE', *, *, #113251, .F. ) ;
#136120=ORIENTED_EDGE ( 'NONE', *, *, #166530, .T. ) ;
#136122=EDGE_CURVE ( 'NONE', #21255, #67257, #183085, .T. ) ;
#136126=CARTESIAN_POINT ( 'NONE',  ( -10.24056286296518614, 5.004077596833054642, -7.476959758773280562 ) ) ;
#136127=FILL_AREA_STYLE_COLOUR ( '', #118029 ) ;
#136132=CARTESIAN_POINT ( 'NONE',  ( 0.000000000000000000, 12.21999999999998288, 0.000000000000000000 ) ) ;
#136142=CARTESIAN_POINT ( 'NONE',  ( 11.79264299610848177, 6.877264176558675501, -1.951597671399909917 ) ) ;
#136155=CARTESIAN_POINT ( 'NONE',  ( 8.642161254816231875, 12.08761591892186082, -8.327710695117993112 ) ) ;
#136166=CARTESIAN_POINT ( 'NONE',  ( -3.518235019283448395, 15.44797960873222742, -11.43489012466130283 ) ) ;
#136170=CARTESIAN_POINT ( 'NONE',  ( 10.56513397747884397, 9.840999034856560357, 3.405015282931167508 ) ) ;
#136180=DIRECTION ( 'NONE',  ( 0.000000000000000000, -1.000000000000000000, -0.000000000000000000 ) ) ;
#136198=PLANE ( 'NONE',  #116022 ) ;
#136229=ORIENTED_EDGE ( 'NONE', *, *, #194044, .T. ) ;
#136253=EDGE_CURVE ( 'NONE', #170509, #163825, #90908, .T. ) ;
#136295=DIRECTION ( 'NONE',  ( 1.000000000000000000, 0.000000000000000000, -0.000000000000000000 ) ) ;
#136303=CARTESIAN_POINT ( 'NONE',  ( -15.75000000000000000, 12.69999999999999929, -0.7000000000000009548 ) ) ;
#136307=CARTESIAN_POINT ( 'NONE',  ( -15.75000000000000000, 10.89999999999998259, 3.599999999999999201 ) ) ;
#136311=B_SPLINE_CURVE_WITH_KNOTS ( 'NONE', 3,
 ( #108263, #146048, #162279, #160141, #47480, #126655, #147106, #180648, #77815, #192622, #64761, #210999, #177462, #62623, #195839, #13866 ),
 .UNSPECIFIED., .F., .F.,
 ( 4, 2, 2, 2, 2, 2, 2, 4 ),
 ( 0.6095821870314059865, 0.6120980958896804491, 0.6146140047479549118, 0.6196458224645037260, 0.6297094578976014656, 0.6397880689092279027, 0.6448273744150412323, 0.6498666799208544509 ),
 .UNSPECIFIED. ) ;
#136313=SURFACE_STYLE_FILL_AREA ( #170925 ) ;
#136314=CIRCLE ( 'NONE', #205388, 0.07999999999999998779 ) ;
#136330=( GEOMETRIC_REPRESENTATION_CONTEXT ( 3 ) GLOBAL_UNCERTAINTY_ASSIGNED_CONTEXT ( ( #9990 ) ) GLOBAL_UNIT_ASSIGNED_CONTEXT ( ( #73905, #191895, #59780 ) ) REPRESENTATION_CONTEXT ( 'NONE', 'WORKASPACE' ) );
#136334=CARTESIAN_POINT ( 'NONE',  ( 11.35573736746270335, 13.61270414413280250, 3.554362808847919553 ) ) ;
#136340=CARTESIAN_POINT ( 'NONE',  ( -11.33772463945036968, 13.40000000000000036, -3.680000000000001048 ) ) ;
#136354=DIRECTION ( 'NONE',  ( -1.000000000000000000, 0.000000000000000000, 1.224646799147352961E-16 ) ) ;
#136382=ORIENTED_EDGE ( 'NONE', *, *, #52780, .T. ) ;
#136416=CARTESIAN_POINT ( 'NONE',  ( -11.89942855770814134, 13.79999999999999893, 0.6999999999999992895 ) ) ;
#136417=CARTESIAN_POINT ( 'NONE',  ( -9.956232484441596142, 5.504245459870187318, 6.026037945409589369 ) ) ;
#136433=DIRECTION ( 'NONE',  ( 0.000000000000000000, -1.000000000000000000, 0.000000000000000000 ) ) ;
#136455=CARTESIAN_POINT ( 'NONE',  ( 1.500000000000053291, 7.750000000000000000, 15.74999999999999289 ) ) ;
#136459=CARTESIAN_POINT ( 'NONE',  ( 1.734723475976807094E-15, 15.42733875946000133, 11.91973154060105955 ) ) ;
#136465=DIRECTION ( 'NONE',  ( 0.000000000000000000, 0.000000000000000000, 1.000000000000000000 ) ) ;
#136466=DIRECTION ( 'NONE',  ( -0.7806247497998004548, 0.000000000000000000, -0.6249999999999992228 ) ) ;
#136481=CARTESIAN_POINT ( 'NONE',  ( -11.48243876534946217, 12.22000000000000064, -3.200000000000001510 ) ) ;
#136491=DIRECTION ( 'NONE',  ( 0.000000000000000000, -1.000000000000000000, -0.000000000000000000 ) ) ;
#136492=CARTESIAN_POINT ( 'NONE',  ( -10.52558186178533539, 3.957600067444659420, 5.763924342718092397 ) ) ;
#136503=ADVANCED_FACE ( 'NONE', ( #49594 ), #212072, .F. ) ;
#136534=EDGE_CURVE ( 'NONE', #195844, #205382, #172584, .T. ) ;
#136559=CARTESIAN_POINT ( 'NONE',  ( -10.22583553578405358, 2.999999999999999556, 7.498742284419905424 ) ) ;
#136560=ORIENTED_EDGE ( 'NONE', *, *, #204060, .F. ) ;
#136574=CARTESIAN_POINT ( 'NONE',  ( 10.56502152068524758, 11.25866949347406631, -3.405356014006697407 ) ) ;
#136589=CARTESIAN_POINT ( 'NONE',  ( -9.367496996949647325, 15.51845925588232333, 7.500000000809289524 ) ) ;
#136600=CARTESIAN_POINT ( 'NONE',  ( 11.96209379583854293, 13.82792940594236519, 0.9572398070798464609 ) ) ;
#136615=CARTESIAN_POINT ( 'NONE',  ( 11.92619526913699701, 12.69999999999998153, 1.328859060402682868 ) ) ;
#136639=CIRCLE ( 'NONE', #74320, 0.07999999999999998779 ) ;
#136641=CARTESIAN_POINT ( 'NONE',  ( -1.120076944892877790, 15.44751560850434302, -11.90518184135781077 ) ) ;
#136644=VERTEX_POINT ( 'NONE', #67939 ) ;
#136646=AXIS2_PLACEMENT_3D ( 'NONE', #79146, #145262, #212328 ) ;
#136652=B_SPLINE_CURVE_WITH_KNOTS ( 'NONE', 3,
 ( #96607, #13186, #93406, #11041, #146426, #47861 ),
 .UNSPECIFIED., .F., .F.,
 ( 4, 2, 4 ),
 ( 0.000000000000000000, 0.0003767643964918265939, 0.0007535287929836531878 ),
 .UNSPECIFIED. ) ;
#136654=ORIENTED_EDGE ( 'NONE', *, *, #77746, .F. ) ;
#136659=FACE_BOUND ( 'NONE', #95482, .T. ) ;
#136675=PLANE ( 'NONE',  #106089 ) ;
#136677=FACE_OUTER_BOUND ( 'NONE', #151761, .T. ) ;
#136694=CARTESIAN_POINT ( 'NONE',  ( -11.37872555039425748, 6.127336012342636806, -3.407788289652350588 ) ) ;
#136699=CARTESIAN_POINT ( 'NONE',  ( 7.032126278729658786, 15.00000000000000000, -9.944928355699694578 ) ) ;
#136710=EDGE_LOOP ( 'NONE', ( #40947, #49445, #162157, #18128 ) ) ;
#136718=CARTESIAN_POINT ( 'NONE',  ( -10.98535488200955079, 9.841774432527699901, -1.593017372382190766 ) ) ;
#136735=AXIS2_PLACEMENT_3D ( 'NONE', #34758, #30529, #100832 ) ;
#136775=LINE ( 'NONE', #185497, #167250 ) ;
#136804=CARTESIAN_POINT ( 'NONE',  ( 7.826754997383993384, 14.96923099944252478, -9.976823565866945742 ) ) ;
#136812=DIRECTION ( 'NONE',  ( -1.000000000000000000, 0.000000000000000000, 1.224646799147352961E-16 ) ) ;
#136820=CARTESIAN_POINT ( 'NONE',  ( 11.89844258446855818, 13.82852689329961215, -1.560502987793222163 ) ) ;
#136856=CARTESIAN_POINT ( 'NONE',  ( -9.367496997602181352, 15.51845925588869690, 7.499999999994336974 ) ) ;
#136860=SURFACE_SIDE_STYLE ('',( #150979 ) ) ;
#136888=ADVANCED_FACE ( 'NONE', ( #153506 ), #136198, .F. ) ;
#136903=CARTESIAN_POINT ( 'NONE',  ( -9.508009452553693563, 15.00000000001204370, -7.612499999986095389 ) ) ;
#136910=CARTESIAN_POINT ( 'NONE',  ( -11.33772463945037146, 10.89999999999998259, 3.599999999999999201 ) ) ;
#136921=CARTESIAN_POINT ( 'NONE',  ( -15.75000000000000000, 10.19999999999999929, -3.600000000000000977 ) ) ;
#136936=AXIS2_PLACEMENT_3D ( 'NONE', #47875, #27317, #177857 ) ;
#136940=FILL_AREA_STYLE ('',( #152115 ) ) ;
#136945=ORIENTED_EDGE ( 'NONE', *, *, #102377, .T. ) ;
#136968=CARTESIAN_POINT ( 'NONE',  ( -9.604686356149274573, 4.518459255872632419, 7.193747284969079558 ) ) ;
#136969=CARTESIAN_POINT ( 'NONE',  ( -0.01238645465998293969, 15.45067886748792851, 11.96329637218392072 ) ) ;
#136977=FACE_OUTER_BOUND ( 'NONE', #133062, .T. ) ;
#137045=CARTESIAN_POINT ( 'NONE',  ( 9.086253353280454803, 13.39999999999999680, -7.838367176906162470 ) ) ;
#137084=CARTESIAN_POINT ( 'NONE',  ( 1.050790385994986309, 14.00000000000000711, -12.64745918785790657 ) ) ;
#137086=CARTESIAN_POINT ( 'NONE',  ( -10.83925572545688176, 5.627432043407306850, 6.488667418600651438 ) ) ;
#137097=CARTESIAN_POINT ( 'NONE',  ( -11.04536101718726293, 10.09542727035991483, 1.099999999999998757 ) ) ;
#137118=CARTESIAN_POINT ( 'NONE',  ( 10.35123481171224569, 10.47441674329072114, 5.983190950231344729 ) ) ;
#137126=( LENGTH_UNIT ( ) NAMED_UNIT ( * ) SI_UNIT ( .MILLI., .METRE. ) );
#137138=( GEOMETRIC_REPRESENTATION_CONTEXT ( 3 ) GLOBAL_UNCERTAINTY_ASSIGNED_CONTEXT ( ( #74750 ) ) GLOBAL_UNIT_ASSIGNED_CONTEXT ( ( #117905, #167655, #24591 ) ) REPRESENTATION_CONTEXT ( 'NONE', 'WORKASPACE' ) );
#137156=VECTOR ( 'NONE', #32069, 1000.000000000000000 ) ;
#137185=EDGE_LOOP ( 'NONE', ( #211526, #10381, #85782, #11874 ) ) ;
#137191=ORIENTED_EDGE ( 'NONE', *, *, #103751, .T. ) ;
#137198=CARTESIAN_POINT ( 'NONE',  ( -11.23979429089589033, 4.930458577253933328, -5.866063493660276684 ) ) ;
#137200=EDGE_CURVE ( 'NONE', #157346, #74053, #139399, .T. ) ;
#137210=CARTESIAN_POINT ( 'NONE',  ( -10.45142682343936791, 5.144546645612242841, 5.216777551074719632 ) ) ;
#137217=CARTESIAN_POINT ( 'NONE',  ( 11.82993880136642417, 6.822466781481484333, -1.712400514339024626 ) ) ;
#137239=CARTESIAN_POINT ( 'NONE',  ( -8.804420911738874977, 15.51845923041438979, -8.203281805575960206 ) ) ;
#137280=CARTESIAN_POINT ( 'NONE',  ( 0.000000000000000000, 7.000000000000000000, 0.000000000000000000 ) ) ;
#137285=FACE_OUTER_BOUND ( 'NONE', #32235, .T. ) ;
#137366=( NAMED_UNIT ( * ) SI_UNIT ( $, .STERADIAN. ) SOLID_ANGLE_UNIT ( ) );
#137396=CYLINDRICAL_SURFACE ( 'NONE', #197993, 0.08000000000000020983 ) ;
#137397=FILL_AREA_STYLE ('',( #186116 ) ) ;
#137412=EDGE_CURVE ( 'NONE', #203495, #130695, #39908, .T. ) ;
#137433=EDGE_CURVE ( 'NONE', #19959, #195013, #91879, .T. ) ;
#137447=( GEOMETRIC_REPRESENTATION_CONTEXT ( 3 ) GLOBAL_UNCERTAINTY_ASSIGNED_CONTEXT ( ( #124653 ) ) GLOBAL_UNIT_ASSIGNED_CONTEXT ( ( #205548, #89706, #5195 ) ) REPRESENTATION_CONTEXT ( 'NONE', 'WORKASPACE' ) );
#137469=CARTESIAN_POINT ( 'NONE',  ( -11.86239285000045918, 9.799999999999981171, 1.812080536912751283 ) ) ;
#137485=CARTESIAN_POINT ( 'NONE',  ( -9.669761313225400556, 3.035266360176858136, 6.558537842936834394 ) ) ;
#137506=DIRECTION ( 'NONE',  ( 0.6250000000000005551, -0.000000000000000000, 0.7806247497997993445 ) ) ;
#137511=CARTESIAN_POINT ( 'NONE',  ( -0.4504913314191360540, 15.51845925279681815, -11.99999999998148326 ) ) ;
#137523=FACE_BOUND ( 'NONE', #55312, .T. ) ;
#137524=EDGE_CURVE ( 'NONE', #210323, #37563, #64186, .T. ) ;
#137530=SURFACE_STYLE_USAGE ( .BOTH. , #69283 ) ;
#137535=SURFACE_STYLE_FILL_AREA ( #87699 ) ;
#137539=DIRECTION ( 'NONE',  ( 0.000000000000000000, 0.000000000000000000, -1.000000000000000000 ) ) ;
#137551=CARTESIAN_POINT ( 'NONE',  ( -11.94980361490429921, 11.00332124735865769, 1.099999952233555733 ) ) ;
#137580=CARTESIAN_POINT ( 'NONE',  ( -7.105968778775219263, 15.51980109384565409, 9.680178325039504372 ) ) ;
#137597=EDGE_CURVE ( 'NONE', #20233, #139854, #176167, .T. ) ;
#137629=CARTESIAN_POINT ( 'NONE',  ( -10.67000816626867810, 5.238978589329153834, 6.814456324518622488 ) ) ;
#137633=CARTESIAN_POINT ( 'NONE',  ( 0.000000000000000000, 13.79999999999999893, 0.000000000000000000 ) ) ;
#137637=ORIENTED_EDGE ( 'NONE', *, *, #75347, .T. ) ;
#137642=ORIENTED_EDGE ( 'NONE', *, *, #196604, .T. ) ;
#137643=PRESENTATION_STYLE_ASSIGNMENT (( #55313 ) ) ;
#137657=CARTESIAN_POINT ( 'NONE',  ( -9.508802380709459712, 14.89824926832925911, -7.212919681761617241 ) ) ;
#137678=CARTESIAN_POINT ( 'NONE',  ( -3.435200284438673535, 14.55196833484455254, 11.46022242559163473 ) ) ;
#137695=LINE ( 'NONE', #135559, #36395 ) ;
#137727=FACE_BOUND ( 'NONE', #38658, .T. ) ;
#137734=PRESENTATION_STYLE_ASSIGNMENT (( #71621 ) ) ;
#137763=CARTESIAN_POINT ( 'NONE',  ( -11.55950211276791428, 12.22000000000000064, -3.221476510067114329 ) ) ;
#137764=CARTESIAN_POINT ( 'NONE',  ( -11.01567899581106325, 5.044704703271206903, 4.264317011375222677 ) ) ;
#137788=VERTEX_POINT ( 'NONE', #159907 ) ;
#137789=AXIS2_PLACEMENT_3D ( 'NONE', #43125, #140635, #62537 ) ;
#137802=AXIS2_PLACEMENT_3D ( 'NONE', #212505, #130288, #170157 ) ;
#137810=ORIENTED_EDGE ( 'NONE', *, *, #173301, .T. ) ;
#137822=ORIENTED_EDGE ( 'NONE', *, *, #163282, .T. ) ;
#137832=CARTESIAN_POINT ( 'NONE',  ( 11.33772463945037146, 10.19999999999998153, 3.599999999999999201 ) ) ;
#137849=ORIENTED_EDGE ( 'NONE', *, *, #182170, .F. ) ;
#137936=( GEOMETRIC_REPRESENTATION_CONTEXT ( 3 ) GLOBAL_UNCERTAINTY_ASSIGNED_CONTEXT ( ( #14754 ) ) GLOBAL_UNIT_ASSIGNED_CONTEXT ( ( #46865, #63088, #112978 ) ) REPRESENTATION_CONTEXT ( 'NONE', 'WORKASPACE' ) );
#138006=CARTESIAN_POINT ( 'NONE',  ( -11.52901446936762575, 13.79425527467597234, 3.330874149801142270 ) ) ;
#138008=ADVANCED_FACE ( 'NONE', ( #211836 ), #15748, .T. ) ;
#138020=ORIENTED_EDGE ( 'NONE', *, *, #48333, .F. ) ;
#138034=CARTESIAN_POINT ( 'NONE',  ( 9.367496997597593023, 3.481540744127370690, -7.500000000000005329 ) ) ;
#138044=CARTESIAN_POINT ( 'NONE',  ( -10.89798411099869035, 6.655715830334343330, 5.027853787196250757 ) ) ;
#138050=CIRCLE ( 'NONE', #186426, 0.08000000000000014044 ) ;
#138078=DIRECTION ( 'NONE',  ( 0.000000000000000000, 1.000000000000000000, 0.000000000000000000 ) ) ;
#138089=( GEOMETRIC_REPRESENTATION_CONTEXT ( 3 ) GLOBAL_UNCERTAINTY_ASSIGNED_CONTEXT ( ( #97117 ) ) GLOBAL_UNIT_ASSIGNED_CONTEXT ( ( #74601, #38899, #140705 ) ) REPRESENTATION_CONTEXT ( 'NONE', 'WORKASPACE' ) );
#138097=( NAMED_UNIT ( * ) SI_UNIT ( $, .STERADIAN. ) SOLID_ANGLE_UNIT ( ) );
#138108=CARTESIAN_POINT ( 'NONE',  ( -9.367496997601300279, 15.00000000000599165, -7.679999999987998649 ) ) ;
#138124=CARTESIAN_POINT ( 'NONE',  ( -11.92045683181315674, 13.65275927879484819, -1.382340670101859237 ) ) ;
#138158=CARTESIAN_POINT ( 'NONE',  ( -12.04410816989902955, 7.377574010548016759, -3.959763750030863783 ) ) ;
#138215=DIRECTION ( 'NONE',  ( -0.000000000000000000, -1.000000000000000000, -0.000000000000000000 ) ) ;
#138227=EDGE_LOOP ( 'NONE', ( #151684, #127052, #116755, #23372, #112771 ) ) ;
#138236=CARTESIAN_POINT ( 'NONE',  ( 0.000000000000000000, 0.000000000000000000, 11.09999999999999964 ) ) ;
#138259=ORIENTED_EDGE ( 'NONE', *, *, #176346, .F. ) ;
#138264=CARTESIAN_POINT ( 'NONE',  ( -9.670366421564544623, 3.035553407718987629, -6.557686755922881972 ) ) ;
#138273=CARTESIAN_POINT ( 'NONE',  ( -10.78237064342727791, 6.270194388237658956, -4.501389708959286473 ) ) ;
#138279=DIRECTION ( 'NONE',  ( -7.993605777301127091E-15, 0.000000000000000000, -1.000000000000000000 ) ) ;
#138289=ORIENTED_EDGE ( 'NONE', *, *, #131699, .F. ) ;
#138322=VERTEX_POINT ( 'NONE', #150055 ) ;
#138340=MECHANICAL_DESIGN_GEOMETRIC_PRESENTATION_REPRESENTATION('',(#155498),#172827);
#138342=CARTESIAN_POINT ( 'NONE',  ( 1.734723475976807094E-15, 15.42691958146951414, 11.91973154060106665 ) ) ;
#138347=CARTESIAN_POINT ( 'NONE',  ( -9.348526197514022584, 4.999985930147239799, -7.001887667968696327 ) ) ;
#138353=EDGE_CURVE ( 'NONE', #77951, #66179, #167912, .T. ) ;
#138453=AXIS2_PLACEMENT_3D ( 'NONE', #79505, #209480, #194321 ) ;
#138474=FILL_AREA_STYLE_COLOUR ( '', #85819 ) ;
#138483=CARTESIAN_POINT ( 'NONE',  ( 9.452953987210896969, 3.481541100950246381, -7.393264229718174541 ) ) ;
#138495=CARTESIAN_POINT ( 'NONE',  ( -1.474414414893459258, 7.826756755319736136, -10.64843978026285320 ) ) ;
#138529=CARTESIAN_POINT ( 'NONE',  ( -11.92619526913700057, 10.19999999999998153, 1.328859060402682868 ) ) ;
#138544=CARTESIAN_POINT ( 'NONE',  ( -11.89204169242383102, 13.79999999999999893, 0.8046421800351404308 ) ) ;
#138545=AXIS2_PLACEMENT_3D ( 'NONE', #195033, #162549, #28269 ) ;
#138546=CARTESIAN_POINT ( 'NONE',  ( -9.645001968711920171, 4.042125922905831281, 6.587946042608958663 ) ) ;
#138556=ADVANCED_FACE ( 'NONE', ( #185720 ), #124038, .T. ) ;
#138587=FACE_BOUND ( 'NONE', #59827, .T. ) ;
#138600=( NAMED_UNIT ( * ) PLANE_ANGLE_UNIT ( ) SI_UNIT ( $, .RADIAN. ) );
#138613=CARTESIAN_POINT ( 'NONE',  ( -11.96212011828584210, 11.32812445049947669, 0.9569185076417884295 ) ) ;
#138623=VERTEX_POINT ( 'NONE', #173794 ) ;
#138644=CARTESIAN_POINT ( 'NONE',  ( -5.577069096748362043, 15.51842150349689042, 10.63472584745987426 ) ) ;
#138654=ORIENTED_EDGE ( 'NONE', *, *, #68346, .F. ) ;
#138656=CARTESIAN_POINT ( 'NONE',  ( 0.000000000000000000, 11.29999999999999893, 0.000000000000000000 ) ) ;
#138659=CARTESIAN_POINT ( 'NONE',  ( 11.86239285000045740, 11.37999999999999901, -1.812080536912752837 ) ) ;
#138664=CARTESIAN_POINT ( 'NONE',  ( 11.89835103415199313, 12.27106914167532103, 1.561208891256346876 ) ) ;
#138672=EDGE_LOOP ( 'NONE', ( #125311, #25745, #49560, #190794 ) ) ;
#138684=SURFACE_STYLE_USAGE ( .BOTH. , #41189 ) ;
#138690=CARTESIAN_POINT ( 'NONE',  ( 11.86145016429272836, 13.40000000000000036, 1.179999999999997051 ) ) ;
#138694=CARTESIAN_POINT ( 'NONE',  ( -11.25552992593869206, 3.531787801817266370, 5.933966561491729408 ) ) ;
#138710=CARTESIAN_POINT ( 'NONE',  ( -15.75000000000000000, 13.79999999999998295, 3.199999999999997957 ) ) ;
#138744=CARTESIAN_POINT ( 'NONE',  ( -9.367496997647986490, 14.53091781611831834, 7.499999999937057460 ) ) ;
#138807=ADVANCED_FACE ( 'NONE', ( #172706 ), #94370, .T. ) ;
#138814=VERTEX_POINT ( 'NONE', #46988 ) ;
#138826=EDGE_CURVE ( 'NONE', #181742, #121570, #55924, .T. ) ;
#138828=( LENGTH_UNIT ( ) NAMED_UNIT ( * ) SI_UNIT ( .MILLI., .METRE. ) );
#138829=CARTESIAN_POINT ( 'NONE',  ( -11.52570357830391323, 8.091488070261075194, -2.173620758456770830 ) ) ;
#138832=CARTESIAN_POINT ( 'NONE',  ( 8.302289836269501677, 14.87052365979419655, 9.588395110663297416 ) ) ;
#138860=DIRECTION ( 'NONE',  ( 5.578174157656880098E-15, 1.000000000000000000, 7.437565543542506798E-15 ) ) ;
#138881=ORIENTED_EDGE ( 'NONE', *, *, #187841, .T. ) ;
#138897=( NAMED_UNIT ( * ) PLANE_ANGLE_UNIT ( ) SI_UNIT ( $, .RADIAN. ) );
#138921=SURFACE_STYLE_FILL_AREA ( #206019 ) ;
#138943=CARTESIAN_POINT ( 'NONE',  ( 9.348381460497192208, 13.52536904890506619, 7.450314784081279562 ) ) ;
#138983=EDGE_CURVE ( 'NONE', #197365, #702, #140429, .T. ) ;
#139003=CARTESIAN_POINT ( 'NONE',  ( 11.81900460097218186, 13.75757134874136334, 1.592493057836596115 ) ) ;
#139004=CARTESIAN_POINT ( 'NONE',  ( -10.48267169704037727, 5.268073273308885973, 5.153989745587932880 ) ) ;
#139009=CARTESIAN_POINT ( 'NONE',  ( -5.995491887707443013, 14.48115541362584402, -10.40458799691657532 ) ) ;
#139043=DIRECTION ( 'NONE',  ( 0.000000000000000000, 0.2128498979015776560, 0.9770849098022587054 ) ) ;
#139088=EDGE_CURVE ( 'NONE', #83814, #49203, #8966, .T. ) ;
#139091=EDGE_LOOP ( 'NONE', ( #92207, #173493 ) ) ;
#139094=ORIENTED_EDGE ( 'NONE', *, *, #57012, .F. ) ;
#139099=ORIENTED_EDGE ( 'NONE', *, *, #158166, .T. ) ;
#139110=PRESENTATION_STYLE_ASSIGNMENT (( #172678 ) ) ;
#139136=CARTESIAN_POINT ( 'NONE',  ( -10.95308175811721085, 12.29999999999998295, 1.799999999999999600 ) ) ;
#139146=FACE_OUTER_BOUND ( 'NONE', #129481, .T. ) ;
#139156=ORIENTED_EDGE ( 'NONE', *, *, #139088, .F. ) ;
#139169=FACE_OUTER_BOUND ( 'NONE', #123494, .T. ) ;
#139180=CARTESIAN_POINT ( 'NONE',  ( 9.086253353280449474, 13.40000000000000036, 7.838367176906169576 ) ) ;
#139187=CARTESIAN_POINT ( 'NONE',  ( 9.410656278130334229, 14.12788591601509758, 8.484697815724119963 ) ) ;
#139220=CARTESIAN_POINT ( 'NONE',  ( -11.31087111570240467, 5.182330806778288057, -5.726608797552268371 ) ) ;
#139228=CARTESIAN_POINT ( 'NONE',  ( 11.01135777277262306, 11.00632581993708570, 1.399999999999998579 ) ) ;
#139241=( BOUNDED_SURFACE ( )  B_SPLINE_SURFACE ( 3, 2, ( 
 ( #158383, #27291, #174650 ),
 ( #156256, #175701, #11033 ),
 ( #91263, #24088, #26226 ),
 ( #92342, #141102, #93399 ),
 ( #189798, #142155, #73926 ),
 ( #59801, #43578, #106475 ),
 ( #127030, #172502, #39287 ),
 ( #143235, #89126, #105382 ),
 ( #171421, #109698, #155180 ),
 ( #90193, #6764, #190855 ),
 ( #42516, #125958, #72839 ),
 ( #138943, #204964, #7835 ) ),
 .UNSPECIFIED., .F., .F., .T. ) 
 B_SPLINE_SURFACE_WITH_KNOTS ( ( 4, 2, 2, 2, 2, 4 ),
 ( 3, 3 ),
 ( 6.288372600415925717E-18, 0.001066554601603806208, 0.001599831902405706276, 0.002133109203207606344, 0.003199663804811406480, 0.004266218406415206617 ),
 ( 0.000000000000000000, 1.000000000000000000 ),
 .UNSPECIFIED. ) 
 GEOMETRIC_REPRESENTATION_ITEM ( )  RATIONAL_B_SPLINE_SURFACE ( (
 ( 1.000000000000000000, 0.8509626965198142656, 1.000000000000000000),
 ( 1.000000000000000000, 0.8509149327537995910, 1.000000000000000000),
 ( 1.000000000000000000, 0.8506374068021691492, 1.000000000000000000),
 ( 1.000000000000000000, 0.8504793255920759520, 1.000000000000000000),
 ( 1.000000000000000000, 0.8504520640024009204, 1.000000000000000000),
 ( 1.000000000000000000, 0.8502690826081933384, 1.000000000000000000),
 ( 1.000000000000000000, 0.8502072942086275065, 1.000000000000000000),
 ( 1.000000000000000000, 0.8489325510347147663, 1.000000000000000000),
 ( 1.000000000000000000, 0.8474238666478376425, 1.000000000000000000),
 ( 1.000000000000000000, 0.8452420265713719294, 1.000000000000000000),
 ( 1.000000000000000000, 0.8443493681871490075, 1.000000000000000000),
 ( 1.000000000000000000, 0.8435444081809017058, 1.000000000000000000) ) ) 
 REPRESENTATION_ITEM ( '' )  SURFACE ( )  );
#139252=CARTESIAN_POINT ( 'NONE',  ( 9.527611255715328298, 12.67370358187078239, 7.222190795531108876 ) ) ;
#139264=FILL_AREA_STYLE ('',( #186920 ) ) ;
#139280=COLOUR_RGB ( '', 0.08235294, 0.09019608, 0.10196078) ;
#139281=AXIS2_PLACEMENT_3D ( 'NONE', #82505, #116142, #35890 ) ;
#139284=CARTESIAN_POINT ( 'NONE',  ( 11.04536101718726293, 10.09537905954598180, 1.099999999999999201 ) ) ;
#139288=LINE ( 'NONE', #170695, #18101 ) ;
#139313=VECTOR ( 'NONE', #11204, 1000.000000000000000 ) ;
#139319=FILL_AREA_STYLE ('',( #207491 ) ) ;
#139344=CARTESIAN_POINT ( 'NONE',  ( -10.12885446735897510, 6.153639267710001803, -5.673676530672286944 ) ) ;
#139350=CARTESIAN_POINT ( 'NONE',  ( 8.868224039976556838, 12.79319246706557678, 8.085344725444658209 ) ) ;
#139372=EDGE_LOOP ( 'NONE', ( #169601, #6145, #45082, #29397 ) ) ;
#139393=VERTEX_POINT ( 'NONE', #65318 ) ;
#139399=LINE ( 'NONE', #205432, #8815 ) ;
#139413=FACE_OUTER_BOUND ( 'NONE', #35945, .T. ) ;
#139418=CARTESIAN_POINT ( 'NONE',  ( -10.30104275384242740, 4.689840931292195592, -5.506867539468097483 ) ) ;
#139503=FILL_AREA_STYLE ('',( #71252 ) ) ;
#139522=CARTESIAN_POINT ( 'NONE',  ( 11.86145017354087372, 11.00485634456124018, 1.099999999999996980 ) ) ;
#139530=EDGE_LOOP ( 'NONE', ( #91252, #200304, #98571, #15050, #17445 ) ) ;
#139531=AXIS2_PLACEMENT_3D ( 'NONE', #139895, #3443, #69510 ) ;
#139589=VECTOR ( 'NONE', #98783, 1000.000000000000000 ) ;
#139595=FACE_OUTER_BOUND ( 'NONE', #92365, .T. ) ;
#139609=CARTESIAN_POINT ( 'NONE',  ( -11.78331023100045627, 9.799999999999982947, 1.799999999999999600 ) ) ;
#139621=ORIENTED_EDGE ( 'NONE', *, *, #85474, .T. ) ;
#139624=FACE_OUTER_BOUND ( 'NONE', #22374, .T. ) ;
#139625=CARTESIAN_POINT ( 'NONE',  ( -11.05071387823260487, 4.509444648491869323, 6.218574854545789066 ) ) ;
#139631=CARTESIAN_POINT ( 'NONE',  ( -11.92050416151432835, 11.15205375279624178, -1.381922468431411088 ) ) ;
#139638=LINE ( 'NONE', #175326, #97473 ) ;
#139650=DIRECTION ( 'NONE',  ( 0.000000000000000000, 1.000000000000000000, 0.000000000000000000 ) ) ;
#139656=CARTESIAN_POINT ( 'NONE',  ( -1.792254920982459199, 15.51967661332317050, -11.87386578584006358 ) ) ;
#139657=CARTESIAN_POINT ( 'NONE',  ( -3.110356790690614215, 14.48006632018288542, 11.59859428470667453 ) ) ;
#139664=SURFACE_SIDE_STYLE ('',( #202473 ) ) ;
#139668=CARTESIAN_POINT ( 'NONE',  ( -15.75000000000000000, 13.40000000000000036, 0.6999999999999992895 ) ) ;
#139674=CARTESIAN_POINT ( 'NONE',  ( -11.07790593930098311, 12.30000000000000071, 0.6999999999999992895 ) ) ;
#139691=CARTESIAN_POINT ( 'NONE',  ( -11.92619526913699879, 13.39999999999998259, 1.328859060402684644 ) ) ;
#139723=CARTESIAN_POINT ( 'NONE',  ( -5.951577129995881954, 15.44725960769734208, 10.37887709679271175 ) ) ;
#139726=( BOUNDED_SURFACE ( )  B_SPLINE_SURFACE ( 3, 2, ( 
 ( #155288, #57784, #26339 ),
 ( #172615, #109810, #11148 ),
 ( #189913, #91377, #41558 ),
 ( #89237, #175819, #205078 ),
 ( #25275, #42628, #59912 ),
 ( #23120, #24191, #6870 ) ),
 .UNSPECIFIED., .F., .F., .T. ) 
 B_SPLINE_SURFACE_WITH_KNOTS ( ( 4, 2, 4 ),
 ( 3, 3 ),
 ( 0.000000000000000000, 0.0003754691837024766443, 0.0007509383674049532886 ),
 ( 0.000000000000000000, 1.000000000000000000 ),
 .UNSPECIFIED. ) 
 GEOMETRIC_REPRESENTATION_ITEM ( )  RATIONAL_B_SPLINE_SURFACE ( (
 ( 1.000000000000000000, 0.6711954675835484219, 1.000000000000000000),
 ( 1.000000000000000000, 0.6709646295267468474, 1.000000000000000000),
 ( 1.000000000000000000, 0.6771840716659200954, 1.000000000000000000),
 ( 1.000000000000000000, 0.6927481755867312962, 1.000000000000000000),
 ( 1.000000000000000000, 0.7017972101310044897, 1.000000000000000000),
 ( 1.000000000000000000, 0.7071067811865475727, 1.000000000000000000) ) ) 
 REPRESENTATION_ITEM ( '' )  SURFACE ( )  );
#139739=CARTESIAN_POINT ( 'NONE',  ( 11.92078253488439721, 7.617083250100837866, -0.8769071248199897806 ) ) ;
#139754=VECTOR ( 'NONE', #122914, 1000.000000000000000 ) ;
#139770=CARTESIAN_POINT ( 'NONE',  ( -11.60067993250125262, 4.148157162114866736, 5.314938114050354656 ) ) ;
#139771=ORIENTED_EDGE ( 'NONE', *, *, #72931, .T. ) ;
#139784=VERTEX_POINT ( 'NONE', #154073 ) ;
#139785=DIRECTION ( 'NONE',  ( -0.000000000000000000, 1.000000000000000000, 9.023263958591317418E-17 ) ) ;
#139797=EDGE_CURVE ( 'NONE', #48021, #9929, #139979, .T. ) ;
#139804=FILL_AREA_STYLE_COLOUR ( '', #22113 ) ;
#139807=CARTESIAN_POINT ( 'NONE',  ( 11.84668730067608600, 10.90000000000000036, -1.400000000000001910 ) ) ;
#139829=EDGE_CURVE ( 'NONE', #121570, #73222, #1976, .T. ) ;
#139834=CARTESIAN_POINT ( 'NONE',  ( 11.48243876534946217, 13.79999999999999893, -3.200000000000001510 ) ) ;
#139854=VERTEX_POINT ( 'NONE', #156217 ) ;
#139872=FACE_OUTER_BOUND ( 'NONE', #197346, .T. ) ;
#139888=CARTESIAN_POINT ( 'NONE',  ( -11.86239285000045918, 13.88000000000000078, -1.812080536912753059 ) ) ;
#139895=CARTESIAN_POINT ( 'NONE',  ( 0.000000000000000000, 14.48195938056239385, 0.000000000000000000 ) ) ;
#139904=CARTESIAN_POINT ( 'NONE',  ( -10.92046113480654768, 4.688422163420479016, 4.459782501114215592 ) ) ;
#139906=CARTESIAN_POINT ( 'NONE',  ( -11.48767021851170078, 9.769957725361562595, 3.470194894594595070 ) ) ;
#139910=EDGE_CURVE ( 'NONE', #1117, #210323, #66243, .T. ) ;
#139919=CARTESIAN_POINT ( 'NONE',  ( 11.95360554405576714, 12.49555003497412464, 1.059413164304728872 ) ) ;
#139931=DIRECTION ( 'NONE',  ( 0.000000000000000000, 1.000000000000000000, 0.000000000000000000 ) ) ;
#139953=CARTESIAN_POINT ( 'NONE',  ( 11.88168509644349058, 13.87999999999997947, 1.685788023084328513 ) ) ;
#139957=VERTEX_POINT ( 'NONE', #90149 ) ;
#139962=DIRECTION ( 'NONE',  ( 0.000000000000000000, 1.000000000000000000, 0.000000000000000000 ) ) ;
#139979=LINE ( 'NONE', #72801, #64326 ) ;
#140080=CARTESIAN_POINT ( 'NONE',  ( -10.52284959769361805, 5.420271152154175986, 5.071911021504272199 ) ) ;
#140084=CARTESIAN_POINT ( 'NONE',  ( -9.367496997694898297, 14.53091781612142697, -7.499999999878477652 ) ) ;
#140091=VERTEX_POINT ( 'NONE', #73110 ) ;
#140119=STYLED_ITEM ( 'NONE', ( #213143 ), #136503 ) ;
#140139=CARTESIAN_POINT ( 'NONE',  ( -11.41381675112453209, 10.90000000000000036, -3.704697986577182078 ) ) ;
#140156=CARTESIAN_POINT ( 'NONE',  ( -11.48243876534946040, 13.79999999999998295, 3.199999999999997957 ) ) ;
#140161=ADVANCED_FACE ( 'NONE', ( #91545 ), #208447, .F. ) ;
#140169=CARTESIAN_POINT ( 'NONE',  ( 9.873106300043385630, 9.984546488800495112, -6.331846131734216065 ) ) ;
#140173=CARTESIAN_POINT ( 'NONE',  ( -11.33772463945043540, 10.19999999999999041, -3.600000000000078693 ) ) ;
#140184=ORIENTED_EDGE ( 'NONE', *, *, #23869, .F. ) ;
#140204=AXIS2_PLACEMENT_3D ( 'NONE', #186845, #102402, #103475 ) ;
#140216=CARTESIAN_POINT ( 'NONE',  ( 11.86239285000045740, 12.22000000000000064, -1.812080536912752837 ) ) ;
#140226=DIRECTION ( 'NONE',  ( 0.000000000000000000, 0.000000000000000000, -1.000000000000000000 ) ) ;
#140256=CIRCLE ( 'NONE', #188773, 11.92000000000000171 ) ;
#140260=CARTESIAN_POINT ( 'NONE',  ( -11.44789321844504215, 11.29999999999998295, 3.303298730975396946 ) ) ;
#140273=CARTESIAN_POINT ( 'NONE',  ( 0.000000000000000000, 15.00000000000000000, 0.000000000000000000 ) ) ;
#140278=CARTESIAN_POINT ( 'NONE',  ( -11.41381675112460847, 12.56983264508524201, -3.704697986577268232 ) ) ;
#140288=UNCERTAINTY_MEASURE_WITH_UNIT (LENGTH_MEASURE( 1.000000000000000082E-05 ), #112870, 'distance_accuracy_value', 'NONE');
#140301=FACE_OUTER_BOUND ( 'NONE', #164103, .T. ) ;
#140314=CARTESIAN_POINT ( 'NONE',  ( -11.88671056400589521, 6.998741290788587754, 4.405061004403326486 ) ) ;
#140320=CARTESIAN_POINT ( 'NONE',  ( 11.01135777277262306, 10.89999999999998259, 1.399999999999998579 ) ) ;
#140333=VERTEX_POINT ( 'NONE', #172407 ) ;
#140341=CARTESIAN_POINT ( 'NONE',  ( 9.472186069782596363, 13.10071810221855593, 7.368474063948833752 ) ) ;
#140371=AXIS2_PLACEMENT_3D ( 'NONE', #185533, #136812, #68572 ) ;
#140389=TRIMMED_CURVE ( 'NONE', #76129, ( PARAMETER_VALUE ( 0.000000000000000000 ), #186838 ), ( PARAMETER_VALUE ( 0.6154797086703889253 ), #190045 ), .T., .PARAMETER. ) ;
#140390=CARTESIAN_POINT ( 'NONE',  ( -9.345718720454827988, 14.55697459676220795, -7.452154232107646159 ) ) ;
#140407=AXIS2_PLACEMENT_3D ( 'NONE', #77847, #159105, #10708 ) ;
#140422=CARTESIAN_POINT ( 'NONE',  ( -9.812680342707254866, 4.108039100808300148, -6.337802944732694677 ) ) ;
#140429=CIRCLE ( 'NONE', #47028, 11.95586200173895008 ) ;
#140435=CARTESIAN_POINT ( 'NONE',  ( -11.21884318011362147, 9.005685702144777594, -2.479759622982018463 ) ) ;
#140439=ORIENTED_EDGE ( 'NONE', *, *, #81935, .F. ) ;
#140441=FILL_AREA_STYLE_COLOUR ( '', #76762 ) ;
#140455=CARTESIAN_POINT ( 'NONE',  ( 0.000000000000000000, 7.980384757729337863, 0.000000000000000000 ) ) ;
#140457=CARTESIAN_POINT ( 'NONE',  ( -11.86239285000045918, 12.21999999999998288, 1.812080536912751283 ) ) ;
#140478=CARTESIAN_POINT ( 'NONE',  ( 11.86145016429272836, 10.19999999999999929, -1.100000000000000311 ) ) ;
#140509=CARTESIAN_POINT ( 'NONE',  ( -10.81659741420782872, 5.544487526538591560, -6.534070432124610583 ) ) ;
#140513=CARTESIAN_POINT ( 'NONE',  ( 11.04536101718726293, 10.19999999999999929, 1.099999999999996758 ) ) ;
#140514=ORIENTED_EDGE ( 'NONE', *, *, #138983, .F. ) ;
#140530=DIRECTION ( 'NONE',  ( 1.000000000000000000, -0.000000000000000000, -0.000000000000000000 ) ) ;
#140563=( GEOMETRIC_REPRESENTATION_CONTEXT ( 3 ) GLOBAL_UNCERTAINTY_ASSIGNED_CONTEXT ( ( #157336 ) ) GLOBAL_UNIT_ASSIGNED_CONTEXT ( ( #54350, #72712, #58609 ) ) REPRESENTATION_CONTEXT ( 'NONE', 'WORKASPACE' ) );
#140565=EDGE_LOOP ( 'NONE', ( #19427, #68716, #118, #58964 ) ) ;
#140575=CARTESIAN_POINT ( 'NONE',  ( 8.990221719931399846, 12.33023651109059493, 7.951427823052896748 ) ) ;
#140576=( GEOMETRIC_REPRESENTATION_CONTEXT ( 3 ) GLOBAL_UNCERTAINTY_ASSIGNED_CONTEXT ( ( #3315 ) ) GLOBAL_UNIT_ASSIGNED_CONTEXT ( ( #57416, #152783, #24897 ) ) REPRESENTATION_CONTEXT ( 'NONE', 'WORKASPACE' ) );
#140577=EDGE_CURVE ( 'NONE', #134499, #204806, #202736, .T. ) ;
#140592=CARTESIAN_POINT ( 'NONE',  ( 11.86239285000045562, 9.799999999999982947, 1.812080536912751061 ) ) ;
#140594=VERTEX_POINT ( 'NONE', #7744 ) ;
#140601=FACE_OUTER_BOUND ( 'NONE', #112797, .T. ) ;
#140613=CARTESIAN_POINT ( 'NONE',  ( -10.85954583250327588, 4.658451743348587470, -5.107361846340859657 ) ) ;
#140627=CARTESIAN_POINT ( 'NONE',  ( -0.008622031262367491067, 15.44736672593548299, 11.95585889282746450 ) ) ;
#140635=DIRECTION ( 'NONE',  ( 0.000000000000000000, 1.000000000000000000, 0.000000000000000000 ) ) ;
#140649=STYLED_ITEM ( 'NONE', ( #125270 ), #15532 ) ;
#140668=VERTEX_POINT ( 'NONE', #173494 ) ;
#140671=CIRCLE ( 'NONE', #182046, 11.09999999999999964 ) ;
#140689=DIRECTION ( 'NONE',  ( 0.000000000000000000, 0.000000000000000000, 1.000000000000000000 ) ) ;
#140705=( NAMED_UNIT ( * ) SI_UNIT ( $, .STERADIAN. ) SOLID_ANGLE_UNIT ( ) );
#140706=CARTESIAN_POINT ( 'NONE',  ( -11.69053533621101160, 4.400474013969419396, 5.144636342886200531 ) ) ;
#140715=ORIENTED_EDGE ( 'NONE', *, *, #130589, .T. ) ;
#140722=EDGE_CURVE ( 'NONE', #66223, #20303, #109386, .T. ) ;
#140731=DIRECTION ( 'NONE',  ( 0.000000000000000000, 1.000000000000000000, 0.000000000000000000 ) ) ;
#140741=ORIENTED_EDGE ( 'NONE', *, *, #35015, .F. ) ;
#140747=CARTESIAN_POINT ( 'NONE',  ( -15.75000000000000000, 11.29999999999999893, 0.6999999999999992895 ) ) ;
#140748=SURFACE_STYLE_FILL_AREA ( #10685 ) ;
#140755=CARTESIAN_POINT ( 'NONE',  ( -11.04978080397792972, 12.49155475012286942, 1.057339094031728211 ) ) ;
#140760=SURFACE_STYLE_USAGE ( .BOTH. , #74656 ) ;
#140768=CARTESIAN_POINT ( 'NONE',  ( 11.94105721237523277, 12.69999999999999929, 1.187919463087244720 ) ) ;
#140775=EDGE_LOOP ( 'NONE', ( #212845, #84063, #31714, #191559 ) ) ;
#140783=SURFACE_STYLE_USAGE ( .BOTH. , #74681 ) ;
#140796=B_SPLINE_CURVE_WITH_KNOTS ( 'NONE', 3,
 ( #79431, #32817, #98891, #13357, #149772, #66343 ),
 .UNSPECIFIED., .F., .F.,
 ( 4, 2, 4 ),
 ( 0.000000000000000000, 0.0003258677429877279035, 0.0006517354859754558071 ),
 .UNSPECIFIED. ) ;
#140802=CARTESIAN_POINT ( 'NONE',  ( -3.505341441177800554, 15.51968381638693195, 11.48538216724446670 ) ) ;
#140804=CARTESIAN_POINT ( 'NONE',  ( -11.89835103415199313, 9.771069141675340575, -1.561208891256348652 ) ) ;
#140816=CARTESIAN_POINT ( 'NONE',  ( 9.767704153745652818, 11.88520199868856331, 6.893175014280387813 ) ) ;
#140821=CARTESIAN_POINT ( 'NONE',  ( -11.89942855770814134, 13.79999999999999893, -0.7000000000000009548 ) ) ;
#140825=AXIS2_PLACEMENT_3D ( 'NONE', #100489, #153523, #38703 ) ;
#140886=CARTESIAN_POINT ( 'NONE',  ( 1.734723475976807094E-15, 14.53394254119687012, 11.91973154060107376 ) ) ;
#140900=CARTESIAN_POINT ( 'NONE',  ( -11.04986227068298277, 12.49060002155663973, -1.056429153205399984 ) ) ;
#140905=B_SPLINE_CURVE_WITH_KNOTS ( 'NONE', 3,
 ( #102192, #168259, #152020, #202863, #53435, #119573, #185559, #103263, #37187, #115312, #20910, #87004, #181302, #165060, #32930, #142195 ),
 .UNSPECIFIED., .F., .F.,
 ( 4, 2, 2, 2, 2, 2, 2, 4 ),
 ( -5.999999999627471727E-08, 0.001048291479606053029, 0.001572467219409077197, 0.002096642959212101365, 0.002620818699015125749, 0.003144994438818149267, 0.003669170178621173652, 0.004193345918424198036 ),
 .UNSPECIFIED. ) ;
#140907=CARTESIAN_POINT ( 'NONE',  ( 11.89321938400731149, 12.33744721639322783, 1.599605898944313154 ) ) ;
#140908=CARTESIAN_POINT ( 'NONE',  ( -10.97030319645364749, 11.30000000000000071, -1.695206765504804869 ) ) ;
#140933=CARTESIAN_POINT ( 'NONE',  ( 10.62873463776380056, 13.79999999999998295, 3.199999999999997957 ) ) ;
#140935=DIRECTION ( 'NONE',  ( 0.000000000000000000, 1.000000000000000000, 0.000000000000000000 ) ) ;
#140974=CARTESIAN_POINT ( 'NONE',  ( -11.80235830595198010, 13.79999999999999893, -1.696088231482795416 ) ) ;
#140977=ORIENTED_EDGE ( 'NONE', *, *, #126509, .F. ) ;
#140993=CARTESIAN_POINT ( 'NONE',  ( 9.663580702207960726, 13.51594383518721365, 8.187698013202092895 ) ) ;
#141025=TOROIDAL_SURFACE ( 'NONE', #9549, 11.92000000000000171, 0.08000000000000000167 ) ;
#141040=DIRECTION ( 'NONE',  ( 0.000000000000000000, 0.000000000000000000, -1.000000000000000000 ) ) ;
#141045=CARTESIAN_POINT ( 'NONE',  ( 0.000000000000000000, 13.88000000000000078, 0.000000000000000000 ) ) ;
#141086=CYLINDRICAL_SURFACE ( 'NONE', #211641, 0.3999999999999993006 ) ;
#141102=CARTESIAN_POINT ( 'NONE',  ( 7.895893545578077877, 15.33679876036382694, 9.037963944523932369 ) ) ;
#141106=PLANE ( 'NONE',  #82833 ) ;
#141107=CARTESIAN_POINT ( 'NONE',  ( 0.000000000000000000, 3.481548657788669843, 0.000000000000000000 ) ) ;
#141119=CARTESIAN_POINT ( 'NONE',  ( -9.898321827454534372, 14.00000000001253930, -7.924999999986504839 ) ) ;
#141124=CARTESIAN_POINT ( 'NONE',  ( 1.464677571780234644E-15, 19.00000000000000000, -11.92000000000000171 ) ) ;
#141130=AXIS2_PLACEMENT_3D ( 'NONE', #145287, #28291, #130144 ) ;
#141146=CIRCLE ( 'NONE', #196446, 11.92000000000000171 ) ;
#141166=CARTESIAN_POINT ( 'NONE',  ( -10.47476534206535170, 5.237283261923990629, -5.169982392003922733 ) ) ;
#141170=CARTESIAN_POINT ( 'NONE',  ( -5.973438521925780620, 14.55272270109815835, -10.36619016570325869 ) ) ;
#141179=( GEOMETRIC_REPRESENTATION_CONTEXT ( 3 ) GLOBAL_UNCERTAINTY_ASSIGNED_CONTEXT ( ( #189810 ) ) GLOBAL_UNIT_ASSIGNED_CONTEXT ( ( #31192, #44251, #207788 ) ) REPRESENTATION_CONTEXT ( 'NONE', 'WORKASPACE' ) );
#141232=CARTESIAN_POINT ( 'NONE',  ( 11.07790593930098311, 9.799999999999998934, 0.6999999999999992895 ) ) ;
#141236=DIRECTION ( 'NONE',  ( 1.000000000000000000, -0.000000000000000000, -0.000000000000000000 ) ) ;
#141246=EDGE_LOOP ( 'NONE', ( #77103, #198337, #102589, #57827 ) ) ;
#141254=CARTESIAN_POINT ( 'NONE',  ( 9.244745934994428538, 11.58786253049815329, -7.169110776657137585 ) ) ;
#141268=ORIENTED_EDGE ( 'NONE', *, *, #212491, .F. ) ;
#141270=CARTESIAN_POINT ( 'NONE',  ( 9.622977958535885890, 4.242291508015296309, -7.169920593678716259 ) ) ;
#141278=AXIS2_PLACEMENT_3D ( 'NONE', #3217, #34673, #136466 ) ;
#141283=EDGE_CURVE ( 'NONE', #115079, #113953, #154146, .T. ) ;
#141313=CARTESIAN_POINT ( 'NONE',  ( 1.050790385994998077, 14.00000000000000533, 12.64745918785790302 ) ) ;
#141351=ADVANCED_FACE ( 'NONE', ( #70338 ), #23738, .T. ) ;
#141353=CARTESIAN_POINT ( 'NONE',  ( 8.662485680320882508, 14.42234338554197315, 8.322065852714080947 ) ) ;
#141361=CARTESIAN_POINT ( 'NONE',  ( 9.672792005750940447, 13.47495944640959920, 8.176450814826708324 ) ) ;
#141380=EDGE_CURVE ( 'NONE', #156687, #48021, #63597, .T. ) ;
#141381=CARTESIAN_POINT ( 'NONE',  ( 11.97185388258315086, 9.720000092796073687, 0.8311143155443657671 ) ) ;
#141386=DIRECTION ( 'NONE',  ( 0.000000000000000000, 0.000000000000000000, -1.000000000000000000 ) ) ;
#141395=CARTESIAN_POINT ( 'NONE',  ( -12.65289843835643069, 8.694282390621570045, -1.237672713095353982 ) ) ;
#141423=CARTESIAN_POINT ( 'NONE',  ( 9.427850895902821549, 13.54474674066948126, 7.423989997610757285 ) ) ;
#141469=SURFACE_SIDE_STYLE ('',( #75357 ) ) ;
#141498=AXIS2_PLACEMENT_3D ( 'NONE', #68402, #132406, #65207 ) ;
#141502=FACE_OUTER_BOUND ( 'NONE', #20927, .T. ) ;
#141510=CARTESIAN_POINT ( 'NONE',  ( 11.04536101718726293, 10.90000000000000036, -1.100000000000002087 ) ) ;
#141511=CARTESIAN_POINT ( 'NONE',  ( -10.37109829931902816, 6.927524423111719898, -5.134218648570218591 ) ) ;
#141526=VERTEX_POINT ( 'NONE', #31223 ) ;
#141528=SURFACE_SIDE_STYLE ('',( #75415 ) ) ;
#141576=SURFACE_STYLE_FILL_AREA ( #59203 ) ;
#141581=CARTESIAN_POINT ( 'NONE',  ( -9.645452764996941042, 5.068254855380425639, -6.574395040668256307 ) ) ;
#141586=CARTESIAN_POINT ( 'NONE',  ( -15.75000000000000000, 11.29999999999999893, -3.200000000000001510 ) ) ;
#141590=DIRECTION ( 'NONE',  ( 0.9982742078614211811, 0.000000000000000000, -0.05872483221476467591 ) ) ;
#141670=SURFACE_SIDE_STYLE ('',( #173075 ) ) ;
#141678=CARTESIAN_POINT ( 'NONE',  ( 11.94650005372637835, 11.15102700337638097, 1.135399707157307203 ) ) ;
#141679=CARTESIAN_POINT ( 'NONE',  ( 10.35986303813127307, 9.178481322669741260, 6.010608889982933078 ) ) ;
#141686=CARTESIAN_POINT ( 'NONE',  ( -9.404393215816320151, 14.49025778602134551, -7.453732457429351754 ) ) ;
#141692=AXIS2_PLACEMENT_3D ( 'NONE', #77974, #162441, #191711 ) ;
#141698=CARTESIAN_POINT ( 'NONE',  ( 8.029509147085835963, 15.33973900756292252, -8.919384641555231141 ) ) ;
#141700=CARTESIAN_POINT ( 'NONE',  ( -15.75000000000000000, 13.40000000000000036, 1.099999999999996758 ) ) ;
#141709=( NAMED_UNIT ( * ) PLANE_ANGLE_UNIT ( ) SI_UNIT ( $, .RADIAN. ) );
#141772=CARTESIAN_POINT ( 'NONE',  ( 9.687436728043250511, 13.40831512142563042, -8.157569025435085663 ) ) ;
#141774=CARTESIAN_POINT ( 'NONE',  ( -10.52476609942256758, 3.676887381874808902, 5.198941853688804571 ) ) ;
#141855=( LENGTH_UNIT ( ) NAMED_UNIT ( * ) SI_UNIT ( .MILLI., .METRE. ) );
#141871=CARTESIAN_POINT ( 'NONE',  ( 0.05548385694414996461, 15.44694884557249459, 11.95573287483746583 ) ) ;
#141873=CARTESIAN_POINT ( 'NONE',  ( -11.92046840572485777, 9.947478752057296703, -1.382231356234943309 ) ) ;
#141883=DIRECTION ( 'NONE',  ( 0.000000000000000000, -0.000000000000000000, 1.000000000000000000 ) ) ;
#141884=CARTESIAN_POINT ( 'NONE',  ( 11.92046840572485777, 11.15252124794270649, -1.382231356234943753 ) ) ;
#141885=CARTESIAN_POINT ( 'NONE',  ( 11.90252275860789588, 7.647352740710921637, -1.095560775704444323 ) ) ;
#141889=LINE ( 'NONE', #207898, #81869 ) ;
#141907=( NAMED_UNIT ( * ) SI_UNIT ( $, .STERADIAN. ) SOLID_ANGLE_UNIT ( ) );
#141914=CARTESIAN_POINT ( 'NONE',  ( -0.01291931824900539524, 15.45162602843430300, 11.96434918058137242 ) ) ;
#141919=EDGE_CURVE ( 'NONE', #176022, #23505, #49140, .T. ) ;
#141933=CARTESIAN_POINT ( 'NONE',  ( -11.41381675112453387, 10.19999999999998153, 3.704697986577180746 ) ) ;
#141963=CARTESIAN_POINT ( 'NONE',  ( -4.304844010029503565, 14.48099179547451953, 11.21040724251216325 ) ) ;
#141969=CARTESIAN_POINT ( 'NONE',  ( -11.80251051724219202, 11.29999999999998117, 1.695257889419070851 ) ) ;
#141975=FILL_AREA_STYLE ('',( #41260 ) ) ;
#142008=CARTESIAN_POINT ( 'NONE',  ( -11.43209210103587914, 11.15596075983916080, -3.649125173352125273 ) ) ;
#142047=CARTESIAN_POINT ( 'NONE',  ( -11.41381675112453387, 10.19999999999998153, 3.704697986577180302 ) ) ;
#142062=CARTESIAN_POINT ( 'NONE',  ( 11.97929049433705728, 12.22000000000000064, 0.7046979865771804130 ) ) ;
#142072=CARTESIAN_POINT ( 'NONE',  ( -11.48243876534946040, 13.79999999999999893, -3.200000000000001510 ) ) ;
#142097=SURFACE_STYLE_FILL_AREA ( #109640 ) ;
#142123=CARTESIAN_POINT ( 'NONE',  ( 11.89321938400742340, 11.26255278360675227, -1.599605898944273852 ) ) ;
#142155=CARTESIAN_POINT ( 'NONE',  ( 8.022420187971052385, 15.29110919921158285, 8.925725321005275603 ) ) ;
#142158=CARTESIAN_POINT ( 'NONE',  ( -15.75000000000000000, 9.799999999999998934, -1.800000000000001155 ) ) ;
#142165=ORIENTED_EDGE ( 'NONE', *, *, #19530, .F. ) ;
#142181=VECTOR ( 'NONE', #107321, 1000.000000000000000 ) ;
#142195=CARTESIAN_POINT ( 'NONE',  ( 9.348761378620915607, 13.52553930298125096, -7.449808453853658641 ) ) ;
#142219=DIRECTION ( 'NONE',  ( -0.000000000000000000, 0.000000000000000000, -1.000000000000000000 ) ) ;
#142224=CARTESIAN_POINT ( 'NONE',  ( -11.86145016429273191, 10.09412123665269334, -1.100000000000000089 ) ) ;
#142227=DIRECTION ( 'NONE',  ( 0.000000000000000000, -1.000000000000000000, 0.000000000000000000 ) ) ;
#142278=COLOUR_RGB ( '', 0.66274510, 0.83137255, 0.94901961) ;
#142279=CARTESIAN_POINT ( 'NONE',  ( -11.44786932348563901, 11.29999999999999893, -3.303370173849772051 ) ) ;
#142281=CARTESIAN_POINT ( 'NONE',  ( 1.500000000000053291, 7.750000000000000000, 15.74999999999999289 ) ) ;
#142292=CARTESIAN_POINT ( 'NONE',  ( 10.72462670916096172, 9.912391986280232103, -5.392981251122232145 ) ) ;
#142299=CARTESIAN_POINT ( 'NONE',  ( -11.41126283316785361, 13.75874606908456954, 3.405403429622881006 ) ) ;
#142301=SURFACE_SIDE_STYLE ('',( #76192 ) ) ;
#142303=ORIENTED_EDGE ( 'NONE', *, *, #157010, .T. ) ;
#142311=CARTESIAN_POINT ( 'NONE',  ( 10.23763000547997493, 9.286261708574206963, 5.789277571301806979 ) ) ;
#142314=ORIENTED_EDGE ( 'NONE', *, *, #74394, .F. ) ;
#142317=EDGE_LOOP ( 'NONE', ( #43890, #117276, #202539, #24660 ) ) ;
#142334=STYLED_ITEM ( 'NONE', ( #196189 ), #60737 ) ;
#142360=EDGE_CURVE ( 'NONE', #158767, #23152, #178560, .T. ) ;
#142371=CARTESIAN_POINT ( 'NONE',  ( -8.065673738749977062, 13.99999998464209305, 8.613976760017859391 ) ) ;
#142386=VERTEX_POINT ( 'NONE', #99967 ) ;
#142414=CARTESIAN_POINT ( 'NONE',  ( -11.41381675112453387, 12.69999999999999929, -3.704697986577184299 ) ) ;
#142416=CARTESIAN_POINT ( 'NONE',  ( 9.271941217832353033, 15.45702117623653749, 8.565526717805919787 ) ) ;
#142440=( LENGTH_UNIT ( ) NAMED_UNIT ( * ) SI_UNIT ( .MILLI., .METRE. ) );
#142449=CARTESIAN_POINT ( 'NONE',  ( -10.88575987782614796, 5.812703298851592315, -6.395352192321499984 ) ) ;
#142473=CARTESIAN_POINT ( 'NONE',  ( 11.62584726340593377, 8.214503055780935981, 3.002169211754254885 ) ) ;
#142485=AXIS2_PLACEMENT_3D ( 'NONE', #47831, #61923, #95519 ) ;
#142518=( NAMED_UNIT ( * ) PLANE_ANGLE_UNIT ( ) SI_UNIT ( $, .RADIAN. ) );
#142521=CARTESIAN_POINT ( 'NONE',  ( -11.12441040585762408, 5.813956397379768326, 4.514688396320016395 ) ) ;
#142535=( NAMED_UNIT ( * ) PLANE_ANGLE_UNIT ( ) SI_UNIT ( $, .RADIAN. ) );
#142553=CARTESIAN_POINT ( 'NONE',  ( -9.470156251935129887, 4.005132839944305800, -6.837168546664702085 ) ) ;
#142562=CARTESIAN_POINT ( 'NONE',  ( -11.68287950975655676, 8.167437761341201252, 4.460353674290588266 ) ) ;
#142567=CARTESIAN_POINT ( 'NONE',  ( 7.694789056592527210, 14.38989046813754946, 9.211249139029591859 ) ) ;
#142592=LINE ( 'NONE', #157756, #62926 ) ;
#142608=EDGE_CURVE ( 'NONE', #41918, #11599, #171924, .T. ) ;
#142630=PLANE ( 'NONE',  #158706 ) ;
#142636=CARTESIAN_POINT ( 'NONE',  ( -10.82855876678636520, 5.585670971531701667, -6.509986581443756748 ) ) ;
#142682=( GEOMETRIC_REPRESENTATION_CONTEXT ( 3 ) GLOBAL_UNCERTAINTY_ASSIGNED_CONTEXT ( ( #213995 ) ) GLOBAL_UNIT_ASSIGNED_CONTEXT ( ( #101529, #72206, #2931 ) ) REPRESENTATION_CONTEXT ( 'NONE', 'WORKASPACE' ) );
#142698=B_SPLINE_CURVE_WITH_KNOTS ( 'NONE', 3,
 ( #74523, #123363, #22538, #75588, #142757, #44168, #126554, #192515, #89725, #24682, #58270, #141698, #205564, #90787, #88646, #154705 ),
 .UNSPECIFIED., .F., .F.,
 ( 4, 2, 2, 2, 2, 2, 2, 4 ),
 ( 0.000000000000000000, 0.0005319996970288863375, 0.001063999394057772675, 0.001595999091086659121, 0.002127998788115545350, 0.002659998485144431796, 0.003191998182173318242, 0.004255997576231089832 ),
 .UNSPECIFIED. ) ;
#142717=VERTEX_POINT ( 'NONE', #205474 ) ;
#142730=DIRECTION ( 'NONE',  ( 0.000000000000000000, -1.000000000000000000, 0.000000000000000000 ) ) ;
#142735=LINE ( 'NONE', #90771, #113830 ) ;
#142739=( GEOMETRIC_REPRESENTATION_CONTEXT ( 3 ) GLOBAL_UNCERTAINTY_ASSIGNED_CONTEXT ( ( #33203 ) ) GLOBAL_UNIT_ASSIGNED_CONTEXT ( ( #161297, #127823, #75775 ) ) REPRESENTATION_CONTEXT ( 'NONE', 'WORKASPACE' ) );
#142746=CARTESIAN_POINT ( 'NONE',  ( -9.383881589528572320, 14.59418599432876640, -7.387911200823596758 ) ) ;
#142757=CARTESIAN_POINT ( 'NONE',  ( 9.175343923411263702, 14.33640814621786674, -7.734832872067204157 ) ) ;
#142760=SURFACE_STYLE_FILL_AREA ( #76644 ) ;
#142779=CARTESIAN_POINT ( 'NONE',  ( 9.327139308102928794, 13.85903420602375036, -7.550757598840666773 ) ) ;
#142831=CARTESIAN_POINT ( 'NONE',  ( 11.25027063990047616, 9.330753595378251219, 3.765175919509110791 ) ) ;
#142832=CIRCLE ( 'NONE', #28699, 11.92000000000000171 ) ;
#142833=CARTESIAN_POINT ( 'NONE',  ( -10.39320420135713263, 4.932286138528427344, 5.331284845095887626 ) ) ;
#142846=B_SPLINE_CURVE_WITH_KNOTS ( 'NONE', 3,
 ( #122361, #6355, #72425, #23682, #155838, #107144 ),
 .UNSPECIFIED., .F., .F.,
 ( 4, 2, 4 ),
 ( 0.000000000000000000, 0.0003845013059668469482, 0.0007690026119336938965 ),
 .UNSPECIFIED. ) ;
#142858=CARTESIAN_POINT ( 'NONE',  ( 9.333039360705550180, 4.446953957879813402, -7.472411811099956225 ) ) ;
#142884=VECTOR ( 'NONE', #83222, 1000.000000000000000 ) ;
#142902=CARTESIAN_POINT ( 'NONE',  ( 0.000000000000000000, 15.00000000000000000, 0.000000000000000000 ) ) ;
#142906=CARTESIAN_POINT ( 'NONE',  ( -10.72721294398669123, 4.499566226064992236, 5.280202143233098333 ) ) ;
#142937=VECTOR ( 'NONE', #166629, 1000.000000000000000 ) ;
#142941=DIRECTION ( 'NONE',  ( -0.000000000000000000, -1.000000000000000000, -0.000000000000000000 ) ) ;
#142946=VECTOR ( 'NONE', #114890, 1000.000000000000000 ) ;
#142948=SURFACE_STYLE_FILL_AREA ( #24875 ) ;
#142970=CARTESIAN_POINT ( 'NONE',  ( 11.84668730067608244, 11.00636224908217287, 1.399999999999998357 ) ) ;
#143012=CARTESIAN_POINT ( 'NONE',  ( -10.62873463776380056, 12.30000000000000071, -3.200000000000001510 ) ) ;
#143013=AXIS2_PLACEMENT_3D ( 'NONE', #203956, #207180, #175772 ) ;
#143015=STYLED_ITEM ( 'NONE', ( #23309 ), #113029 ) ;
#143046=SURFACE_STYLE_FILL_AREA ( #141975 ) ;
#143061=EDGE_LOOP ( 'NONE', ( #48010, #37690, #129046, #21288 ) ) ;
#143081=CARTESIAN_POINT ( 'NONE',  ( 11.01135777277262306, 0.000000000000000000, 1.399999999999998579 ) ) ;
#143084=EDGE_CURVE ( 'NONE', #156205, #163314, #27803, .T. ) ;
#143086=SURFACE_STYLE_USAGE ( .BOTH. , #44496 ) ;
#143105=CARTESIAN_POINT ( 'NONE',  ( 11.48243876534946217, 9.799999999999998934, -3.200000000000001510 ) ) ;
#143141=ADVANCED_FACE ( 'NONE', ( #111258, #15792, #176202, #29947, #161008, #78675, #178338 ), #144801, .T. ) ;
#143149=FACE_OUTER_BOUND ( 'NONE', #183558, .T. ) ;
#143157=LINE ( 'NONE', #10954, #179121 ) ;
#143170=CIRCLE ( 'NONE', #67013, 0.08000000000000020983 ) ;
#143171=ADVANCED_FACE ( 'NONE', ( #14732 ), #26635, .T. ) ;
#143176=VECTOR ( 'NONE', #145173, 1000.000000000000000 ) ;
#143180=ORIENTED_EDGE ( 'NONE', *, *, #206662, .T. ) ;
#143186=EDGE_LOOP ( 'NONE', ( #148170, #171854, #171646, #207060 ) ) ;
#143235=CARTESIAN_POINT ( 'NONE',  ( 8.680911210833158975, 14.87390181681097090, 8.226265084022907459 ) ) ;
#143260=ORIENTED_EDGE ( 'NONE', *, *, #195779, .F. ) ;
#143289=CARTESIAN_POINT ( 'NONE',  ( 11.55950211276791428, 11.37999999999998302, 3.221476510067112109 ) ) ;
#143300=CARTESIAN_POINT ( 'NONE',  ( -0.8991744117087477894, 14.53091782053303049, -11.99999999953292296 ) ) ;
#143324=CARTESIAN_POINT ( 'NONE',  ( -11.48243876534946040, 11.29999999999999893, -3.200000000000001510 ) ) ;
#143335=SURFACE_STYLE_FILL_AREA ( #108729 ) ;
#143356=CARTESIAN_POINT ( 'NONE',  ( 11.01135777277262306, 10.89999999999998259, 1.399999999999998579 ) ) ;
#143357=ORIENTED_EDGE ( 'NONE', *, *, #117333, .T. ) ;
#143363=CARTESIAN_POINT ( 'NONE',  ( 11.97035325917572379, 7.690326957080006132, -0.8713173324656824370 ) ) ;
#143365=ORIENTED_EDGE ( 'NONE', *, *, #83013, .F. ) ;
#143371=AXIS2_PLACEMENT_3D ( 'NONE', #98438, #13959, #97389 ) ;
#143381=CARTESIAN_POINT ( 'NONE',  ( 8.523843703926681670, 12.47051211315569574, -8.417911888829477718 ) ) ;
#143394=EDGE_CURVE ( 'NONE', #163825, #91840, #30004, .T. ) ;
#143410=CARTESIAN_POINT ( 'NONE',  ( 0.000000000000000000, 11.37999999999999901, 0.000000000000000000 ) ) ;
#143439=CARTESIAN_POINT ( 'NONE',  ( -11.81718632094301746, 7.791935455490584417, 1.824594704062737271 ) ) ;
#143442=CARTESIAN_POINT ( 'NONE',  ( -3.501245407925564823, 14.00000000000089173, 11.28115623562654513 ) ) ;
#143443=FACE_OUTER_BOUND ( 'NONE', #103100, .T. ) ;
#143462=PRESENTATION_STYLE_ASSIGNMENT (( #156483 ) ) ;
#143466=VECTOR ( 'NONE', #103148, 1000.000000000000000 ) ;
#143474=SURFACE_STYLE_USAGE ( .BOTH. , #77360 ) ;
#143483=CARTESIAN_POINT ( 'NONE',  ( 0.000000000000000000, 3.999999999999996447, 0.000000000000000000 ) ) ;
#143487=CARTESIAN_POINT ( 'NONE',  ( 7.320801413324473650, 15.00000000000000000, -10.35317664616355771 ) ) ;
#143490=CARTESIAN_POINT ( 'NONE',  ( 6.978632775467555227, 14.99421780237605795, 9.366897188349161851 ) ) ;
#143509=( BOUNDED_SURFACE ( )  B_SPLINE_SURFACE ( 3, 2, ( 
 ( #66493, #16690, #85980 ),
 ( #83835, #197587, #115350 ),
 ( #53475, #185597, #165099 ),
 ( #181341, #36147, #200767 ),
 ( #148848, #34025, #132633 ),
 ( #32968, #421, #149926 ) ),
 .UNSPECIFIED., .F., .F., .F. ) 
 B_SPLINE_SURFACE_WITH_KNOTS ( ( 4, 2, 4 ),
 ( 3, 3 ),
 ( 0.000000000000000000, 0.0003766405729503174787, 0.0007532811459006349573 ),
 ( 0.000000000000000000, 1.000000000000000000 ),
 .UNSPECIFIED. ) 
 GEOMETRIC_REPRESENTATION_ITEM ( )  RATIONAL_B_SPLINE_SURFACE ( (
 ( 1.000000000000000000, 0.7071067811865551223, 1.000000000000000000),
 ( 1.000000000000000000, 0.7211294902953826469, 1.000000000000000000),
 ( 1.000000000000000000, 0.7311181975230335306, 1.000000000000000000),
 ( 1.000000000000000000, 0.7429553055061443034, 1.000000000000000000),
 ( 1.000000000000000000, 0.7451698531058299491, 1.000000000000000000),
 ( 1.000000000000000000, 0.7452309222762957264, 1.000000000000000000) ) ) 
 REPRESENTATION_ITEM ( '' )  SURFACE ( )  );
#143525=CARTESIAN_POINT ( 'NONE',  ( -11.04445182892037813, 5.143275749589305335, -4.203165840917552742 ) ) ;
#143530=COLOUR_RGB ( '', 0.31764706, 0.68627451, 0.89019608) ;
#143535=AXIS2_PLACEMENT_3D ( 'NONE', #122419, #9627, #28016 ) ;
#143536=ADVANCED_FACE ( 'NONE', ( #52570 ), #87204, .F. ) ;
#143551=CARTESIAN_POINT ( 'NONE',  ( 11.27771153926699377, 8.828701344599535261, -4.118830345813656812 ) ) ;
#143583=ADVANCED_FACE ( 'NONE', ( #139169 ), #8079, .F. ) ;
#143593=CARTESIAN_POINT ( 'NONE',  ( -9.367496997901325173, 14.48154074412966175, -7.499999999620646562 ) ) ;
#143610=CARTESIAN_POINT ( 'NONE',  ( -11.16739129266794350, 7.275426543628465303, -4.398590771924178355 ) ) ;
#143616=VERTEX_POINT ( 'NONE', #55768 ) ;
#143631=CARTESIAN_POINT ( 'NONE',  ( -9.409940793360268785, 3.999985931113709814, -6.919963696468023784 ) ) ;
#143643=CARTESIAN_POINT ( 'NONE',  ( -11.47199464713663453, 5.776720398841780124, 5.393175811422019628 ) ) ;
#143656=EDGE_CURVE ( 'NONE', #141526, #102037, #188905, .T. ) ;
#143674=CARTESIAN_POINT ( 'NONE',  ( -3.104766810201186278, 15.44820807305922195, 11.55390834459370097 ) ) ;
#143713=CARTESIAN_POINT ( 'NONE',  ( 11.33772463945037146, 12.69999999999998153, 3.679999999999999272 ) ) ;
#143734=ORIENTED_EDGE ( 'NONE', *, *, #209881, .F. ) ;
#143773=ORIENTED_EDGE ( 'NONE', *, *, #116113, .F. ) ;
#143789=FILL_AREA_STYLE ('',( #125442 ) ) ;
#143795=CARTESIAN_POINT ( 'NONE',  ( 11.89321938400720491, 9.837447216393373495, 1.599605898944226334 ) ) ;
#143814=CARTESIAN_POINT ( 'NONE',  ( 11.79269373152572342, 6.877189549381032663, -1.951281263922989950 ) ) ;
#143817=FILL_AREA_STYLE ('',( #11622 ) ) ;
#143821=CARTESIAN_POINT ( 'NONE',  ( -9.088333505345289609, 15.51845924943720867, 7.848675090006571153 ) ) ;
#143823=DIRECTION ( 'NONE',  ( 0.000000000000000000, 0.000000000000000000, 1.000000000000000000 ) ) ;
#143840=ADVANCED_FACE ( 'NONE', ( #178072 ), #12342, .F. ) ;
#143844=CARTESIAN_POINT ( 'NONE',  ( -11.84101807917483740, 11.11021500260875250, 1.444039656437077879 ) ) ;
#143853=FACE_OUTER_BOUND ( 'NONE', #188744, .T. ) ;
#143856=CARTESIAN_POINT ( 'NONE',  ( 8.021163746898499980, 15.29143580044878625, -8.926870001462752668 ) ) ;
#143907=CARTESIAN_POINT ( 'NONE',  ( 10.13422073961231185, 13.69230262657889874, -7.310424441678322616 ) ) ;
#143948=CARTESIAN_POINT ( 'NONE',  ( -15.75000000000000000, 10.89999999999998259, 1.799999999999999600 ) ) ;
#143955=VERTEX_POINT ( 'NONE', #109935 ) ;
#143956=EDGE_CURVE ( 'NONE', #211051, #197321, #5831, .T. ) ;
#143974=ADVANCED_FACE ( 'NONE', ( #100795 ), #195385, .T. ) ;
#143976=AXIS2_PLACEMENT_3D ( 'NONE', #102879, #185170, #135390 ) ;
#144017=VERTEX_POINT ( 'NONE', #27540 ) ;
#144031=CARTESIAN_POINT ( 'NONE',  ( -1.499999999999964029, 7.750000000000000000, 10.64483442802189117 ) ) ;
#144044=CARTESIAN_POINT ( 'NONE',  ( 11.84668730067608600, 10.89999999999998259, 1.399999999999998579 ) ) ;
#144057=CARTESIAN_POINT ( 'NONE',  ( -0.07926560466948139039, 15.51761135634724198, 11.99972816967691891 ) ) ;
#144058=CARTESIAN_POINT ( 'NONE',  ( -9.410012541129075814, 4.000000000000001776, 6.919867902370715917 ) ) ;
#144076=ORIENTED_EDGE ( 'NONE', *, *, #85474, .F. ) ;
#144084=ORIENTED_EDGE ( 'NONE', *, *, #80961, .F. ) ;
#144085=CARTESIAN_POINT ( 'NONE',  ( -11.86145016429273724, 11.00587408513255561, -1.100000000000002531 ) ) ;
#144088=VECTOR ( 'NONE', #28840, 1000.000000000000000 ) ;
#144093=EDGE_CURVE ( 'NONE', #3699, #210323, #81937, .T. ) ;
#144118=ORIENTED_EDGE ( 'NONE', *, *, #208749, .T. ) ;
#144120=CARTESIAN_POINT ( 'NONE',  ( 11.52460864928264783, 11.38000000000000078, -3.346683403123526190 ) ) ;
#144130=CARTESIAN_POINT ( 'NONE',  ( 0.000000000000000000, 12.22000000000000064, 0.000000000000000000 ) ) ;
#144142=CARTESIAN_POINT ( 'NONE',  ( 11.33772467203874612, 12.59267152018150426, -3.600000000000000977 ) ) ;
#144155=AXIS2_PLACEMENT_3D ( 'NONE', #62433, #162083, #13672 ) ;
#144187=EDGE_LOOP ( 'NONE', ( #83406, #2199, #180729, #125668, #42928, #107432, #31613, #203946 ) ) ;
#144199=DIRECTION ( 'NONE',  ( 0.000000000000000000, 0.000000000000000000, -1.000000000000000000 ) ) ;
#144204=CARTESIAN_POINT ( 'NONE',  ( -11.97302537858672444, 9.801240101919498571, -0.8111997896468137181 ) ) ;
#144223=FACE_OUTER_BOUND ( 'NONE', #162588, .T. ) ;
#144229=CARTESIAN_POINT ( 'NONE',  ( 11.48243876534946217, 9.799999999999982947, 3.199999999999997957 ) ) ;
#144246=( NAMED_UNIT ( * ) SI_UNIT ( $, .STERADIAN. ) SOLID_ANGLE_UNIT ( ) );
#144257=VERTEX_POINT ( 'NONE', #171133 ) ;
#144259=EDGE_CURVE ( 'NONE', #138814, #204988, #123471, .T. ) ;
#144268=DIRECTION ( 'NONE',  ( -0.5994789404140901112, 2.055006554627987857E-15, 0.8003905296791060664 ) ) ;
#144330=ORIENTED_EDGE ( 'NONE', *, *, #195285, .T. ) ;
#144346=CARTESIAN_POINT ( 'NONE',  ( -11.86145016429273014, 19.00000000000000000, -1.180000000000002158 ) ) ;
#144349=VERTEX_POINT ( 'NONE', #122486 ) ;
#144362=CARTESIAN_POINT ( 'NONE',  ( 11.44786932348564257, 11.29999999999998117, 3.303370173849760061 ) ) ;
#144366=ORIENTED_EDGE ( 'NONE', *, *, #127165, .F. ) ;
#144372=CARTESIAN_POINT ( 'NONE',  ( -11.41381675112453564, 19.00000000000000000, 3.704697986577180746 ) ) ;
#144374=CARTESIAN_POINT ( 'NONE',  ( 11.43190902327453529, 11.15522128257866363, -3.649704988378122739 ) ) ;
#144385=DIRECTION ( 'NONE',  ( -3.491481338843133355E-15, 0.000000000000000000, -1.000000000000000000 ) ) ;
#144390=FACE_OUTER_BOUND ( 'NONE', #41397, .T. ) ;
#144438=CARTESIAN_POINT ( 'NONE',  ( 11.34721833292158699, 8.766100218939394395, 3.908682455922633192 ) ) ;
#144440=EDGE_LOOP ( 'NONE', ( #87771, #66024, #123784, #156635 ) ) ;
#144441=STYLED_ITEM ( 'NONE', ( #120677 ), #151177 ) ;
#144445=DIRECTION ( 'NONE',  ( -0.9885327375000381167, 0.000000000000000000, 0.1510067114093955609 ) ) ;
#144458=CARTESIAN_POINT ( 'NONE',  ( 9.809883170912574002, 12.88719579058855125, -8.001885615786651584 ) ) ;
#144464=ORIENTED_EDGE ( 'NONE', *, *, #20907, .F. ) ;
#144486=CARTESIAN_POINT ( 'NONE',  ( -15.75000000000000000, 12.69999999999998153, 1.399999999999998579 ) ) ;
#144497=B_SPLINE_CURVE_WITH_KNOTS ( 'NONE', 3,
 ( #30261, #212181, #109446, #95283, #96347, #161331 ),
 .UNSPECIFIED., .F., .F.,
 ( 4, 2, 4 ),
 ( 0.000000000000000000, 0.0003767011250903909642, 0.0007534022501807819284 ),
 .UNSPECIFIED. ) ;
#144514=CARTESIAN_POINT ( 'NONE',  ( 0.3554123170485725680, 15.00000000000058265, 12.67999999502907649 ) ) ;
#144525=AXIS2_PLACEMENT_3D ( 'NONE', #175925, #9137, #40588 ) ;
#144526=CARTESIAN_POINT ( 'NONE',  ( 11.06298660227979802, 9.843196003747330280, -0.9087478855431304625 ) ) ;
#144540=CIRCLE ( 'NONE', #47737, 0.08000000000000020983 ) ;
#144544=SURFACE_STYLE_USAGE ( .BOTH. , #28616 ) ;
#144557=CARTESIAN_POINT ( 'NONE',  ( 8.793960880499607669, 13.45135513836973296, -7.698180313484015436 ) ) ;
#144560=CARTESIAN_POINT ( 'NONE',  ( 8.800798923547361596, 13.41831251038806982, 7.690207505967889823 ) ) ;
#144592=CARTESIAN_POINT ( 'NONE',  ( -10.60630588279735242, 5.715763139788331948, 4.896273837757428637 ) ) ;
#144593=VECTOR ( 'NONE', #67100, 1000.000000000000000 ) ;
#144609=CARTESIAN_POINT ( 'NONE',  ( -9.489836703312123589, 15.20205537403712093, 7.238794766165088213 ) ) ;
#144610=VERTEX_POINT ( 'NONE', #93110 ) ;
#144615=ORIENTED_EDGE ( 'NONE', *, *, #91785, .T. ) ;
#144616=CARTESIAN_POINT ( 'NONE',  ( 11.87979087550123758, 7.786822373289821186, -1.749581464211011905 ) ) ;
#144626=PRESENTATION_STYLE_ASSIGNMENT (( #75316 ) ) ;
#144666=CARTESIAN_POINT ( 'NONE',  ( -11.33126667303324275, 6.586199079536864787, -3.816285274238954806 ) ) ;
#144674=CARTESIAN_POINT ( 'NONE',  ( -11.98806725462682721, 9.050750434120253374, 0.6182873949870071328 ) ) ;
#144677=SURFACE_SIDE_STYLE ('',( #27680 ) ) ;
#144695=VECTOR ( 'NONE', #98646, 1000.000000000000000 ) ;
#144707=CARTESIAN_POINT ( 'NONE',  ( -11.38508626655161216, 5.468933214068770532, 5.576081633246319669 ) ) ;
#144711=( LENGTH_UNIT ( ) NAMED_UNIT ( * ) SI_UNIT ( .MILLI., .METRE. ) );
#144721=ORIENTED_EDGE ( 'NONE', *, *, #173138, .T. ) ;
#144723=FACE_OUTER_BOUND ( 'NONE', #96509, .T. ) ;
#144726=CYLINDRICAL_SURFACE ( 'NONE', #130996, 0.3999999999999997446 ) ;
#144728=COLOUR_RGB ( '', 0.08235294, 0.09019608, 0.10196078) ;
#144735=AXIS2_PLACEMENT_3D ( 'NONE', #18913, #100187, #199802 ) ;
#144736=DIRECTION ( 'NONE',  ( -3.706092522800016599E-15, 0.000000000000000000, -1.000000000000000000 ) ) ;
#144781=CARTESIAN_POINT ( 'NONE',  ( -9.587917471435847716, 4.026361754648488223, -6.670783315233271615 ) ) ;
#144801=CYLINDRICAL_SURFACE ( 'NONE', #144155, 12.00000000000000178 ) ;
#144802=ADVANCED_FACE ( 'NONE', ( #128049 ), #211979, .T. ) ;
#144821=UNCERTAINTY_MEASURE_WITH_UNIT (LENGTH_MEASURE( 1.000000000000000082E-05 ), #173998, 'distance_accuracy_value', 'NONE');
#144846=CARTESIAN_POINT ( 'NONE',  ( 11.41381675112453564, 10.06994333910006567, -3.704697986577182522 ) ) ;
#144857=ORIENTED_EDGE ( 'NONE', *, *, #126259, .F. ) ;
#144859=CARTESIAN_POINT ( 'NONE',  ( 11.92051736251533534, 9.948197562073195499, 1.381800029228856808 ) ) ;
#144880=SURFACE_STYLE_USAGE ( .BOTH. , #78756 ) ;
#144884=SURFACE_STYLE_FILL_AREA ( #78760 ) ;
#144902=CARTESIAN_POINT ( 'NONE',  ( 11.35569630219391968, 9.987315607086321378, 3.554478010595061743 ) ) ;
#144913=CARTESIAN_POINT ( 'NONE',  ( 7.221524917713163738, 15.51845925282233196, -9.590549216876459226 ) ) ;
#144946=CARTESIAN_POINT ( 'NONE',  ( -11.41157692552970460, 12.34089662912998620, 3.404533818002359435 ) ) ;
#144952=CARTESIAN_POINT ( 'NONE',  ( 9.022614842422171932, 12.34770622016754515, -7.914810590312522542 ) ) ;
#144961=CARTESIAN_POINT ( 'NONE',  ( 10.14963603790778812, 13.57268984379813936, -7.272210095438468080 ) ) ;
#144973=EDGE_CURVE ( 'NONE', #180747, #58680, #97603, .T. ) ;
#144977=CARTESIAN_POINT ( 'NONE',  ( -11.07790593930098311, 13.79999999999999893, -0.7000000000000009548 ) ) ;
#144978=AXIS2_PLACEMENT_3D ( 'NONE', #175878, #92510, #41616 ) ;
#144986=FILL_AREA_STYLE_COLOUR ( '', #132326 ) ;
#144988=CARTESIAN_POINT ( 'NONE',  ( 9.601861804102849618, 3.883750271632767870, -7.121441872635297266 ) ) ;
#144997=CARTESIAN_POINT ( 'NONE',  ( -9.508795732819944391, 15.08621132298791423, 7.212928819065541397 ) ) ;
#144999=ORIENTED_EDGE ( 'NONE', *, *, #102377, .F. ) ;
#145006=DIRECTION ( 'NONE',  ( 0.000000000000000000, 0.000000000000000000, -1.000000000000000000 ) ) ;
#145064=UNCERTAINTY_MEASURE_WITH_UNIT (LENGTH_MEASURE( 1.000000000000000082E-05 ), #120361, 'distance_accuracy_value', 'NONE');
#145081=DIRECTION ( 'NONE',  ( 0.000000000000000000, 1.000000000000000000, 0.000000000000000000 ) ) ;
#145083=CARTESIAN_POINT ( 'NONE',  ( 11.48788097203293823, 13.83043054397688287, 3.469500700354829714 ) ) ;
#145088=VECTOR ( 'NONE', #76770, 1000.000000000000000 ) ;
#145111=CARTESIAN_POINT ( 'NONE',  ( 0.000000000000000000, 9.799999999999982947, 0.000000000000000000 ) ) ;
#145115=CARTESIAN_POINT ( 'NONE',  ( -10.33392256004288079, 4.765625372279607141, 5.445010993851796322 ) ) ;
#145119=LINE ( 'NONE', #47606, #123872 ) ;
#145130=CARTESIAN_POINT ( 'NONE',  ( 11.89942855770814312, 12.30000000000000071, 0.6999999999999992895 ) ) ;
#145158=ADVANCED_FACE ( 'NONE', ( #166848 ), #201443, .F. ) ;
#145173=DIRECTION ( 'NONE',  ( 0.000000000000000000, 1.000000000000000000, 0.000000000000000000 ) ) ;
#145216=SURFACE_STYLE_FILL_AREA ( #94318 ) ;
#145231=FACE_OUTER_BOUND ( 'NONE', #25471, .T. ) ;
#145234=EDGE_LOOP ( 'NONE', ( #72412, #181143, #98050, #198912 ) ) ;
#145256=CYLINDRICAL_SURFACE ( 'NONE', #116117, 0.07999999999999998779 ) ;
#145262=DIRECTION ( 'NONE',  ( 0.000000000000000000, 0.000000000000000000, 1.000000000000000000 ) ) ;
#145280=DIRECTION ( 'NONE',  ( 0.000000000000000000, 0.000000000000000000, -1.000000000000000000 ) ) ;
#145287=CARTESIAN_POINT ( 'NONE',  ( -11.33772463945037146, 12.69999999999998153, 3.679999999999999272 ) ) ;
#145300=CARTESIAN_POINT ( 'NONE',  ( 1.500000000000039524, 7.000000000000000000, -10.99818166789401097 ) ) ;
#145302=FACE_OUTER_BOUND ( 'NONE', #26218, .T. ) ;
#145308=ORIENTED_EDGE ( 'NONE', *, *, #150358, .T. ) ;
#145317=ADVANCED_FACE ( 'NONE', ( #149529 ), #84521, .T. ) ;
#145325=CARTESIAN_POINT ( 'NONE',  ( 11.07790593930098311, 13.79999999999999893, 0.6999999999999992895 ) ) ;
#145337=CARTESIAN_POINT ( 'NONE',  ( -11.35573736746270335, 12.48729585586721491, 3.554362808847973731 ) ) ;
#145396=ORIENTED_EDGE ( 'NONE', *, *, #56811, .T. ) ;
#145411=VERTEX_POINT ( 'NONE', #58428 ) ;
#145416=ORIENTED_EDGE ( 'NONE', *, *, #143956, .F. ) ;
#145429=CARTESIAN_POINT ( 'NONE',  ( 11.35573736746281526, 11.11270414413281848, 3.554362808847904009 ) ) ;
#145457=EDGE_CURVE ( 'NONE', #212473, #186645, #174710, .T. ) ;
#145458=( NAMED_UNIT ( * ) SI_UNIT ( $, .STERADIAN. ) SOLID_ANGLE_UNIT ( ) );
#145461=ORIENTED_EDGE ( 'NONE', *, *, #57003, .F. ) ;
#145500=LINE ( 'NONE', #142281, #171830 ) ;
#145508=CARTESIAN_POINT ( 'NONE',  ( 10.72402378181932114, 9.913041843844986545, 5.394155308403613347 ) ) ;
#145526=CARTESIAN_POINT ( 'NONE',  ( 9.268416190114901809, 13.02345702987866893, 8.984174778941602213 ) ) ;
#145539=CARTESIAN_POINT ( 'NONE',  ( -15.75000000000000000, 13.79999999999999893, -3.200000000000001510 ) ) ;
#145542=CIRCLE ( 'NONE', #79773, 0.08000000000000040412 ) ;
#145550=DIRECTION ( 'NONE',  ( 1.000000000000000000, -0.000000000000000000, -0.000000000000000000 ) ) ;
#145552=DIRECTION ( 'NONE',  ( 0.000000000000000000, 1.000000000000000000, 0.000000000000000000 ) ) ;
#145555=CARTESIAN_POINT ( 'NONE',  ( -11.94980361058168938, 10.90000000000000036, -1.100000000000000311 ) ) ;
#145557=B_SPLINE_CURVE_WITH_KNOTS ( 'NONE', 3,
 ( #169628, #139284, #58013, #174990, #205314, #92679 ),
 .UNSPECIFIED., .F., .F.,
 ( 4, 2, 4 ),
 ( 0.001251957608719239451, 0.001565178843344208238, 0.001878400077969176810 ),
 .UNSPECIFIED. ) ;
#145578=CARTESIAN_POINT ( 'NONE',  ( -11.81838370251299075, 7.795688761918559528, -1.817169319662425009 ) ) ;
#145582=CARTESIAN_POINT ( 'NONE',  ( -9.898321827459227507, 16.00000000000624212, 7.924999999990193444 ) ) ;
#145600=AXIS2_PLACEMENT_3D ( 'NONE', #12716, #160057, #126576 ) ;
#145624=CARTESIAN_POINT ( 'NONE',  ( -10.71870444596734195, 5.124999999999999112, -5.395310463726811001 ) ) ;
#145627=CARTESIAN_POINT ( 'NONE',  ( 7.652507619935904337, 14.87749650460459705, -8.827801418404110478 ) ) ;
#145630=CARTESIAN_POINT ( 'NONE',  ( 7.649194982119887243, 14.87821958379617016, 8.830808698579634353 ) ) ;
#145662=CARTESIAN_POINT ( 'NONE',  ( -10.44369227015510404, 5.112964020592957404, 5.232143560358708534 ) ) ;
#145686=ORIENTED_EDGE ( 'NONE', *, *, #146979, .T. ) ;
#145688=CARTESIAN_POINT ( 'NONE',  ( 11.46766370916821742, 8.380394332300772575, 3.382753340440862289 ) ) ;
#145694=CIRCLE ( 'NONE', #169754, 11.92000000000000171 ) ;
#145737=CARTESIAN_POINT ( 'NONE',  ( -11.38917015317169579, 6.531398568769805735, 3.785358204000274007 ) ) ;
#145745=CARTESIAN_POINT ( 'NONE',  ( -11.55921752046871553, 8.211226526406720794, -3.233205798298055544 ) ) ;
#145767=DIRECTION ( 'NONE',  ( -0.000000000000000000, 1.000000000000000000, 0.000000000000000000 ) ) ;
#145775=CARTESIAN_POINT ( 'NONE',  ( -12.65289843835643069, 8.694282390621570045, -1.237672713095353982 ) ) ;
#145841=CARTESIAN_POINT ( 'NONE',  ( -10.89408488338165348, 4.581043481790748828, -4.512313115195546231 ) ) ;
#145857=ORIENTED_EDGE ( 'NONE', *, *, #95954, .F. ) ;
#145861=CARTESIAN_POINT ( 'NONE',  ( -11.84668729035137069, 13.50518580017410386, 1.399999999999998357 ) ) ;
#145899=TOROIDAL_SURFACE ( 'NONE', #52466, 11.92000000000000171, 0.08000000000000000167 ) ;
#145905=DIRECTION ( 'NONE',  ( -0.000000000000000000, -1.000000000000000000, -0.000000000000000000 ) ) ;
#145934=CARTESIAN_POINT ( 'NONE',  ( 11.82996952080117836, 6.822421697701821053, -1.712177087675395226 ) ) ;
#145937=FACE_OUTER_BOUND ( 'NONE', #161747, .T. ) ;
#145943=LINE ( 'NONE', #147000, #56233 ) ;
#145970=CARTESIAN_POINT ( 'NONE',  ( 7.894472390712621745, 15.33652541417121640, -9.039190989196168147 ) ) ;
#145980=STYLED_ITEM ( 'NONE', ( #199356 ), #173474 ) ;
#145987=ADVANCED_FACE ( 'NONE', ( #77865 ), #60549, .T. ) ;
#146009=FACE_OUTER_BOUND ( 'NONE', #184671, .T. ) ;
#146018=CARTESIAN_POINT ( 'NONE',  ( 9.897453898556438645, 12.56651866558563313, 7.888353118025118071 ) ) ;
#146024=STYLED_ITEM ( 'NONE', ( #16334 ), #60799 ) ;
#146030=ORIENTED_EDGE ( 'NONE', *, *, #108972, .F. ) ;
#146042=CARTESIAN_POINT ( 'NONE',  ( -11.92619526913699879, 10.90000000000000036, -1.328859060402686199 ) ) ;
#146048=CARTESIAN_POINT ( 'NONE',  ( -10.43233925736708301, 5.066585305077033752, -5.254699789447807134 ) ) ;
#146069=DIRECTION ( 'NONE',  ( 0.000000000000000000, -7.228014483236694583E-17, 1.000000000000000000 ) ) ;
#146075=CARTESIAN_POINT ( 'NONE',  ( 11.04536101718726293, 11.00590937888831000, -1.100000000000000311 ) ) ;
#146076=DIRECTION ( 'NONE',  ( 0.000000000000000000, 1.000000000000000000, 0.000000000000000000 ) ) ;
#146094=ORIENTED_EDGE ( 'NONE', *, *, #2148, .T. ) ;
#146131=( NAMED_UNIT ( * ) SI_UNIT ( $, .STERADIAN. ) SOLID_ANGLE_UNIT ( ) );
#146166=CARTESIAN_POINT ( 'NONE',  ( 1.677086603292890824E-15, 14.57145996863935800, 11.92238957220009610 ) ) ;
#146170=CARTESIAN_POINT ( 'NONE',  ( 10.98549472050129694, 12.34270202721272014, -1.592011381755358723 ) ) ;
#146188=COLOUR_RGB ( '', 0.09019608, 0.27058824, 0.51372549) ;
#146218=CARTESIAN_POINT ( 'NONE',  ( -0.7616689537640918273, 14.53077577685077415, 12.01010950169515468 ) ) ;
#146227=CARTESIAN_POINT ( 'NONE',  ( 6.928203230280113090, 14.48195938056039900, 9.797958971139216544 ) ) ;
#146245=ORIENTED_EDGE ( 'NONE', *, *, #122928, .T. ) ;
#146255=CIRCLE ( 'NONE', #139281, 0.08000000000000020983 ) ;
#146262=ADVANCED_FACE ( 'NONE', ( #98392 ), #65850, .F. ) ;
#146271=DIRECTION ( 'NONE',  ( -0.000000000000000000, 1.000000000000000000, -0.000000000000000000 ) ) ;
#146272=CIRCLE ( 'NONE', #49452, 10.75000000000000000 ) ;
#146291=ORIENTED_EDGE ( 'NONE', *, *, #144973, .F. ) ;
#146292=DIRECTION ( 'NONE',  ( -0.9982742078614211811, 0.000000000000000000, 0.05872483221476467591 ) ) ;
#146311=CARTESIAN_POINT ( 'NONE',  ( -10.87904062401159422, 6.606773729959338759, 4.960639138626822486 ) ) ;
#146341=MECHANICAL_DESIGN_GEOMETRIC_PRESENTATION_REPRESENTATION('',(#211995),#104889);
#146365=ADVANCED_FACE ( 'NONE', ( #169785 ), #170855, .F. ) ;
#146380=CARTESIAN_POINT ( 'NONE',  ( 11.80251051724185807, 11.29999999999999893, -1.695257889419042874 ) ) ;
#146383=CARTESIAN_POINT ( 'NONE',  ( -11.96533679318038068, 13.75246011186986372, -0.9151144679400586845 ) ) ;
#146394=SURFACE_STYLE_FILL_AREA ( #118190 ) ;
#146395=SURFACE_STYLE_USAGE ( .BOTH. , #64052 ) ;
#146426=CARTESIAN_POINT ( 'NONE',  ( 11.94105721237523277, 12.57259215598211100, 1.187919463087244720 ) ) ;
#146429=CARTESIAN_POINT ( 'NONE',  ( 11.00592642091246454, 11.11020272436436507, -1.444015479094874710 ) ) ;
#146504=PLANE ( 'NONE',  #158798 ) ;
#146515=CARTESIAN_POINT ( 'NONE',  ( 11.97929049433705728, 11.37999999999999901, -0.7046979865771821894 ) ) ;
#146550=LINE ( 'NONE', #197387, #6285 ) ;
#146551=ORIENTED_EDGE ( 'NONE', *, *, #83136, .T. ) ;
#146557=CARTESIAN_POINT ( 'NONE',  ( -11.87828357749949149, 9.796897472595777145, -1.708055325888893972 ) ) ;
#146577=CARTESIAN_POINT ( 'NONE',  ( 9.635860615942547724, 11.95819851461962813, 8.658877209414601595 ) ) ;
#146603=CARTESIAN_POINT ( 'NONE',  ( -11.89942855770813956, 11.29999999999999893, -0.7000000000000009548 ) ) ;
#146629=CARTESIAN_POINT ( 'NONE',  ( -8.752560967064900055, 13.99999998466135231, 9.356054886190362296 ) ) ;
#146672=FILL_AREA_STYLE_COLOUR ( '', #200715 ) ;
#146676=CARTESIAN_POINT ( 'NONE',  ( 8.790672116344218523, 15.72076966503868789, -9.208843758835506321 ) ) ;
#146679=CARTESIAN_POINT ( 'NONE',  ( 8.779893817263781486, 13.51977368570809013, 7.713389242581872196 ) ) ;
#146710=CARTESIAN_POINT ( 'NONE',  ( -12.00295043402534212, 5.507662538472692049, -4.496421502479775789 ) ) ;
#146715=COLOUR_RGB ( '', 0.40784314, 0.44705882, 0.49803922) ;
#146724=DIRECTION ( 'NONE',  ( -0.000000000000000000, 1.000000000000000000, -0.000000000000000000 ) ) ;
#146730=CARTESIAN_POINT ( 'NONE',  ( -9.386185638472888115, 14.48154095986880918, 7.476657895028183454 ) ) ;
#146738=CARTESIAN_POINT ( 'NONE',  ( 11.51992191991745251, 8.397398980953870051, -3.382552691539911116 ) ) ;
#146746=CARTESIAN_POINT ( 'NONE',  ( -10.87339879486171590, 5.131770238416462959, 5.487091846871368084 ) ) ;
#146765=CARTESIAN_POINT ( 'NONE',  ( 10.98546401119367566, 13.75740562920347188, 1.592223900679732518 ) ) ;
#146773=CARTESIAN_POINT ( 'NONE',  ( -15.75000000000000000, 13.39999999999998259, 1.399999999999998579 ) ) ;
#146775=ADVANCED_FACE ( 'NONE', ( #157066 ), #122514, .F. ) ;
#146783=( NAMED_UNIT ( * ) PLANE_ANGLE_UNIT ( ) SI_UNIT ( $, .RADIAN. ) );
#146788=CARTESIAN_POINT ( 'NONE',  ( -11.37863701345828993, 6.568914681733530436, 3.817141491415757759 ) ) ;
#146796=CARTESIAN_POINT ( 'NONE',  ( -11.99998407866956107, 9.073076179820285248, -0.6191218322778160310 ) ) ;
#146842=DIRECTION ( 'NONE',  ( -0.9885327375000381167, 0.000000000000000000, -0.1510067114093955609 ) ) ;
#146845=CARTESIAN_POINT ( 'NONE',  ( 11.48784849554592924, 13.83049527181923111, -3.469614872287849927 ) ) ;
#146865=CARTESIAN_POINT ( 'NONE',  ( 9.534866695232230072, 3.538528462892242654, 7.286654780214751881 ) ) ;
#146881=LINE ( 'NONE', #48307, #78170 ) ;
#146914=CARTESIAN_POINT ( 'NONE',  ( -11.84104725192634966, 13.60983537451416048, 1.443823348526939165 ) ) ;
#146923=ADVANCED_FACE ( 'NONE', ( #107296 ), #171161, .F. ) ;
#146936=UNCERTAINTY_MEASURE_WITH_UNIT (LENGTH_MEASURE( 1.000000000000000082E-05 ), #179971, 'distance_accuracy_value', 'NONE');
#146942=CARTESIAN_POINT ( 'NONE',  ( 11.84668730067608600, 13.39999999999998259, 1.399999999999998579 ) ) ;
#146960=CARTESIAN_POINT ( 'NONE',  ( 11.01135777277261951, 10.09499145469730941, -1.400000000000001243 ) ) ;
#146971=VERTEX_POINT ( 'NONE', #160246 ) ;
#146975=ORIENTED_EDGE ( 'NONE', *, *, #82633, .T. ) ;
#146979=EDGE_CURVE ( 'NONE', #173456, #66261, #64610, .T. ) ;
#146985=ORIENTED_EDGE ( 'NONE', *, *, #152817, .F. ) ;
#146994=DIRECTION ( 'NONE',  ( 0.000000000000000000, 0.000000000000000000, -1.000000000000000000 ) ) ;
#147000=CARTESIAN_POINT ( 'NONE',  ( -15.75000000000000000, 12.69999999999999929, -3.600000000000000977 ) ) ;
#147013=AXIS2_PLACEMENT_3D ( 'NONE', #67130, #137506, #202459 ) ;
#147026=CARTESIAN_POINT ( 'NONE',  ( 9.019512274088125281, 14.59495137906214346, -7.915989402198163383 ) ) ;
#147041=AXIS2_PLACEMENT_3D ( 'NONE', #61513, #63647, #95105 ) ;
#147049=EDGE_CURVE ( 'NONE', #39641, #90767, #168659, .T. ) ;
#147067=CARTESIAN_POINT ( 'NONE',  ( 8.776573235218638303, 13.27486625357122385, -8.183627694784497919 ) ) ;
#147073=ORIENTED_EDGE ( 'NONE', *, *, #112984, .T. ) ;
#147076=CARTESIAN_POINT ( 'NONE',  ( 11.99987416209243385, 8.248970243831804439, 3.607522456176011971 ) ) ;
#147085=CARTESIAN_POINT ( 'NONE',  ( 7.299895746552897968, 14.53718666743123045, -9.471644787737316662 ) ) ;
#147106=CARTESIAN_POINT ( 'NONE',  ( -10.30104275384242740, 4.689840931292195592, -5.506867539468097483 ) ) ;
#147108=CARTESIAN_POINT ( 'NONE',  ( -9.445283354644281815, 15.31899899171029666, 7.300214616139077073 ) ) ;
#147129=( NAMED_UNIT ( * ) PLANE_ANGLE_UNIT ( ) SI_UNIT ( $, .RADIAN. ) );
#147131=B_SPLINE_CURVE_WITH_KNOTS ( 'NONE', 3,
 ( #77840, #110420, #191578, #176423, #28030, #73578 ),
 .UNSPECIFIED., .F., .F.,
 ( 4, 2, 4 ),
 ( 0.000000000000000000, 0.0003172254002810694388, 0.0006344508005621388776 ),
 .UNSPECIFIED. ) ;
#147143=( NAMED_UNIT ( * ) SI_UNIT ( $, .STERADIAN. ) SOLID_ANGLE_UNIT ( ) );
#147148=COLOUR_RGB ( '', 0.66274510, 0.83137255, 0.94901961) ;
#147227=SURFACE_STYLE_USAGE ( .BOTH. , #131028 ) ;
#147272=EDGE_CURVE ( 'NONE', #93151, #118697, #103350, .T. ) ;
#147275=CARTESIAN_POINT ( 'NONE',  ( 8.226144498209521316, 14.18988382969902418, 8.737432991257948700 ) ) ;
#147298=CIRCLE ( 'NONE', #181891, 11.92000000000000171 ) ;
#147299=CARTESIAN_POINT ( 'NONE',  ( 11.88156762547254175, 11.37999991545966516, 1.686557021358693786 ) ) ;
#147303=ADVANCED_FACE ( 'NONE', ( #51841 ), #180758, .T. ) ;
#147330=ORIENTED_EDGE ( 'NONE', *, *, #127684, .F. ) ;
#147409=CARTESIAN_POINT ( 'NONE',  ( -9.604686356149271020, 4.469090097702010489, -7.193747284969076894 ) ) ;
#147421=FACE_OUTER_BOUND ( 'NONE', #80999, .T. ) ;
#147424=MECHANICAL_DESIGN_GEOMETRIC_PRESENTATION_REPRESENTATION('',(#140649),#12566);
#147431=CARTESIAN_POINT ( 'NONE',  ( -11.48767021851170078, 12.26995772536156437, 3.470194894594595070 ) ) ;
#147443=FILL_AREA_STYLE_COLOUR ( '', #114680 ) ;
#147450=CIRCLE ( 'NONE', #161365, 11.18000000000000149 ) ;
#147470=DIRECTION ( 'NONE',  ( -0.000000000000000000, -1.000000000000000000, -0.000000000000000000 ) ) ;
#147536=CARTESIAN_POINT ( 'NONE',  ( 11.55950211276791428, 11.37999999999999901, -3.221476510067115662 ) ) ;
#147537=DIRECTION ( 'NONE',  ( 1.000000000000000000, -0.000000000000000000, -0.000000000000000000 ) ) ;
#147561=( NAMED_UNIT ( * ) SI_UNIT ( $, .STERADIAN. ) SOLID_ANGLE_UNIT ( ) );
#147572=ORIENTED_EDGE ( 'NONE', *, *, #20726, .F. ) ;
#147592=CARTESIAN_POINT ( 'NONE',  ( -9.348561386899502779, 3.999985931113709814, -7.001914024221965960 ) ) ;
#147603=CARTESIAN_POINT ( 'NONE',  ( -11.80251051724186695, 9.799999999999998934, -1.695257889419022890 ) ) ;
#147612=FILL_AREA_STYLE ('',( #111976 ) ) ;
#147623=CARTESIAN_POINT ( 'NONE',  ( 8.431556522904017470, 12.79655328865047892, 8.481395780940484741 ) ) ;
#147625=VERTEX_POINT ( 'NONE', #101645 ) ;
#147648=EDGE_CURVE ( 'NONE', #118044, #12777, #92326, .T. ) ;
#147665=DIRECTION ( 'NONE',  ( 0.000000000000000000, 0.000000000000000000, 1.000000000000000000 ) ) ;
#147671=EDGE_CURVE ( 'NONE', #124, #141526, #154449, .T. ) ;
#147680=CARTESIAN_POINT ( 'NONE',  ( -11.57263578245408908, 7.021380543846468036, 3.181795205153499673 ) ) ;
#147694=ORIENTED_EDGE ( 'NONE', *, *, #3410, .F. ) ;
#147723=CARTESIAN_POINT ( 'NONE',  ( 9.681426354872444406, 13.43812210156014686, -8.165041025796163865 ) ) ;
#147756=CARTESIAN_POINT ( 'NONE',  ( -10.93365108933372198, 4.740440605563193799, -4.433365903526399698 ) ) ;
#147782=ORIENTED_EDGE ( 'NONE', *, *, #111061, .F. ) ;
#147805=AXIS2_PLACEMENT_3D ( 'NONE', #173084, #152546, #120123 ) ;
#147820=DIRECTION ( 'NONE',  ( 0.000000000000000000, -7.228014483236694583E-17, 1.000000000000000000 ) ) ;
#147821=( GEOMETRIC_REPRESENTATION_CONTEXT ( 3 ) GLOBAL_UNCERTAINTY_ASSIGNED_CONTEXT ( ( #85658 ) ) GLOBAL_UNIT_ASSIGNED_CONTEXT ( ( #35766, #151673, #3244 ) ) REPRESENTATION_CONTEXT ( 'NONE', 'WORKASPACE' ) );
#147830=DIRECTION ( 'NONE',  ( 0.000000000000000000, 0.000000000000000000, -1.000000000000000000 ) ) ;
#147835=CARTESIAN_POINT ( 'NONE',  ( -11.67711829288551328, 7.340396131222296283, -2.774295504980774485 ) ) ;
#147877=SURFACE_STYLE_FILL_AREA ( #14645 ) ;
#147880=EDGE_LOOP ( 'NONE', ( #72720, #207015, #188054, #20673 ) ) ;
#147889=ORIENTED_EDGE ( 'NONE', *, *, #158942, .T. ) ;
#147892=CARTESIAN_POINT ( 'NONE',  ( -11.01135777277262306, 12.59376995022298473, 1.399999999999998579 ) ) ;
#147894=CARTESIAN_POINT ( 'NONE',  ( -10.49999999999999822, 13.50840886959780462, -3.600000000000000977 ) ) ;
#147895=DIRECTION ( 'NONE',  ( 0.1700204568168880159, -0.9655305911742139147, 0.1970881066187147312 ) ) ;
#147912=CARTESIAN_POINT ( 'NONE',  ( 9.534369015033190564, 4.462424917548984737, 7.287319680779482667 ) ) ;
#147938=EDGE_CURVE ( 'NONE', #127758, #106229, #212128, .T. ) ;
#147946=VERTEX_POINT ( 'NONE', #154668 ) ;
#147949=CARTESIAN_POINT ( 'NONE',  ( -11.78331023100045627, 12.30000000000000071, -1.800000000000001155 ) ) ;
#147970=ADVANCED_FACE ( 'NONE', ( #169842 ), #103792, .F. ) ;
#147982=CARTESIAN_POINT ( 'NONE',  ( -15.75000000000000000, 11.29999999999999893, -1.800000000000001155 ) ) ;
#148009=CARTESIAN_POINT ( 'NONE',  ( 0.05368761658891522265, 14.48153887695537456, 11.99990993953711893 ) ) ;
#148011=FACE_OUTER_BOUND ( 'NONE', #8482, .T. ) ;
#148025=ORIENTED_EDGE ( 'NONE', *, *, #145457, .F. ) ;
#148036=UNCERTAINTY_MEASURE_WITH_UNIT (LENGTH_MEASURE( 1.000000000000000082E-05 ), #49298, 'distance_accuracy_value', 'NONE');
#148070=DIRECTION ( 'NONE',  ( 0.000000000000000000, -0.000000000000000000, 1.000000000000000000 ) ) ;
#148077=CARTESIAN_POINT ( 'NONE',  ( 11.96209379583854115, 9.772070594057634452, -0.9572398070798752157 ) ) ;
#148078=CARTESIAN_POINT ( 'NONE',  ( -15.75000000000000000, 10.19999999999999929, 1.099999999999996758 ) ) ;
#148109=CARTESIAN_POINT ( 'NONE',  ( -9.813523197712067159, 5.212597839642568509, -6.298667959258508198 ) ) ;
#148135=CARTESIAN_POINT ( 'NONE',  ( 9.300803202052959406, 13.23374025275723120, 6.731078372561743350 ) ) ;
#148138=EDGE_LOOP ( 'NONE', ( #205186, #154913, #105867, #173534, #133677 ) ) ;
#148145=CARTESIAN_POINT ( 'NONE',  ( 8.434158656714652480, 13.95694151194098431, -8.536592743144272077 ) ) ;
#148152=CARTESIAN_POINT ( 'NONE',  ( 0.05083683574733967314, 14.51110989222127223, 11.99422657299097494 ) ) ;
#148161=FILL_AREA_STYLE_COLOUR ( '', #147148 ) ;
#148170=ORIENTED_EDGE ( 'NONE', *, *, #30193, .T. ) ;
#148177=CARTESIAN_POINT ( 'NONE',  ( -9.453429865429503920, 15.47131253150566721, -7.391430728740559175 ) ) ;
#148193=AXIS2_PLACEMENT_3D ( 'NONE', #178550, #45360, #146069 ) ;
#148232=EDGE_CURVE ( 'NONE', #138814, #86850, #56937, .T. ) ;
#148251=DIRECTION ( 'NONE',  ( 1.000000000000000000, -0.000000000000000000, -0.000000000000000000 ) ) ;
#148257=CARTESIAN_POINT ( 'NONE',  ( 11.84668730067608600, 12.69999999999998153, 1.399999999999998579 ) ) ;
#148279=DIRECTION ( 'NONE',  ( 0.000000000000000000, 0.000000000000000000, -1.000000000000000000 ) ) ;
#148333=CARTESIAN_POINT ( 'NONE',  ( 11.48243876534946217, 12.29999999999998295, 3.199999999999997957 ) ) ;
#148339=CARTESIAN_POINT ( 'NONE',  ( 8.359932177502960471, 14.08591219777413528, 8.547035205493129340 ) ) ;
#148341=DIRECTION ( 'NONE',  ( -0.000000000000000000, -1.000000000000000000, -0.000000000000000000 ) ) ;
#148346=AXIS2_PLACEMENT_3D ( 'NONE', #157796, #40849, #153519 ) ;
#148360=ADVANCED_FACE ( 'NONE', ( #127595 ), #12713, .T. ) ;
#148366=( NAMED_UNIT ( * ) PLANE_ANGLE_UNIT ( ) SI_UNIT ( $, .RADIAN. ) );
#148399=DIRECTION ( 'NONE',  ( 0.6250000000000000000, 1.408756634010579545E-16, -0.7806247497997997886 ) ) ;
#148417=DIRECTION ( 'NONE',  ( 1.000000000000000000, -0.000000000000000000, -0.000000000000000000 ) ) ;
#148447=ORIENTED_EDGE ( 'NONE', *, *, #52547, .T. ) ;
#148475=FILL_AREA_STYLE ('',( #68247 ) ) ;
#148476=ORIENTED_EDGE ( 'NONE', *, *, #88601, .F. ) ;
#148541=UNCERTAINTY_MEASURE_WITH_UNIT (LENGTH_MEASURE( 1.000000000000000082E-05 ), #53701, 'distance_accuracy_value', 'NONE');
#148542=CARTESIAN_POINT ( 'NONE',  ( 1.734723475976807094E-15, 14.57349900225068495, 11.91973154060107376 ) ) ;
#148595=CARTESIAN_POINT ( 'NONE',  ( -11.91826848330605770, 12.59270354043021989, -1.400000080589191898 ) ) ;
#148621=CARTESIAN_POINT ( 'NONE',  ( 0.000000000000000000, 0.000000000000000000, 0.000000000000000000 ) ) ;
#148622=DIRECTION ( 'NONE',  ( 0.000000000000000000, 1.000000000000000000, 0.000000000000000000 ) ) ;
#148644=DIRECTION ( 'NONE',  ( 0.9632918427306595976, 0.000000000000000000, 0.2684563758389253985 ) ) ;
#148656=VERTEX_POINT ( 'NONE', #58268 ) ;
#148684=CARTESIAN_POINT ( 'NONE',  ( 8.356287327758902705, 13.10650915898924751, 8.534003350902178653 ) ) ;
#148685=VERTEX_POINT ( 'NONE', #90786 ) ;
#148721=CARTESIAN_POINT ( 'NONE',  ( 11.33772463945036968, 10.09097530385349728, -3.600000000000000977 ) ) ;
#148778=CARTESIAN_POINT ( 'NONE',  ( 7.913958811377831637, 15.96374183207315944, -9.911989391671550464 ) ) ;
#148799=AXIS2_PLACEMENT_3D ( 'NONE', #140273, #203071, #54715 ) ;
#148822=ORIENTED_EDGE ( 'NONE', *, *, #72042, .T. ) ;
#148827=CARTESIAN_POINT ( 'NONE',  ( -9.453965129859655647, 15.47074423828725109, 7.390745084306966639 ) ) ;
#148835=CARTESIAN_POINT ( 'NONE',  ( 9.905912401576173920, 11.51299872167799343, -6.694621976437109545 ) ) ;
#148843=CARTESIAN_POINT ( 'NONE',  ( 7.402824606385355111, 14.51624126053141595, -9.389026765318357448 ) ) ;
#148848=CARTESIAN_POINT ( 'NONE',  ( 11.84668729410392274, 12.59379487675467324, -1.400000000000001688 ) ) ;
#148887=CARTESIAN_POINT ( 'NONE',  ( -11.99137977967679092, 8.009002857758401817, -0.5240188267039559422 ) ) ;
#148896=CARTESIAN_POINT ( 'NONE',  ( -11.78331023100045627, 13.87999999999998302, 1.799999999999999600 ) ) ;
#148912=FILL_AREA_STYLE ('',( #200825 ) ) ;
#148914=EDGE_CURVE ( 'NONE', #118348, #7674, #9514, .T. ) ;
#148942=CARTESIAN_POINT ( 'NONE',  ( -11.92619526248521034, 12.57255386085832605, 1.328859120100916558 ) ) ;
#148946=CARTESIAN_POINT ( 'NONE',  ( 11.41381675112459959, 13.40000000000001101, -3.704697986577260682 ) ) ;
#148953=DIRECTION ( 'NONE',  ( 0.000000000000000000, 0.000000000000000000, 1.000000000000000000 ) ) ;
#148969=ORIENTED_EDGE ( 'NONE', *, *, #5255, .T. ) ;
#149001=CIRCLE ( 'NONE', #173304, 0.08000000000000040412 ) ;
#149029=UNCERTAINTY_MEASURE_WITH_UNIT (LENGTH_MEASURE( 1.000000000000000082E-05 ), #134807, 'distance_accuracy_value', 'NONE');
#149053=CARTESIAN_POINT ( 'NONE',  ( -6.671583288097857611, 16.00000000000178701, -9.747470831326625174 ) ) ;
#149056=CIRCLE ( 'NONE', #17463, 12.00000000000000178 ) ;
#149077=VERTEX_POINT ( 'NONE', #191448 ) ;
#149100=STYLED_ITEM ( 'NONE', ( #61449 ), #72370 ) ;
#149144=ORIENTED_EDGE ( 'NONE', *, *, #153343, .F. ) ;
#149154=CARTESIAN_POINT ( 'NONE',  ( -10.77321989194975416, 5.423924896255240213, -6.620653902763565135 ) ) ;
#149181=EDGE_LOOP ( 'NONE', ( #56484, #115939, #145396, #20038 ) ) ;
#149184=CARTESIAN_POINT ( 'NONE',  ( 9.377738819465895048, 12.64169150452043766, -6.543016420796631039 ) ) ;
#149185=AXIS2_PLACEMENT_3D ( 'NONE', #204023, #42656, #158519 ) ;
#149196=CARTESIAN_POINT ( 'NONE',  ( 8.776573235218652513, 13.27486625357121852, -8.183627694784506801 ) ) ;
#149199=CARTESIAN_POINT ( 'NONE',  ( -11.92619526913699524, 12.57219975838509463, -1.328859060402685976 ) ) ;
#149209=DIRECTION ( 'NONE',  ( -0.9982742078614211811, 0.000000000000000000, -0.05872483221476467591 ) ) ;
#149214=CARTESIAN_POINT ( 'NONE',  ( -11.55950211276791428, 13.88000000000000078, -3.221476510067114329 ) ) ;
#149227=SURFACE_STYLE_USAGE ( .BOTH. , #20280 ) ;
#149243=CARTESIAN_POINT ( 'NONE',  ( 11.06299035296667732, 11.25683704376094418, -0.9087041361035911313 ) ) ;
#149245=CIRCLE ( 'NONE', #59264, 11.09999999999999964 ) ;
#149251=AXIS2_PLACEMENT_3D ( 'NONE', #40510, #71897, #205104 ) ;
#149252=EDGE_LOOP ( 'NONE', ( #212039, #5418, #197123, #47865 ) ) ;
#149271=SURFACE_STYLE_USAGE ( .BOTH. , #99461 ) ;
#149286=UNCERTAINTY_MEASURE_WITH_UNIT (LENGTH_MEASURE( 1.000000000000000082E-05 ), #76691, 'distance_accuracy_value', 'NONE');
#149288=ADVANCED_FACE ( 'NONE', ( #181593 ), #132891, .T. ) ;
#149330=CARTESIAN_POINT ( 'NONE',  ( -11.86145016429273014, 13.40000000000000036, 1.179999999999997051 ) ) ;
#149343=( LENGTH_UNIT ( ) NAMED_UNIT ( * ) SI_UNIT ( .MILLI., .METRE. ) );
#149344=ORIENTED_EDGE ( 'NONE', *, *, #95824, .T. ) ;
#149351=AXIS2_PLACEMENT_3D ( 'NONE', #100364, #101430, #15896 ) ;
#149381=ADVANCED_FACE ( 'NONE', ( #20399 ), #87555, .F. ) ;
#149388=SURFACE_SIDE_STYLE ('',( #34561 ) ) ;
#149396=DIRECTION ( 'NONE',  ( 0.000000000000000000, 0.000000000000000000, -1.000000000000000000 ) ) ;
#149426=EDGE_CURVE ( 'NONE', #87946, #58569, #40951, .T. ) ;
#149452=CARTESIAN_POINT ( 'NONE',  ( -10.24086661081948435, 5.004020940043352184, 7.476643068812830251 ) ) ;
#149463=CARTESIAN_POINT ( 'NONE',  ( -11.35569630219380777, 11.11268439291364452, 3.554478010595060411 ) ) ;
#149465=EDGE_LOOP ( 'NONE', ( #10508, #90591, #147782, #192892 ) ) ;
#149470=AXIS2_PLACEMENT_3D ( 'NONE', #80632, #146724, #66466 ) ;
#149471=ADVANCED_FACE ( 'NONE', ( #187173 ), #88631, .T. ) ;
#149488=ORIENTED_EDGE ( 'NONE', *, *, #2982, .T. ) ;
#149512=CARTESIAN_POINT ( 'NONE',  ( 1.271070482941954571, 8.436788551174016604, -10.93994114196923029 ) ) ;
#149518=CARTESIAN_POINT ( 'NONE',  ( 1.459778984583645340E-15, 18.91999999999999815, -11.92000000000000171 ) ) ;
#149529=FACE_OUTER_BOUND ( 'NONE', #8377, .T. ) ;
#149538=CARTESIAN_POINT ( 'NONE',  ( 11.48788097203293823, 11.33043054397688465, 3.469500700354830158 ) ) ;
#149548=DIRECTION ( 'NONE',  ( 0.000000000000000000, 1.804652791718263484E-16, -1.000000000000000000 ) ) ;
#149549=CARTESIAN_POINT ( 'NONE',  ( -8.800111196542582448, 15.51845924339754390, 8.208664638256164992 ) ) ;
#149566=ADVANCED_FACE ( 'NONE', ( #6272 ), #34858, .T. ) ;
#149628=CARTESIAN_POINT ( 'NONE',  ( -9.367496997601234554, 15.46908218389367029, -7.499999999995462296 ) ) ;
#149630=AXIS2_PLACEMENT_3D ( 'NONE', #43431, #201873, #88162 ) ;
#149652=CARTESIAN_POINT ( 'NONE',  ( -10.91033749632887151, 4.885617943545217834, -4.996452313011736202 ) ) ;
#149659=CARTESIAN_POINT ( 'NONE',  ( -11.86239285000045918, 12.29999999999999716, -1.812080536912752837 ) ) ;
#149685=DIRECTION ( 'NONE',  ( 0.000000000000000000, 0.000000000000000000, 1.000000000000000000 ) ) ;
#149687=ORIENTED_EDGE ( 'NONE', *, *, #62182, .T. ) ;
#149693=DIRECTION ( 'NONE',  ( 0.000000000000000000, 0.000000000000000000, 1.000000000000000000 ) ) ;
#149715=CARTESIAN_POINT ( 'NONE',  ( -11.41176686791169104, 12.34049196513146107, -3.404018756831829418 ) ) ;
#149717=FACE_OUTER_BOUND ( 'NONE', #213623, .T. ) ;
#149722=STYLED_ITEM ( 'NONE', ( #58430 ), #65706 ) ;
#149736=CARTESIAN_POINT ( 'NONE',  ( -11.36822525729066413, 5.406166865499119289, 5.610767994321700591 ) ) ;
#149751=CARTESIAN_POINT ( 'NONE',  ( 12.00693267275518572, 8.237831693621128437, -3.583085096157309302 ) ) ;
#149762=CARTESIAN_POINT ( 'NONE',  ( -1.249999999999964695, 8.500000000000000000, 10.97907099895069294 ) ) ;
#149765=COLOUR_RGB ( '', 0.09019608, 0.27058824, 0.51372549) ;
#149766=DIRECTION ( 'NONE',  ( 0.000000000000000000, -1.000000000000000000, -1.804652791718263484E-16 ) ) ;
#149772=CARTESIAN_POINT ( 'NONE',  ( 11.44789321844504215, 11.29999999999999716, -3.303298730975399167 ) ) ;
#149782=( GEOMETRIC_REPRESENTATION_CONTEXT ( 3 ) GLOBAL_UNCERTAINTY_ASSIGNED_CONTEXT ( ( #131282 ) ) GLOBAL_UNIT_ASSIGNED_CONTEXT ( ( #177501, #127778, #147143 ) ) REPRESENTATION_CONTEXT ( 'NONE', 'WORKASPACE' ) );
#149797=ORIENTED_EDGE ( 'NONE', *, *, #150358, .F. ) ;
#149809=CARTESIAN_POINT ( 'NONE',  ( -11.68285187161687233, 7.296907067810727732, 2.749671221570443080 ) ) ;
#149836=SURFACE_SIDE_STYLE ('',( #50192 ) ) ;
#149857=CARTESIAN_POINT ( 'NONE',  ( 9.645118626927368766, 13.59280469987849216, -8.209452448563446580 ) ) ;
#149864=VERTEX_POINT ( 'NONE', #105 ) ;
#149875=ORIENTED_EDGE ( 'NONE', *, *, #125621, .F. ) ;
#149901=VERTEX_POINT ( 'NONE', #66171 ) ;
#149906=CARTESIAN_POINT ( 'NONE',  ( -9.383881589012478486, 15.40581400629704945, 7.387911201601294664 ) ) ;
#149907=ORIENTED_EDGE ( 'NONE', *, *, #111061, .T. ) ;
#149913=CARTESIAN_POINT ( 'NONE',  ( 10.65566590394000634, 9.862353226835116615, -5.420130399562989254 ) ) ;
#149926=CARTESIAN_POINT ( 'NONE',  ( 11.92619526913699701, 12.69999999999999929, -1.328859060402686199 ) ) ;
#149952=CARTESIAN_POINT ( 'NONE',  ( -9.053429965380070499, 14.55305227869001783, -7.821648902489916289 ) ) ;
#149962=CARTESIAN_POINT ( 'NONE',  ( -11.96212011828583677, 12.27187554950063308, -0.9569185076418453839 ) ) ;
#149964=EDGE_CURVE ( 'NONE', #11599, #8789, #80175, .T. ) ;
#149987=SURFACE_STYLE_FILL_AREA ( #148912 ) ;
#149991=DIRECTION ( 'NONE',  ( -0.000000000000000000, 1.000000000000000000, -0.000000000000000000 ) ) ;
#150046=ORIENTED_EDGE ( 'NONE', *, *, #176483, .F. ) ;
#150055=CARTESIAN_POINT ( 'NONE',  ( -11.86239285000045918, 12.22000000000000064, -1.812080536912752837 ) ) ;
#150077=ADVANCED_FACE ( 'NONE', ( #166920 ), #205024, .T. ) ;
#150079=B_SPLINE_CURVE_WITH_KNOTS ( 'NONE', 3,
 ( #44772, #176885, #211497, #95664, #31711, #78305 ),
 .UNSPECIFIED., .F., .F.,
 ( 4, 2, 4 ),
 ( 0.000000000000000000, 0.0003767011250903909642, 0.0007534022501807819284 ),
 .UNSPECIFIED. ) ;
#150083=ORIENTED_EDGE ( 'NONE', *, *, #201840, .F. ) ;
#150087=DIRECTION ( 'NONE',  ( 0.000000000000000000, -0.000000000000000000, 1.000000000000000000 ) ) ;
#150089=STYLED_ITEM ( 'NONE', ( #208312 ), #185816 ) ;
#150138=CARTESIAN_POINT ( 'NONE',  ( -1.724555757183582561, 15.99999999999538858, -11.68000002332616205 ) ) ;
#150140=CARTESIAN_POINT ( 'NONE',  ( -10.45142907045522129, 5.144535043903895932, -5.216774619840575333 ) ) ;
#150175=DIRECTION ( 'NONE',  ( 0.000000000000000000, 1.000000000000000000, 0.000000000000000000 ) ) ;
#150211=CARTESIAN_POINT ( 'NONE',  ( 11.94105722165070560, 10.07417237917041142, -1.187919369849492757 ) ) ;
#150241=CARTESIAN_POINT ( 'NONE',  ( -10.39336823037077195, 4.932734307774878424, -5.330979603150785451 ) ) ;
#150253=CARTESIAN_POINT ( 'NONE',  ( -11.52114515671133610, 8.081606464056415362, 2.192706985476595261 ) ) ;
#150260=CARTESIAN_POINT ( 'NONE',  ( 11.40211703457567971, 7.516167754840261672, -3.765886988443341021 ) ) ;
#150269=ORIENTED_EDGE ( 'NONE', *, *, #127920, .T. ) ;
#150271=CARTESIAN_POINT ( 'NONE',  ( 9.802633114045661955, 10.59323031708064455, 5.525202073719254869 ) ) ;
#150279=CARTESIAN_POINT ( 'NONE',  ( -11.86145016429273724, 12.59412591486745114, 1.099999999999996980 ) ) ;
#150280=CARTESIAN_POINT ( 'NONE',  ( 8.762672035042523788, 13.53725231859170997, -8.198939407311630845 ) ) ;
#150281=CARTESIAN_POINT ( 'NONE',  ( 11.07790593930098311, 11.29999999999999893, -0.7000000000000009548 ) ) ;
#150289=CIRCLE ( 'NONE', #101734, 0.08000000000000020983 ) ;
#150296=SURFACE_STYLE_FILL_AREA ( #38670 ) ;
#150324=CARTESIAN_POINT ( 'NONE',  ( 11.86145016429272836, 19.00000000000000000, -1.180000000000002158 ) ) ;
#150334=ORIENTED_EDGE ( 'NONE', *, *, #164392, .F. ) ;
#150358=EDGE_CURVE ( 'NONE', #140091, #97721, #157693, .T. ) ;
#150393=CARTESIAN_POINT ( 'NONE',  ( 10.37617649292455724, 9.136187099972529424, -6.038418756994051506 ) ) ;
#150425=CARTESIAN_POINT ( 'NONE',  ( 10.95308175811721085, 12.30000000000000071, -1.800000000000001155 ) ) ;
#150451=AXIS2_PLACEMENT_3D ( 'NONE', #129970, #126768, #112635 ) ;
#150469=CARTESIAN_POINT ( 'NONE',  ( 9.452953409716815969, 4.518459255873298552, -7.393264975473035072 ) ) ;
#150477=CARTESIAN_POINT ( 'NONE',  ( 8.382543407088986598, 14.06748126314016289, 8.587517679487557842 ) ) ;
#150532=CARTESIAN_POINT ( 'NONE',  ( 7.217903723666667659, 15.51194592830137786, 9.588197132884870300 ) ) ;
#150547=ADVANCED_FACE ( 'NONE', ( #922 ), #49706, .F. ) ;
#150555=( GEOMETRIC_REPRESENTATION_CONTEXT ( 3 ) GLOBAL_UNCERTAINTY_ASSIGNED_CONTEXT ( ( #44356 ) ) GLOBAL_UNIT_ASSIGNED_CONTEXT ( ( #30136, #212057, #179590 ) ) REPRESENTATION_CONTEXT ( 'NONE', 'WORKASPACE' ) );
#150560=CARTESIAN_POINT ( 'NONE',  ( -11.13163773270227530, 7.261023013786968683, 4.365999805656710642 ) ) ;
#150590=CARTESIAN_POINT ( 'NONE',  ( 1.250000000000037526, 8.500000000000000000, -10.97907099895068583 ) ) ;
#150613=EDGE_CURVE ( 'NONE', #54318, #125323, #10341, .T. ) ;
#150619=CARTESIAN_POINT ( 'NONE',  ( -11.49978884755372555, 12.35729178837191888, -3.429452816445187402 ) ) ;
#150644=( NAMED_UNIT ( * ) SI_UNIT ( $, .STERADIAN. ) SOLID_ANGLE_UNIT ( ) );
#150677=( NAMED_UNIT ( * ) PLANE_ANGLE_UNIT ( ) SI_UNIT ( $, .RADIAN. ) );
#150680=CARTESIAN_POINT ( 'NONE',  ( -10.30047605039691128, 4.688744718740807116, 5.507884344589919934 ) ) ;
#150681=ORIENTED_EDGE ( 'NONE', *, *, #186335, .T. ) ;
#150697=VERTEX_POINT ( 'NONE', #185580 ) ;
#150709=CARTESIAN_POINT ( 'NONE',  ( -9.490193176475230530, 15.20116513229150534, -7.238303200632643986 ) ) ;
#150732=FACE_OUTER_BOUND ( 'NONE', #71073, .T. ) ;
#150764=CARTESIAN_POINT ( 'NONE',  ( 11.95360554405576359, 11.10444996502598336, -1.059413164304676469 ) ) ;
#150773=DIRECTION ( 'NONE',  ( 0.000000000000000000, 1.000000000000000000, 0.000000000000000000 ) ) ;
#150795=DIRECTION ( 'NONE',  ( 5.578174157656880098E-15, 1.000000000000000000, -7.437565543542506798E-15 ) ) ;
#150811=EDGE_CURVE ( 'NONE', #200044, #27064, #168505, .T. ) ;
#150814=CARTESIAN_POINT ( 'NONE',  ( -11.88671056400589521, 6.998741290788587754, 4.405061004403326486 ) ) ;
#150827=CARTESIAN_POINT ( 'NONE',  ( 9.709990956404908502, 13.29774486163194958, 8.129890332494706939 ) ) ;
#150875=CARTESIAN_POINT ( 'NONE',  ( -11.86145016429273191, 10.90000000000000036, 1.099999999999996758 ) ) ;
#150877=CARTESIAN_POINT ( 'NONE',  ( -9.670366421564544623, 3.035553407718987629, -6.557686755922881972 ) ) ;
#150878=CARTESIAN_POINT ( 'NONE',  ( -10.30047605039691128, 4.688744718740807116, 5.507884344589919934 ) ) ;
#150882=CARTESIAN_POINT ( 'NONE',  ( -11.96447454455668513, 7.947521973683856267, 1.052947412299385377 ) ) ;
#150892=AXIS2_PLACEMENT_3D ( 'NONE', #27164, #192852, #93269 ) ;
#150912=B_SPLINE_CURVE_WITH_KNOTS ( 'NONE', 3,
 ( #98472, #165602, #17191, #82206, #199136, #83266, #116909, #182909, #34525, #166673 ),
 .UNSPECIFIED., .F., .F.,
 ( 4, 2, 2, 2, 4 ),
 ( 7.239403734759171957E-05, 0.0003307887970069800987, 0.0005891835566663685591, 0.0008475783163257569110, 0.001105973075985145371 ),
 .UNSPECIFIED. ) ;
#150928=CARTESIAN_POINT ( 'NONE',  ( 9.200879715223321043, 13.24877694306529641, -9.037004148943696080 ) ) ;
#150934=EDGE_CURVE ( 'NONE', #45474, #48843, #103284, .T. ) ;
#150945=CARTESIAN_POINT ( 'NONE',  ( 11.89321938400721379, 13.76255278360646983, -1.599605898944101323 ) ) ;
#150958=CARTESIAN_POINT ( 'NONE',  ( -11.33772463945036968, 10.19999999999999929, -3.600000000000000977 ) ) ;
#150960=EDGE_CURVE ( 'NONE', #16328, #4563, #135791, .T. ) ;
#150973=DIRECTION ( 'NONE',  ( -0.000000000000000000, 1.000000000000000000, -0.000000000000000000 ) ) ;
#150979=SURFACE_STYLE_FILL_AREA ( #84892 ) ;
#150986=CARTESIAN_POINT ( 'NONE',  ( 11.86145016429272836, 13.40000000000000036, -1.100000000000000533 ) ) ;
#150990=CARTESIAN_POINT ( 'NONE',  ( 7.106142513049811704, 14.54891773411305245, -9.615630241012095070 ) ) ;
#151023=CARTESIAN_POINT ( 'NONE',  ( -8.120144897977780829, 14.55205941280230242, -8.786172316246053882 ) ) ;
#151032=CARTESIAN_POINT ( 'NONE',  ( -11.94651559118242901, 12.44869344121018173, -1.135242698369575587 ) ) ;
#151041=CARTESIAN_POINT ( 'NONE',  ( -11.89942855770813956, 9.719999999999998863, 0.6999999999999992895 ) ) ;
#151045=DIRECTION ( 'NONE',  ( 0.000000000000000000, 0.000000000000000000, -1.000000000000000000 ) ) ;
#151057=EDGE_CURVE ( 'NONE', #74053, #14390, #92628, .T. ) ;
#151067=AXIS2_PLACEMENT_3D ( 'NONE', #22726, #201473, #167938 ) ;
#151091=( BOUNDED_CURVE ( )  B_SPLINE_CURVE ( 3, ( #70546, #123695, #55397, #151844 ),
 .UNSPECIFIED., .F., .T. ) 
 B_SPLINE_CURVE_WITH_KNOTS ( ( 4, 4 ),
 ( 0.001563600248854528623, 0.002072481089630083019 ),
 .UNSPECIFIED. ) 
 CURVE ( )  GEOMETRIC_REPRESENTATION_ITEM ( )  RATIONAL_B_SPLINE_CURVE ( ( 0.9992558763692048762, 0.7599451551847443698, 0.6066669034981619912, 0.5394211213094574076 ) ) 
 REPRESENTATION_ITEM ( '' )  );
#151118=ORIENTED_EDGE ( 'NONE', *, *, #78415, .F. ) ;
#151150=( GEOMETRIC_REPRESENTATION_CONTEXT ( 3 ) GLOBAL_UNCERTAINTY_ASSIGNED_CONTEXT ( ( #206582 ) ) GLOBAL_UNIT_ASSIGNED_CONTEXT ( ( #123017, #89362, #181252 ) ) REPRESENTATION_CONTEXT ( 'NONE', 'WORKASPACE' ) );
#151170=SURFACE_SIDE_STYLE ('',( #34198 ) ) ;
#151177=ADVANCED_FACE ( 'NONE', ( #20931 ), #87027, .F. ) ;
#151202=FACE_OUTER_BOUND ( 'NONE', #175655, .T. ) ;
#151204=CARTESIAN_POINT ( 'NONE',  ( -11.69380381030441107, 8.410673437356566140, -1.083569014401829955 ) ) ;
#151216=ORIENTED_EDGE ( 'NONE', *, *, #85559, .T. ) ;
#151228=VERTEX_POINT ( 'NONE', #105444 ) ;
#151244=( NAMED_UNIT ( * ) PLANE_ANGLE_UNIT ( ) SI_UNIT ( $, .RADIAN. ) );
#151245=CARTESIAN_POINT ( 'NONE',  ( -11.86145016429273724, 10.09412591486744404, 1.099999999999996980 ) ) ;
#151276=CARTESIAN_POINT ( 'NONE',  ( 11.94655611907589154, 9.947990554530955265, 1.134828163062136852 ) ) ;
#151300=EDGE_CURVE ( 'NONE', #198793, #193425, #38744, .T. ) ;
#151306=CARTESIAN_POINT ( 'NONE',  ( -10.36744940472232379, 5.031894517187950555, -7.294791872146300982 ) ) ;
#151307=( LENGTH_UNIT ( ) NAMED_UNIT ( * ) SI_UNIT ( .MILLI., .METRE. ) );
#151323=CARTESIAN_POINT ( 'NONE',  ( 11.08792111388080492, 7.949474773914394277, -4.609825048350510102 ) ) ;
#151334=CARTESIAN_POINT ( 'NONE',  ( -11.33772463945037146, 13.39999999999998259, 3.599999999999999201 ) ) ;
#151335=CARTESIAN_POINT ( 'NONE',  ( 9.805160342514797733, 10.58486009514582449, -5.518090938306281501 ) ) ;
#151347=CARTESIAN_POINT ( 'NONE',  ( 8.455729991919987754, 13.99694205269637948, -8.515310571025079156 ) ) ;
#151400=ORIENTED_EDGE ( 'NONE', *, *, #42056, .T. ) ;
#151455=FILL_AREA_STYLE_COLOUR ( '', #99848 ) ;
#151477=CARTESIAN_POINT ( 'NONE',  ( -9.404907903324922103, 15.51845925627663192, 7.453273793731242769 ) ) ;
#151490=ORIENTED_EDGE ( 'NONE', *, *, #425, .T. ) ;
#151507=VECTOR ( 'NONE', #188340, 1000.000000000000000 ) ;
#151558=ORIENTED_EDGE ( 'NONE', *, *, #169477, .T. ) ;
#151575=EDGE_CURVE ( 'NONE', #140594, #124513, #120456, .T. ) ;
#151595=CARTESIAN_POINT ( 'NONE',  ( 8.277047300324623436, 15.22811773329036278, 8.690146159871410703 ) ) ;
#151607=ORIENTED_EDGE ( 'NONE', *, *, #29138, .F. ) ;
#151640=B_SPLINE_CURVE_WITH_KNOTS ( 'NONE', 3,
 ( #106768, #187947, #42811, #75283, #76344, #172797 ),
 .UNSPECIFIED., .F., .F.,
 ( 4, 2, 4 ),
 ( 0.0006305064395556263506, 0.0009448735008584378857, 0.001259240562161249421 ),
 .UNSPECIFIED. ) ;
#151652=CARTESIAN_POINT ( 'NONE',  ( -11.07790593930098311, 9.799999999999998934, -0.7000000000000009548 ) ) ;
#151673=( NAMED_UNIT ( * ) PLANE_ANGLE_UNIT ( ) SI_UNIT ( $, .RADIAN. ) );
#151681=CARTESIAN_POINT ( 'NONE',  ( 11.41381675112453387, 10.89999999999998259, 3.704697986577180746 ) ) ;
#151684=ORIENTED_EDGE ( 'NONE', *, *, #84119, .T. ) ;
#151690=MECHANICAL_DESIGN_GEOMETRIC_PRESENTATION_REPRESENTATION('',(#2902),#137936);
#151693=CARTESIAN_POINT ( 'NONE',  ( -11.84668730067608600, 13.40000000000000036, -1.400000000000001910 ) ) ;
#151694=DIRECTION ( 'NONE',  ( -0.000000000000000000, -1.000000000000000000, 0.000000000000000000 ) ) ;
#151742=CARTESIAN_POINT ( 'NONE',  ( -9.911963570431085557, 5.384551446482307213, 6.114068938207696036 ) ) ;
#151745=CARTESIAN_POINT ( 'NONE',  ( -1.292128843000315275, 8.373613470998943598, 10.90074592850030832 ) ) ;
#151755=ORIENTED_EDGE ( 'NONE', *, *, #183608, .F. ) ;
#151759=MECHANICAL_DESIGN_GEOMETRIC_PRESENTATION_REPRESENTATION('',(#20298),#203664);
#151761=EDGE_LOOP ( 'NONE', ( #55369, #134010, #35320 ) ) ;
#151773=CARTESIAN_POINT ( 'NONE',  ( -9.472628840046096954, 15.37212083323948519, -7.367007921997711151 ) ) ;
#151777=SURFACE_STYLE_FILL_AREA ( #85689 ) ;
#151792=CARTESIAN_POINT ( 'NONE',  ( -10.61355984101064642, 4.139919643648435787, -5.602303138431320662 ) ) ;
#151795=DIRECTION ( 'NONE',  ( 1.000000000000000000, -0.000000000000000000, -0.000000000000000000 ) ) ;
#151802=EDGE_CURVE ( 'NONE', #91840, #21255, #2571, .T. ) ;
#151828=ORIENTED_EDGE ( 'NONE', *, *, #19138, .F. ) ;
#151844=CARTESIAN_POINT ( 'NONE',  ( 1.734723475976806897E-15, 14.57308041853048408, 11.91973154060107376 ) ) ;
#151855=CARTESIAN_POINT ( 'NONE',  ( -11.44789321844504215, 12.30000000000000249, -3.303298730975397834 ) ) ;
#151860=ORIENTED_EDGE ( 'NONE', *, *, #147272, .T. ) ;
#151876=CARTESIAN_POINT ( 'NONE',  ( -10.50659947519749693, 5.359800460605414152, -5.105385958519358169 ) ) ;
#151879=EDGE_CURVE ( 'NONE', #210693, #129573, #168646, .T. ) ;
#151886=EDGE_CURVE ( 'NONE', #55386, #173258, #213624, .T. ) ;
#151888=CARTESIAN_POINT ( 'NONE',  ( 10.32570460010716396, 11.37497670666806826, 7.285500311179339938 ) ) ;
#151900=CARTESIAN_POINT ( 'NONE',  ( 11.96209379583854115, 12.27207059405763445, -0.9572398070798752157 ) ) ;
#151939=CARTESIAN_POINT ( 'NONE',  ( -11.68361888283353522, 7.298829597232358246, -2.746533259346354505 ) ) ;
#151966=PRESENTATION_STYLE_ASSIGNMENT (( #38210 ) ) ;
#151984=CARTESIAN_POINT ( 'NONE',  ( 7.596942422597253497, 13.84883568004298127, -8.824041907131851659 ) ) ;
#152018=ADVANCED_FACE ( 'NONE', ( #43414 ), #94304, .T. ) ;
#152020=CARTESIAN_POINT ( 'NONE',  ( 7.465383582577691968, 15.41927370284943244, -9.344668898791677947 ) ) ;
#152035=CARTESIAN_POINT ( 'NONE',  ( -9.434499673548478071, 15.42021604052381711, 7.415633384624290336 ) ) ;
#152050=CARTESIAN_POINT ( 'NONE',  ( 7.691668836200880044, 14.45522512263782389, -9.156333440833073212 ) ) ;
#152056=FACE_OUTER_BOUND ( 'NONE', #80808, .T. ) ;
#152081=DIRECTION ( 'NONE',  ( -0.7806247498001170904, 9.887923813067782263E-13, -0.6249999999996038724 ) ) ;
#152099=CARTESIAN_POINT ( 'NONE',  ( -11.76226697576122504, 8.565577005366957763, 2.393665422351130001 ) ) ;
#152102=FACE_OUTER_BOUND ( 'NONE', #82760, .T. ) ;
#152115=FILL_AREA_STYLE_COLOUR ( '', #35131 ) ;
#152119=VERTEX_POINT ( 'NONE', #196052 ) ;
#152135=ORIENTED_EDGE ( 'NONE', *, *, #210187, .T. ) ;
#152193=FACE_OUTER_BOUND ( 'NONE', #122113, .T. ) ;
#152239=CARTESIAN_POINT ( 'NONE',  ( -11.84668730067608600, 12.69999999999998153, 1.319999999999998286 ) ) ;
#152258=CARTESIAN_POINT ( 'NONE',  ( -1.724555757181114535, 13.99999999999846167, -11.68000002332616205 ) ) ;
#152260=CARTESIAN_POINT ( 'NONE',  ( -9.979823206198361163, 5.589814398814587193, -5.978750339097102184 ) ) ;
#152271=( NAMED_UNIT ( * ) PLANE_ANGLE_UNIT ( ) SI_UNIT ( $, .RADIAN. ) );
#152281=EDGE_CURVE ( 'NONE', #61789, #90767, #146550, .T. ) ;
#152302=SURFACE_STYLE_FILL_AREA ( #20144 ) ;
#152364=CARTESIAN_POINT ( 'NONE',  ( -10.89408488338165348, 4.581043481790748828, -4.512313115195546231 ) ) ;
#152380=CARTESIAN_POINT ( 'NONE',  ( 11.53637437042702807, 7.311055218951850065, -3.335631568537873459 ) ) ;
#152392=CARTESIAN_POINT ( 'NONE',  ( -11.86145016429273191, 10.90000000000000036, -1.180000000000002158 ) ) ;
#152393=CARTESIAN_POINT ( 'NONE',  ( 10.15156572269492052, 13.57203269338523022, 7.275605886047803672 ) ) ;
#152405=CARTESIAN_POINT ( 'NONE',  ( -5.969164047770019188, 15.44727374689618138, -10.36856719086336298 ) ) ;
#152410=DIRECTION ( 'NONE',  ( 1.000000000000000000, -5.578174157656880887E-15, 1.224646799146938316E-16 ) ) ;
#152451=DIRECTION ( 'NONE',  ( 0.000000000000000000, -7.254698431490450587E-17, 1.000000000000000000 ) ) ;
#152466=DIRECTION ( 'NONE',  ( 1.000000000000000000, -0.000000000000000000, -0.000000000000000000 ) ) ;
#152468=VERTEX_POINT ( 'NONE', #168103 ) ;
#152497=CARTESIAN_POINT ( 'NONE',  ( -11.94105721237523099, 10.19999999999999929, 1.187919463087245386 ) ) ;
#152504=ORIENTED_EDGE ( 'NONE', *, *, #129415, .T. ) ;
#152514=CARTESIAN_POINT ( 'NONE',  ( -15.75000000000000000, 10.89999999999998259, 1.399999999999998579 ) ) ;
#152546=DIRECTION ( 'NONE',  ( 1.000000000000000000, -0.000000000000000000, -0.000000000000000000 ) ) ;
#152580=CARTESIAN_POINT ( 'NONE',  ( 9.648753856163393650, 3.729559674063779084, -7.135166539715068978 ) ) ;
#152645=FACE_OUTER_BOUND ( 'NONE', #117004, .T. ) ;
#152646=CARTESIAN_POINT ( 'NONE',  ( -10.20579153398542616, 5.000000000000003553, 7.525503907114123869 ) ) ;
#152696=CARTESIAN_POINT ( 'NONE',  ( 10.62873463776380056, 12.29999999999998295, 3.199999999999997957 ) ) ;
#152730=CARTESIAN_POINT ( 'NONE',  ( -11.44779964734733113, 12.60189529870398850, -3.599999963171534478 ) ) ;
#152757=DIRECTION ( 'NONE',  ( 0.8164965809277295872, 1.445884258466820787E-16, -0.5773502691896208461 ) ) ;
#152764=DIRECTION ( 'NONE',  ( 0.000000000000000000, 0.000000000000000000, 1.000000000000000000 ) ) ;
#152783=( NAMED_UNIT ( * ) PLANE_ANGLE_UNIT ( ) SI_UNIT ( $, .RADIAN. ) );
#152792=CARTESIAN_POINT ( 'NONE',  ( 0.08000000000000194456, 19.00000000000000000, 11.91973154060107376 ) ) ;
#152793=CARTESIAN_POINT ( 'NONE',  ( -10.40865662669954084, 4.028931174475638421, 7.242212795919873436 ) ) ;
#152794=ORIENTED_EDGE ( 'NONE', *, *, #87773, .T. ) ;
#152796=UNCERTAINTY_MEASURE_WITH_UNIT (LENGTH_MEASURE( 1.000000000000000082E-05 ), #142440, 'distance_accuracy_value', 'NONE');
#152797=DIRECTION ( 'NONE',  ( -0.000000000000000000, -1.000000000000000000, -0.000000000000000000 ) ) ;
#152801=ORIENTED_EDGE ( 'NONE', *, *, #151575, .T. ) ;
#152817=EDGE_CURVE ( 'NONE', #210028, #96576, #154904, .T. ) ;
#152825=CARTESIAN_POINT ( 'NONE',  ( -9.497949338967845989, 14.58023493191535813, -7.334250927369855511 ) ) ;
#152826=CARTESIAN_POINT ( 'NONE',  ( 11.33772463945037146, 10.19999999999998153, 3.679999999999999272 ) ) ;
#152830=PRESENTATION_STYLE_ASSIGNMENT (( #20671 ) ) ;
#152835=CARTESIAN_POINT ( 'NONE',  ( 11.97929049433705373, 9.719999999999998863, 0.7046979865771783036 ) ) ;
#152840=ADVANCED_FACE ( 'NONE', ( #72717 ), #25362, .T. ) ;
#152846=EDGE_LOOP ( 'NONE', ( #95408, #43000, #114382, #212105 ) ) ;
#152849=CARTESIAN_POINT ( 'NONE',  ( -10.72915461426146244, 4.504162602840288798, -5.276318705760902894 ) ) ;
#152876=CARTESIAN_POINT ( 'NONE',  ( -5.580151458600902004, 15.44693024363194134, -10.58312568620482708 ) ) ;
#152879=EDGE_LOOP ( 'NONE', ( #190360, #104438, #58057, #129861 ) ) ;
#152896=SURFACE_SIDE_STYLE ('',( #86832 ) ) ;
#152903=ORIENTED_EDGE ( 'NONE', *, *, #21155, .F. ) ;
#152913=VERTEX_POINT ( 'NONE', #211240 ) ;
#152928=CARTESIAN_POINT ( 'NONE',  ( -10.94023239993386554, 4.766145680744502400, 4.420001064107922595 ) ) ;
#152932=B_SPLINE_CURVE_WITH_KNOTS ( 'NONE', 3,
 ( #209811, #93978, #113471, #91847, #43097, #160019, #128673, #125468, #177340, #95037, #141679, #179476, #207692, #11618, #127613, #59311, #191430, #211945, #92909, #193578, #109211, #145934, #143814, #175222, #13750, #47356, #158955, #26807, #63581, #61446, #10550, #157904, #111336, #46284, #9498, #195721, #76624, #129738, #96107, #75570 ),
 .UNSPECIFIED., .F., .F.,
 ( 4, 2, 2, 2, 2, 2, 2, 2, 2, 2, 2, 2, 2, 2, 2, 2, 2, 2, 2, 4 ),
 ( -6.000000000487433838E-08, 0.0003665413137380137175, 0.0007331426274760322829, 0.001466345254952070715, 0.002932750509904150180, 0.005865561019808307811, 0.007331966274760386842, 0.008798371529712465874, 0.01026477678466454491, 0.01173118203961662567, 0.01319758729456870470, 0.01393078992204474335, 0.01466399254952078374, 0.01613039780447286450, 0.01759680305942494180, 0.02052961356932909293, 0.02199601882428117369, 0.02272922145175720887, 0.02309582276549522820, 0.02346242407923325446 ),
 .UNSPECIFIED. ) ;
#152942=CARTESIAN_POINT ( 'NONE',  ( 12.13020669054560408, 8.043700598764450760, -3.170917236059372257 ) ) ;
#152951=CARTESIAN_POINT ( 'NONE',  ( -10.50000000000000000, 13.39999999999998259, 3.599999999999999201 ) ) ;
#152961=( GEOMETRIC_REPRESENTATION_CONTEXT ( 3 ) GLOBAL_UNCERTAINTY_ASSIGNED_CONTEXT ( ( #203084 ) ) GLOBAL_UNIT_ASSIGNED_CONTEXT ( ( #160485, #80298, #30497 ) ) REPRESENTATION_CONTEXT ( 'NONE', 'WORKASPACE' ) );
#152995=DIRECTION ( 'NONE',  ( -0.000000000000000000, -1.000000000000000000, -0.000000000000000000 ) ) ;
#152998=FILL_AREA_STYLE_COLOUR ( '', #183528 ) ;
#153062=ORIENTED_EDGE ( 'NONE', *, *, #82220, .F. ) ;
#153094=CARTESIAN_POINT ( 'NONE',  ( 8.856876352573948452, 14.66742331072540040, 8.031069393654634681 ) ) ;
#153095=CARTESIAN_POINT ( 'NONE',  ( -9.421119845716953378, 15.43474195405156912, 7.432612891326888516 ) ) ;
#153099=DIRECTION ( 'NONE',  ( 1.000000000000000000, -0.000000000000000000, -0.000000000000000000 ) ) ;
#153117=AXIS2_PLACEMENT_3D ( 'NONE', #206362, #71007, #119858 ) ;
#153147=CARTESIAN_POINT ( 'NONE',  ( -11.92619526913699879, 12.69999999999998153, 1.328859060402684644 ) ) ;
#153148=CARTESIAN_POINT ( 'NONE',  ( 7.032126278729658786, 15.00000000000000000, -9.944928355699694578 ) ) ;
#153149=CARTESIAN_POINT ( 'NONE',  ( -11.88237951145550575, 11.25680652621284494, 0.9087114598430686696 ) ) ;
#153159=CARTESIAN_POINT ( 'NONE',  ( -11.08179121629665786, 7.064944825185786037, 4.608651903429358043 ) ) ;
#153162=PRESENTATION_STYLE_ASSIGNMENT (( #198688 ) ) ;
#153168=CARTESIAN_POINT ( 'NONE',  ( -10.50000000000000000, 10.90000000000000036, -3.600000000000002309 ) ) ;
#153179=ORIENTED_EDGE ( 'NONE', *, *, #108300, .T. ) ;
#153247=AXIS2_PLACEMENT_3D ( 'NONE', #42116, #90862, #174253 ) ;
#153265=ORIENTED_EDGE ( 'NONE', *, *, #190444, .T. ) ;
#153271=FACE_OUTER_BOUND ( 'NONE', #102508, .T. ) ;
#153280=( NAMED_UNIT ( * ) PLANE_ANGLE_UNIT ( ) SI_UNIT ( $, .RADIAN. ) );
#153287=FACE_OUTER_BOUND ( 'NONE', #5704, .T. ) ;
#153294=UNCERTAINTY_MEASURE_WITH_UNIT (LENGTH_MEASURE( 1.000000000000000082E-05 ), #105235, 'distance_accuracy_value', 'NONE');
#153299=DIRECTION ( 'NONE',  ( 0.000000000000000000, -1.000000000000000000, 0.000000000000000000 ) ) ;
#153308=EDGE_CURVE ( 'NONE', #121817, #47282, #186112, .T. ) ;
#153321=CARTESIAN_POINT ( 'NONE',  ( -9.898321827453750998, 15.00000000001253753, -7.924999999985899990 ) ) ;
#153323=CARTESIAN_POINT ( 'NONE',  ( -11.41048919578708443, 9.369870944694024928, -1.242167297096143264 ) ) ;
#153336=ORIENTED_EDGE ( 'NONE', *, *, #202203, .T. ) ;
#153343=EDGE_CURVE ( 'NONE', #121123, #91407, #2098, .T. ) ;
#153404=B_SPLINE_CURVE_WITH_KNOTS ( 'NONE', 3,
 ( #61121, #178085, #92589, #14484, #93647, #95784 ),
 .UNSPECIFIED., .F., .F.,
 ( 4, 2, 4 ),
 ( 0.000000000000000000, 0.5000000000000000000, 1.000000000000000000 ),
 .UNSPECIFIED. ) ;
#153428=EDGE_LOOP ( 'NONE', ( #137849, #2786, #23010, #203139, #33197 ) ) ;
#153436=CARTESIAN_POINT ( 'NONE',  ( -10.43233925736708301, 5.066585305077033752, -5.254699789447807134 ) ) ;
#153437=CYLINDRICAL_SURFACE ( 'NONE', #131773, 0.3999999999999997446 ) ;
#153452=CARTESIAN_POINT ( 'NONE',  ( 11.91937595155575735, 6.691077280819706097, 0.9935125740681040041 ) ) ;
#153474=CARTESIAN_POINT ( 'NONE',  ( -4.778160426688590867, 15.44696632703637995, -10.96857316220853029 ) ) ;
#153480=CARTESIAN_POINT ( 'NONE',  ( 10.51582573219069694, 9.987091415217268064, 3.554376768052132540 ) ) ;
#153482=MECHANICAL_DESIGN_GEOMETRIC_PRESENTATION_REPRESENTATION('',(#80818),#136330);
#153496=EDGE_CURVE ( 'NONE', #118849, #61426, #9702, .T. ) ;
#153499=ORIENTED_EDGE ( 'NONE', *, *, #74564, .T. ) ;
#153506=FACE_OUTER_BOUND ( 'NONE', #193418, .T. ) ;
#153519=DIRECTION ( 'NONE',  ( 0.000000000000000000, 0.000000000000000000, -1.000000000000000000 ) ) ;
#153523=DIRECTION ( 'NONE',  ( -0.000000000000000000, 1.000000000000000000, 9.023263958591317418E-17 ) ) ;
#153548=FILL_AREA_STYLE_COLOUR ( '', #40671 ) ;
#153593=AXIS2_PLACEMENT_3D ( 'NONE', #214030, #84062, #86199 ) ;
#153604=EDGE_CURVE ( 'NONE', #115034, #79990, #197130, .T. ) ;
#153606=CARTESIAN_POINT ( 'NONE',  ( -11.89197415570408900, 13.80000000000000071, -0.8055989572471861093 ) ) ;
#153614=FACE_OUTER_BOUND ( 'NONE', #107014, .T. ) ;
#153618=ORIENTED_EDGE ( 'NONE', *, *, #95972, .T. ) ;
#153635=( NAMED_UNIT ( * ) SI_UNIT ( $, .STERADIAN. ) SOLID_ANGLE_UNIT ( ) );
#153653=B_SPLINE_CURVE_WITH_KNOTS ( 'NONE', 3,
 ( #55494, #105335, #70644, #156213, #200646, #171372, #22965 ),
 .UNSPECIFIED., .F., .F.,
 ( 4, 3, 4 ),
 ( 2.452946696069607193E-07, 0.0004046562657335365035, 0.0006364688305826707347 ),
 .UNSPECIFIED. ) ;
#153669=CARTESIAN_POINT ( 'NONE',  ( -15.75000000000000000, 12.30000000000000071, 0.6999999999999992895 ) ) ;
#153717=CARTESIAN_POINT ( 'NONE',  ( 11.87815913191693618, 13.80307820631413307, 1.708869976696506754 ) ) ;
#153722=CARTESIAN_POINT ( 'NONE',  ( -11.97185388258315086, 13.87999990720392596, 0.8311143155443557751 ) ) ;
#153731=EDGE_LOOP ( 'NONE', ( #151755, #86206, #51044, #120568 ) ) ;
#153745=SPHERICAL_SURFACE ( 'NONE', #147013, 0.5000000000000001110 ) ;
#153760=FACE_BOUND ( 'NONE', #108571, .T. ) ;
#153761=( NAMED_UNIT ( * ) SI_UNIT ( $, .STERADIAN. ) SOLID_ANGLE_UNIT ( ) );
#153763=AXIS2_PLACEMENT_3D ( 'NONE', #128020, #161504, #145280 ) ;
#153828=ORIENTED_EDGE ( 'NONE', *, *, #185659, .T. ) ;
#153869=CARTESIAN_POINT ( 'NONE',  ( -10.68898853036274055, 3.992937990999307907, 4.901699750972148273 ) ) ;
#153873=EDGE_CURVE ( 'NONE', #177822, #33058, #31453, .T. ) ;
#153883=ORIENTED_EDGE ( 'NONE', *, *, #51382, .F. ) ;
#153884=FILL_AREA_STYLE_COLOUR ( '', #169815 ) ;
#153898=CARTESIAN_POINT ( 'NONE',  ( -9.508835372382730355, 15.10147904770789573, -7.212874380515887474 ) ) ;
#153919=CARTESIAN_POINT ( 'NONE',  ( -5.540653355401692792, 14.53096581237021567, 10.65389762808975149 ) ) ;
#153973=CYLINDRICAL_SURFACE ( 'NONE', #66495, 0.3999999999999997446 ) ;
#153985=DIRECTION ( 'NONE',  ( -3.491481338843133750E-15, -0.000000000000000000, -1.000000000000000000 ) ) ;
#154002=CARTESIAN_POINT ( 'NONE',  ( -15.75000000000000000, 10.19999999999998153, 3.199999999999997957 ) ) ;
#154003=CARTESIAN_POINT ( 'NONE',  ( -10.94029418865078362, 4.766281873824294024, -4.419956640179717233 ) ) ;
#154004=MECHANICAL_DESIGN_GEOMETRIC_PRESENTATION_REPRESENTATION('',(#192010),#88274);
#154005=( NAMED_UNIT ( * ) SI_UNIT ( $, .STERADIAN. ) SOLID_ANGLE_UNIT ( ) );
#154009=MECHANICAL_DESIGN_GEOMETRIC_PRESENTATION_REPRESENTATION('',(#140119),#192020);
#154010=EDGE_CURVE ( 'NONE', #79400, #154255, #200311, .T. ) ;
#154016=CARTESIAN_POINT ( 'NONE',  ( 11.57754556164262993, 8.947311289249686439, -4.715264992745044736 ) ) ;
#154031=FACE_OUTER_BOUND ( 'NONE', #54119, .T. ) ;
#154069=CARTESIAN_POINT ( 'NONE',  ( 11.07790593930098311, 12.30000000000000071, 0.6999999999999992895 ) ) ;
#154073=CARTESIAN_POINT ( 'NONE',  ( 9.367496997597598352, 4.518459255872631530, -7.500000000000005329 ) ) ;
#154122=VERTEX_POINT ( 'NONE', #57034 ) ;
#154139=CIRCLE ( 'NONE', #8791, 11.95586206894144965 ) ;
#154146=B_SPLINE_CURVE_WITH_KNOTS ( 'NONE', 3,
 ( #24803, #89844, #36790, #7481, #119180, #168933 ),
 .UNSPECIFIED., .F., .F.,
 ( 4, 2, 4 ),
 ( 0.000000000000000000, 0.0003779448103413555527, 0.0007558896206827111055 ),
 .UNSPECIFIED. ) ;
#154250=CARTESIAN_POINT ( 'NONE',  ( 11.04536101718726293, 13.40000000000000036, 1.099999999999996758 ) ) ;
#154255=VERTEX_POINT ( 'NONE', #190215 ) ;
#154267=FACE_OUTER_BOUND ( 'NONE', #81773, .T. ) ;
#154322=FACE_OUTER_BOUND ( 'NONE', #6385, .T. ) ;
#154361=FACE_OUTER_BOUND ( 'NONE', #80226, .T. ) ;
#154371=DIRECTION ( 'NONE',  ( -0.1827044046890596851, 0.9634447193773951756, -0.1959422700976716503 ) ) ;
#154375=LINE ( 'NONE', #185779, #114980 ) ;
#154383=CARTESIAN_POINT ( 'NONE',  ( 11.97929049433705728, 9.719999999999998863, 0.7046979865771804130 ) ) ;
#154396=CARTESIAN_POINT ( 'NONE',  ( -11.31088518949709965, 5.182344123437907513, 5.726584094856639773 ) ) ;
#154403=STYLED_ITEM ( 'NONE', ( #199875 ), #196354 ) ;
#154426=ORIENTED_EDGE ( 'NONE', *, *, #12829, .F. ) ;
#154446=EDGE_CURVE ( 'NONE', #14213, #176917, #105821, .T. ) ;
#154449=CIRCLE ( 'NONE', #9255, 0.08000000000000020983 ) ;
#154453=ADVANCED_FACE ( 'NONE', ( #193430 ), #129232, .T. ) ;
#154470=ORIENTED_EDGE ( 'NONE', *, *, #151886, .F. ) ;
#154493=ORIENTED_EDGE ( 'NONE', *, *, #82737, .T. ) ;
#154506=CARTESIAN_POINT ( 'NONE',  ( -10.49139461985735977, 3.038394114823554482, -7.128631142076787164 ) ) ;
#154515=CARTESIAN_POINT ( 'NONE',  ( -10.52284959769361805, 5.420271152154175986, 5.071911021504272199 ) ) ;
#154522=DIRECTION ( 'NONE',  ( 0.000000000000000000, 1.000000000000000000, 0.000000000000000000 ) ) ;
#154526=ORIENTED_EDGE ( 'NONE', *, *, #79201, .F. ) ;
#154531=ORIENTED_EDGE ( 'NONE', *, *, #14021, .T. ) ;
#154536=EDGE_CURVE ( 'NONE', #138322, #147946, #89349, .T. ) ;
#154543=CARTESIAN_POINT ( 'NONE',  ( -3.090297434914522690, 15.44821197608033536, -11.55767568840040127 ) ) ;
#154545=ORIENTED_EDGE ( 'NONE', *, *, #111152, .F. ) ;
#154558=( LENGTH_UNIT ( ) NAMED_UNIT ( * ) SI_UNIT ( .MILLI., .METRE. ) );
#154563=ADVANCED_FACE ( 'NONE', ( #115440 ), #144726, .F. ) ;
#154569=ORIENTED_EDGE ( 'NONE', *, *, #64259, .T. ) ;
#154588=DIRECTION ( 'NONE',  ( 0.000000000000000000, 0.000000000000000000, 1.000000000000000000 ) ) ;
#154592=CARTESIAN_POINT ( 'NONE',  ( -10.55260481140867235, 5.124873218919925755, -7.009574331923702495 ) ) ;
#154593=MECHANICAL_DESIGN_GEOMETRIC_PRESENTATION_REPRESENTATION('',(#16170),#106245);
#154646=ORIENTED_EDGE ( 'NONE', *, *, #88694, .F. ) ;
#154668=CARTESIAN_POINT ( 'NONE',  ( -11.78331023100045627, 12.30000000000000071, -1.800000000000001155 ) ) ;
#154670=ORIENTED_EDGE ( 'NONE', *, *, #193087, .T. ) ;
#154678=FILL_AREA_STYLE ('',( #24656 ) ) ;
#154688=DIRECTION ( 'NONE',  ( 0.000000000000000000, 0.000000000000000000, -1.000000000000000000 ) ) ;
#154690=EDGE_CURVE ( 'NONE', #183276, #195372, #177591, .T. ) ;
#154705=CARTESIAN_POINT ( 'NONE',  ( 6.928203230275524760, 15.51845925587262798, -9.797958971132702644 ) ) ;
#154707=CARTESIAN_POINT ( 'NONE',  ( -11.92619526913699879, 13.40000000000000036, -1.328859060402686199 ) ) ;
#154730=DIRECTION ( 'NONE',  ( -0.5773502691896238437, 0.000000000000000000, -0.8164965809277274778 ) ) ;
#154735=DIRECTION ( 'NONE',  ( 1.000000000000000000, -0.000000000000000000, -0.000000000000000000 ) ) ;
#154772=CARTESIAN_POINT ( 'NONE',  ( 11.41381675112453387, 19.00000000000000000, -3.704697986577182522 ) ) ;
#154788=CARTESIAN_POINT ( 'NONE',  ( -9.587704862635016312, 4.026159954882873926, 6.671158199369250141 ) ) ;
#154810=EDGE_CURVE ( 'NONE', #95488, #11477, #51447, .T. ) ;
#154812=CARTESIAN_POINT ( 'NONE',  ( 9.574755730265700038, 4.231293077548122561, -7.158835739769526363 ) ) ;
#154829=CARTESIAN_POINT ( 'NONE',  ( 11.48243876534946217, 13.79999999999998295, 3.199999999999997957 ) ) ;
#154830=EDGE_CURVE ( 'NONE', #127020, #70402, #68595, .T. ) ;
#154837=CARTESIAN_POINT ( 'NONE',  ( -11.89942855770814134, 13.79999999999999893, 0.6999999999999992895 ) ) ;
#154844=AXIS2_PLACEMENT_3D ( 'NONE', #68777, #167376, #87184 ) ;
#154855=EDGE_CURVE ( 'NONE', #193391, #71097, #19983, .T. ) ;
#154877=EDGE_LOOP ( 'NONE', ( #119174, #88116, #168234, #5476, #16811, #54282, #212825, #67111 ) ) ;
#154890=STYLED_ITEM ( 'NONE', ( #5186 ), #105052 ) ;
#154902=CARTESIAN_POINT ( 'NONE',  ( 11.95069383916873207, 7.566995367135784356, 0.4543839392838792124 ) ) ;
#154904=CIRCLE ( 'NONE', #168805, 0.07999999999999969635 ) ;
#154913=ORIENTED_EDGE ( 'NONE', *, *, #106881, .F. ) ;
#154923=FILL_AREA_STYLE_COLOUR ( '', #29842 ) ;
#154932=CARTESIAN_POINT ( 'NONE',  ( -10.32660017610915837, 5.019824769181640889, 7.354833152352289183 ) ) ;
#154936=UNCERTAINTY_MEASURE_WITH_UNIT (LENGTH_MEASURE( 1.000000000000000082E-05 ), #44739, 'distance_accuracy_value', 'NONE');
#154951=ORIENTED_EDGE ( 'NONE', *, *, #52849, .T. ) ;
#154973=CARTESIAN_POINT ( 'NONE',  ( 11.96533679318037890, 13.75246011186996498, 0.9151144679400620152 ) ) ;
#154997=TOROIDAL_SURFACE ( 'NONE', #168748, 12.17999999982603399, 0.5000000000000008882 ) ;
#155007=ORIENTED_EDGE ( 'NONE', *, *, #50194, .F. ) ;
#155016=DIRECTION ( 'NONE',  ( 1.000000000000000000, -0.000000000000000000, -0.000000000000000000 ) ) ;
#155067=SURFACE_STYLE_FILL_AREA ( #121580 ) ;
#155068=CARTESIAN_POINT ( 'NONE',  ( -11.52114515671133610, 8.081606464056415362, 2.192706985476595261 ) ) ;
#155070=DIRECTION ( 'NONE',  ( -0.9632918427306580433, 0.000000000000000000, 0.2684563758389303945 ) ) ;
#155074=B_SPLINE_CURVE_WITH_KNOTS ( 'NONE', 3,
 ( #189713, #108540, #136718, #171330, #54394, #73839 ),
 .UNSPECIFIED., .F., .F.,
 ( 4, 2, 4 ),
 ( 0.0006305064395556263506, 0.0009448735008584378857, 0.001259240562161249421 ),
 .UNSPECIFIED. ) ;
#155097=EDGE_LOOP ( 'NONE', ( #106486, #61293, #127919, #165854 ) ) ;
#155106=CARTESIAN_POINT ( 'NONE',  ( 11.84668730067608600, 13.39999999999998259, 1.399999999999998579 ) ) ;
#155133=ORIENTED_EDGE ( 'NONE', *, *, #21155, .T. ) ;
#155137=( LENGTH_UNIT ( ) NAMED_UNIT ( * ) SI_UNIT ( .MILLI., .METRE. ) );
#155165=DIRECTION ( 'NONE',  ( 0.000000000000000000, 0.000000000000000000, -1.000000000000000000 ) ) ;
#155180=CARTESIAN_POINT ( 'NONE',  ( 8.939234941184713179, 14.72725019231858390, 8.009301753890152753 ) ) ;
#155181=ORIENTED_EDGE ( 'NONE', *, *, #67497, .F. ) ;
#155189=CARTESIAN_POINT ( 'NONE',  ( 11.01135777277262306, 0.000000000000000000, 1.399999999999998579 ) ) ;
#155225=CARTESIAN_POINT ( 'NONE',  ( -9.569358774149643310, 3.553052365627049625, 7.167287524840453727 ) ) ;
#155238=CARTESIAN_POINT ( 'NONE',  ( -10.71026998871754721, 6.055660674263378951, 4.667787751035539223 ) ) ;
#155240=DIRECTION ( 'NONE',  ( 0.000000000000000000, 0.000000000000000000, -1.000000000000000000 ) ) ;
#155243=CARTESIAN_POINT ( 'NONE',  ( -6.730854013983878836, 14.55213468793103182, -9.890941155911500360 ) ) ;
#155273=ADVANCED_FACE ( 'NONE', ( #157492 ), #90551, .T. ) ;
#155288=CARTESIAN_POINT ( 'NONE',  ( -11.86145016429273014, 12.69999999999999929, 1.099999999999996980 ) ) ;
#155301=AXIS2_PLACEMENT_3D ( 'NONE', #201955, #70897, #38430 ) ;
#155337=ORIENTED_EDGE ( 'NONE', *, *, #58229, .T. ) ;
#155362=CARTESIAN_POINT ( 'NONE',  ( 0.000000000000000000, 19.00000000000000000, -12.00000000000000178 ) ) ;
#155375=DIRECTION ( 'NONE',  ( 0.000000000000000000, 0.000000000000000000, -1.000000000000000000 ) ) ;
#155382=DIRECTION ( 'NONE',  ( 0.000000000000000000, -9.023263958591318651E-17, 1.000000000000000000 ) ) ;
#155407=CARTESIAN_POINT ( 'NONE',  ( -11.35605497252127449, 11.11418145951643943, 3.553547709190206128 ) ) ;
#155418=CARTESIAN_POINT ( 'NONE',  ( 7.416489442564358825, 14.99999999999999467, 9.452688479263381183 ) ) ;
#155425=CARTESIAN_POINT ( 'NONE',  ( 9.153107034568822797, 14.18422307519461789, 6.999546554107224594 ) ) ;
#155432=UNCERTAINTY_MEASURE_WITH_UNIT (LENGTH_MEASURE( 1.000000000000000082E-05 ), #174971, 'distance_accuracy_value', 'NONE');
#155460=CARTESIAN_POINT ( 'NONE',  ( -11.68287950975655676, 8.167437761341201252, 4.460353674290588266 ) ) ;
#155462=EDGE_CURVE ( 'NONE', #48008, #185203, #61040, .T. ) ;
#155498=STYLED_ITEM ( 'NONE', ( #156870 ), #25342 ) ;
#155502=FACE_BOUND ( 'NONE', #30560, .T. ) ;
#155571=CARTESIAN_POINT ( 'NONE',  ( -11.94105721237523099, 10.90000000000000036, -1.187919463087249827 ) ) ;
#155573=CARTESIAN_POINT ( 'NONE',  ( -10.19200560444942560, 4.477620260464512114, -5.707107691925500603 ) ) ;
#155576=CARTESIAN_POINT ( 'NONE',  ( 11.84668730067608600, 10.89999999999998259, 1.399999999999998579 ) ) ;
#155582=CARTESIAN_POINT ( 'NONE',  ( -10.05278092738192619, 5.876216011288541985, -5.831672646394378212 ) ) ;
#155586=VERTEX_POINT ( 'NONE', #212536 ) ;
#155607=CARTESIAN_POINT ( 'NONE',  ( -9.367496997608871112, 15.42330868759649043, 7.413898975919298806 ) ) ;
#155631=EDGE_LOOP ( 'NONE', ( #19692, #172372, #150681, #144464 ) ) ;
#155656=CARTESIAN_POINT ( 'NONE',  ( -11.25372107582773396, 4.972923339538419363, -5.839092030517418763 ) ) ;
#155756=CARTESIAN_POINT ( 'NONE',  ( 11.04536101718726293, 13.40000000000000036, -1.100000000000002087 ) ) ;
#155757=CARTESIAN_POINT ( 'NONE',  ( 11.94105721237523277, 10.90000000000000036, 1.187919463087245386 ) ) ;
#155798=LINE ( 'NONE', #205590, #24462 ) ;
#155828=SURFACE_STYLE_USAGE ( .BOTH. , #27950 ) ;
#155831=CARTESIAN_POINT ( 'NONE',  ( 9.533882724342092274, 4.462909762398312274, 7.287958407156895468 ) ) ;
#155838=CARTESIAN_POINT ( 'NONE',  ( 11.41381675112460847, 13.53016735491475941, -3.704697986577268232 ) ) ;
#155840=CARTESIAN_POINT ( 'NONE',  ( -11.84103413958623818, 9.989955215268501831, 1.443924719788817423 ) ) ;
#155854=CARTESIAN_POINT ( 'NONE',  ( -11.94980361490430099, 13.50332124735869854, 1.099999952233555955 ) ) ;
#155855=AXIS2_PLACEMENT_3D ( 'NONE', #4785, #85010, #148953 ) ;
#155856=CARTESIAN_POINT ( 'NONE',  ( -10.22583553578405358, 2.999999999999999556, 7.498742284419905424 ) ) ;
#155865=ORIENTED_EDGE ( 'NONE', *, *, #210252, .T. ) ;
#155884=CARTESIAN_POINT ( 'NONE',  ( -8.171050021823464959, 15.51987628352802417, -8.834037178151259440 ) ) ;
#155897=SURFACE_SIDE_STYLE ('',( #140748 ) ) ;
#155921=DIRECTION ( 'NONE',  ( 0.000000000000000000, 1.485208455481716443E-16, -1.000000000000000000 ) ) ;
#155925=CARTESIAN_POINT ( 'NONE',  ( -11.95360554405587017, 11.10444996502583237, 1.059413164304700006 ) ) ;
#155928=ORIENTED_EDGE ( 'NONE', *, *, #3914, .T. ) ;
#155954=CARTESIAN_POINT ( 'NONE',  ( -4.353222949258705121, 15.46947200944509682, 11.19154526970763364 ) ) ;
#155969=CARTESIAN_POINT ( 'NONE',  ( 10.80647848125409993, 9.579244470042894477, -5.114164611927699333 ) ) ;
#155970=CARTESIAN_POINT ( 'NONE',  ( -1.423205080756851260, 7.980384757729337863, 10.65537363484302524 ) ) ;
#155991=SURFACE_SIDE_STYLE ('',( #89940 ) ) ;
#155998=CARTESIAN_POINT ( 'NONE',  ( -0.06005734137062879868, 15.49847999378906138, 11.99783618803943241 ) ) ;
#155999=CARTESIAN_POINT ( 'NONE',  ( -9.748179543381699119, 3.057003318903428912, 6.445181705109019887 ) ) ;
#156000=ORIENTED_EDGE ( 'NONE', *, *, #52471, .T. ) ;
#156038=CARTESIAN_POINT ( 'NONE',  ( 11.97297122925952273, 13.79874920673088745, 0.8121202983519189011 ) ) ;
#156042=EDGE_CURVE ( 'NONE', #62806, #173456, #105794, .T. ) ;
#156048=CARTESIAN_POINT ( 'NONE',  ( -9.864361085393147377, 3.580476348100011919, -6.759752543078383802 ) ) ;
#156055=CARTESIAN_POINT ( 'NONE',  ( -11.92619526913699879, 10.89999999999998259, 1.328859060402682868 ) ) ;
#156064=CARTESIAN_POINT ( 'NONE',  ( 11.33772463945036790, 13.40000000000000036, -3.600000000000002309 ) ) ;
#156071=AXIS2_PLACEMENT_3D ( 'NONE', #194838, #164477, #81091 ) ;
#156088=CARTESIAN_POINT ( 'NONE',  ( 0.000000000000000000, 12.30000000000000071, 0.000000000000000000 ) ) ;
#156090=ORIENTED_EDGE ( 'NONE', *, *, #113251, .T. ) ;
#156104=( BOUNDED_SURFACE ( )  B_SPLINE_SURFACE ( 3, 3, ( 
 ( #124089, #141361, #5940, #24333, #206299, #88300, #158637, #207374, #139187, #191108, #72011, #58994, #26485, #123033, #187909, #188984, #172758, #76309 ),
 ( #192176, #55786, #104554, #157580, #190052, #92595, #60059, #57924, #42776, #125150, #142416, #9173, #174906, #121943, #105640, #10234, #208425, #126214 ),
 ( #22184, #106731, #8098, #107814, #23264, #89376, #155425, #74187, #41704, #173839, #25416, #7010, #91521, #73086, #56859, #90441, #156509, #11296 ),
 ( #61128, #144560, #28636, #146679, #63262, #30782, #45970, #44906, #211627, #130477, #79512, #127288, #145630, #43837, #209487, #143490, #14491, #160766 ),
 ( #129424, #114222, #62204, #111014, #195407, #94723, #95791, #212694, #77375, #47037, #193259, #109953, #177019, #12361, #80581, #178092, #113152, #13436 ),
 ( #175963, #179158, #96861, #194328, #27558, #159697, #162909, #64336, #93654, #196468, #48110, #112091, #78440, #210570, #128360, #29710, #161848, #109590 ),
 ( #191807, #23980, #140993, #90083, #208063, #57569, #74885, #157210, #60758, #40257, #123727, #175596, #138832, #106369, #56502, #207001, #7728, #43472 ) ),
 .UNSPECIFIED., .T., .F., .T. ) 
 B_SPLINE_SURFACE_WITH_KNOTS ( ( 4, 3, 4 ),
 ( 4, 2, 2, 2, 2, 2, 2, 2, 4 ),
 ( 0.000000000000000000, 0.5000000000000000000, 1.000000000000000000 ),
 ( 0.7548633226336768365, 0.7573624263556413272, 0.7598615300776057069, 0.7648597375215344663, 0.7748561524093919850, 0.7948489821851072445, 0.8148337662062091757, 0.8248261582167601969, 0.8348185502273111069 ),
 .UNSPECIFIED. ) 
 GEOMETRIC_REPRESENTATION_ITEM ( )  RATIONAL_B_SPLINE_SURFACE ( (
 ( 1.000000000000000000, 1.000000000000000000, 1.000000000000000000, 1.000000000000000000, 1.000000000000000000, 1.000000000000000000, 1.000000000000000000, 1.000000000000000000, 1.000000000000000000, 1.000000000000000000, 1.000000000000000000, 1.000000000000000000, 1.000000000000000000, 1.000000000000000000, 1.000000000000000000, 1.000000000000000000, 1.000000000000000000, 1.000000000000000000),
 ( 0.3333333333333333703, 0.3333333333333333703, 0.3333333333333333703, 0.3333333333333333703, 0.3333333333333333703, 0.3333333333333333703, 0.3333333333333333703, 0.3333333333333333703, 0.3333333333333333703, 0.3333333333333333703, 0.3333333333333333703, 0.3333333333333333703, 0.3333333333333333703, 0.3333333333333333703, 0.3333333333333333703, 0.3333333333333333703, 0.3333333333333333703, 0.3333333333333333703),
 ( 0.3333333333333333703, 0.3333333333333333703, 0.3333333333333333703, 0.3333333333333333703, 0.3333333333333333703, 0.3333333333333333703, 0.3333333333333333703, 0.3333333333333333703, 0.3333333333333333703, 0.3333333333333333703, 0.3333333333333333703, 0.3333333333333333703, 0.3333333333333333703, 0.3333333333333333703, 0.3333333333333333703, 0.3333333333333333703, 0.3333333333333333703, 0.3333333333333333703),
 ( 1.000000000000000000, 1.000000000000000000, 1.000000000000000000, 1.000000000000000000, 1.000000000000000000, 1.000000000000000000, 1.000000000000000000, 1.000000000000000000, 1.000000000000000000, 1.000000000000000000, 1.000000000000000000, 1.000000000000000000, 1.000000000000000000, 1.000000000000000000, 1.000000000000000000, 1.000000000000000000, 1.000000000000000000, 1.000000000000000000),
 ( 0.3333333333333333703, 0.3333333333333333703, 0.3333333333333333703, 0.3333333333333333703, 0.3333333333333333703, 0.3333333333333333703, 0.3333333333333333703, 0.3333333333333333703, 0.3333333333333333703, 0.3333333333333333703, 0.3333333333333333703, 0.3333333333333333703, 0.3333333333333333703, 0.3333333333333333703, 0.3333333333333333703, 0.3333333333333333703, 0.3333333333333333703, 0.3333333333333333703),
 ( 0.3333333333333333703, 0.3333333333333333703, 0.3333333333333333703, 0.3333333333333333703, 0.3333333333333333703, 0.3333333333333333703, 0.3333333333333333703, 0.3333333333333333703, 0.3333333333333333703, 0.3333333333333333703, 0.3333333333333333703, 0.3333333333333333703, 0.3333333333333333703, 0.3333333333333333703, 0.3333333333333333703, 0.3333333333333333703, 0.3333333333333333703, 0.3333333333333333703),
 ( 1.000000000000000000, 1.000000000000000000, 1.000000000000000000, 1.000000000000000000, 1.000000000000000000, 1.000000000000000000, 1.000000000000000000, 1.000000000000000000, 1.000000000000000000, 1.000000000000000000, 1.000000000000000000, 1.000000000000000000, 1.000000000000000000, 1.000000000000000000, 1.000000000000000000, 1.000000000000000000, 1.000000000000000000, 1.000000000000000000) ) ) 
 REPRESENTATION_ITEM ( '' )  SURFACE ( )  );
#156128=CARTESIAN_POINT ( 'NONE',  ( -11.78331023100045627, 13.79999999999999893, -1.800000000000001155 ) ) ;
#156143=CARTESIAN_POINT ( 'NONE',  ( -10.78237064342727791, 6.270194388237658956, -4.501389708959286473 ) ) ;
#156144=AXIS2_PLACEMENT_3D ( 'NONE', #69729, #188838, #139043 ) ;
#156146=CARTESIAN_POINT ( 'NONE',  ( -11.48243876534946217, 9.799999999999982947, 3.199999999999997957 ) ) ;
#156158=FACE_OUTER_BOUND ( 'NONE', #199234, .T. ) ;
#156167=FACE_OUTER_BOUND ( 'NONE', #41839, .T. ) ;
#156205=VERTEX_POINT ( 'NONE', #8243 ) ;
#156208=ORIENTED_EDGE ( 'NONE', *, *, #62427, .F. ) ;
#156213=CARTESIAN_POINT ( 'NONE',  ( -1.313174662617493382, 8.310476012147637093, -10.86148356754322819 ) ) ;
#156217=CARTESIAN_POINT ( 'NONE',  ( 0.08053691275167890185, 14.48153890507870223, 11.99972973886013961 ) ) ;
#156218=SURFACE_STYLE_USAGE ( .BOTH. , #204921 ) ;
#156242=DIRECTION ( 'NONE',  ( 1.000000000000000000, -0.000000000000000000, -0.000000000000000000 ) ) ;
#156256=CARTESIAN_POINT ( 'NONE',  ( 7.189988563920103104, 15.44736672437920433, 9.558790995692916681 ) ) ;
#156312=CARTESIAN_POINT ( 'NONE',  ( -15.75000000000000000, 10.90000000000000036, -1.100000000000002087 ) ) ;
#156318=CARTESIAN_POINT ( 'NONE',  ( -0.8956962585354001360, 14.55305237108631466, -11.95586207031294101 ) ) ;
#156322=CIRCLE ( 'NONE', #62915, 11.09999999999999964 ) ;
#156337=COLOUR_RGB ( '', 0.66274510, 0.83137255, 0.94901961) ;
#156373=CARTESIAN_POINT ( 'NONE',  ( -11.44779963594988814, 10.90000000000000036, -3.600000000000000977 ) ) ;
#156400=CARTESIAN_POINT ( 'NONE',  ( 8.826461557825265203, 13.26498588611182505, 7.661703860454772474 ) ) ;
#156413=ORIENTED_EDGE ( 'NONE', *, *, #121519, .F. ) ;
#156416=CARTESIAN_POINT ( 'NONE',  ( 9.475937985776971217, 4.398642190548649467, -7.290290962746341918 ) ) ;
#156430=EDGE_CURVE ( 'NONE', #145411, #72859, #213882, .T. ) ;
#156431=DIRECTION ( 'NONE',  ( 1.000000000000000000, -0.000000000000000000, -0.000000000000000000 ) ) ;
#156436=AXIS2_PLACEMENT_3D ( 'NONE', #152826, #187449, #202613 ) ;
#156459=CARTESIAN_POINT ( 'NONE',  ( -11.84668730067608600, 19.00000000000000000, 1.319999999999998286 ) ) ;
#156483=SURFACE_STYLE_USAGE ( .BOTH. , #92569 ) ;
#156502=CARTESIAN_POINT ( 'NONE',  ( 10.21213376015692909, 9.983165060110801292, -6.481890735896122635 ) ) ;
#156509=CARTESIAN_POINT ( 'NONE',  ( 6.870046935992006887, 15.99925261518604636, 9.444314260337707267 ) ) ;
#156543=CARTESIAN_POINT ( 'NONE',  ( -11.65676533170044138, 6.358709890710655621, 4.978123860300238235 ) ) ;
#156548=CARTESIAN_POINT ( 'NONE',  ( -11.07790593930098311, 9.799999999999998934, 0.6999999999999992895 ) ) ;
#156563=DIRECTION ( 'NONE',  ( 1.000000000000000000, -0.000000000000000000, -0.000000000000000000 ) ) ;
#156576=CIRCLE ( 'NONE', #115190, 12.00000000000000178 ) ;
#156580=FACE_OUTER_BOUND ( 'NONE', #117459, .T. ) ;
#156596=COLOUR_RGB ( '', 0.40784314, 0.44705882, 0.49803922) ;
#156635=ORIENTED_EDGE ( 'NONE', *, *, #13181, .F. ) ;
#156656=CARTESIAN_POINT ( 'NONE',  ( -10.85762644215163775, 5.701980886241464042, -6.452002860825420960 ) ) ;
#156663=CARTESIAN_POINT ( 'NONE',  ( 7.872268696974136226, 14.32328115913407096, 9.059783805236799381 ) ) ;
#156674=DIRECTION ( 'NONE',  ( -0.000000000000000000, -1.000000000000000000, 0.000000000000000000 ) ) ;
#156687=VERTEX_POINT ( 'NONE', #161988 ) ;
#156690=EDGE_CURVE ( 'NONE', #156842, #156205, #8499, .T. ) ;
#156701=CARTESIAN_POINT ( 'NONE',  ( 0.000000000000000000, 15.00000000000000000, -12.18000000000000149 ) ) ;
#156734=CARTESIAN_POINT ( 'NONE',  ( -10.65086514279933994, 4.118349190211191058, -6.883315229069521202 ) ) ;
#156764=EDGE_CURVE ( 'NONE', #173456, #113953, #74231, .T. ) ;
#156796=CARTESIAN_POINT ( 'NONE',  ( 11.97929049433705373, 11.37999999999999901, -0.7046979865771834106 ) ) ;
#156823=DIRECTION ( 'NONE',  ( 0.000000000000000000, 0.000000000000000000, -1.000000000000000000 ) ) ;
#156824=DIRECTION ( 'NONE',  ( 1.000000000000000000, -0.000000000000000000, -0.000000000000000000 ) ) ;
#156826=DIRECTION ( 'NONE',  ( 0.000000000000000000, 0.000000000000000000, -1.000000000000000000 ) ) ;
#156832=CARTESIAN_POINT ( 'NONE',  ( 11.07131242353766254, 13.80000000000000071, -0.8043462106219256835 ) ) ;
#156833=ADVANCED_FACE ( 'NONE', ( #97000 ), #11905, .T. ) ;
#156842=VERTEX_POINT ( 'NONE', #28776 ) ;
#156843=STYLED_ITEM ( 'NONE', ( #205294 ), #55827 ) ;
#156862=CARTESIAN_POINT ( 'NONE',  ( -11.81905481421901705, 11.25735655617265074, 1.592167362352176818 ) ) ;
#156870=PRESENTATION_STYLE_ASSIGNMENT (( #173123 ) ) ;
#156892=CARTESIAN_POINT ( 'NONE',  ( -9.356550365033054817, 15.43420774010369811, -7.432331899221634508 ) ) ;
#156915=CARTESIAN_POINT ( 'NONE',  ( -11.44791656467458374, 9.799999999999982947, 3.303228920649577294 ) ) ;
#156916=CYLINDRICAL_SURFACE ( 'NONE', #128993, 0.07999999999999998779 ) ;
#156931=CARTESIAN_POINT ( 'NONE',  ( 0.000000000000000000, 19.00000000000000000, 0.000000000000000000 ) ) ;
#156932=CARTESIAN_POINT ( 'NONE',  ( -11.25552992593869206, 3.531787801817266370, 5.933966561491729408 ) ) ;
#156937=CARTESIAN_POINT ( 'NONE',  ( -11.86239285000045918, 11.30000000000000249, -1.812080536912752837 ) ) ;
#156940=ORIENTED_EDGE ( 'NONE', *, *, #142360, .F. ) ;
#156944=DIRECTION ( 'NONE',  ( -0.000000000000000000, -1.000000000000000000, -0.000000000000000000 ) ) ;
#156958=CARTESIAN_POINT ( 'NONE',  ( 10.95308175811721085, 11.29999999999999893, -1.800000000000001155 ) ) ;
#156986=CARTESIAN_POINT ( 'NONE',  ( -2.226451178929228281, 14.55178036729105884, 11.75480792874617819 ) ) ;
#156990=AXIS2_PLACEMENT_3D ( 'NONE', #146746, #212765, #64400 ) ;
#157001=CARTESIAN_POINT ( 'NONE',  ( -9.604686356149274573, 3.530917816115240804, 7.193747284969077782 ) ) ;
#157010=EDGE_CURVE ( 'NONE', #43590, #182367, #118605, .T. ) ;
#157012=CARTESIAN_POINT ( 'NONE',  ( -11.06296324151031918, 11.25662273973621730, 0.9090245397293565954 ) ) ;
#157024=B_SPLINE_CURVE_WITH_KNOTS ( 'NONE', 3,
 ( #119142, #49816, #34624, #166771, #18367, #84444 ),
 .UNSPECIFIED., .F., .F.,
 ( 4, 2, 4 ),
 ( 0.001889712630306643673, 0.002203932548491402497, 0.002518152466676161320 ),
 .UNSPECIFIED. ) ;
#157029=CARTESIAN_POINT ( 'NONE',  ( -6.739251124622717803, 15.51951738225662325, 9.939126542081607951 ) ) ;
#157031=CARTESIAN_POINT ( 'NONE',  ( -11.92619526913699524, 10.07219975838509818, -1.328859060402685976 ) ) ;
#157044=CARTESIAN_POINT ( 'NONE',  ( 11.92559808404167576, 7.608499137140611879, 0.8913980220144042121 ) ) ;
#157048=DIRECTION ( 'NONE',  ( 0.000000000000000000, 1.000000000000000000, 0.000000000000000000 ) ) ;
#157066=FACE_OUTER_BOUND ( 'NONE', #70527, .T. ) ;
#157076=CARTESIAN_POINT ( 'NONE',  ( -10.55163518180063242, 5.124035624933899413, 7.011265714045999076 ) ) ;
#157090=ORIENTED_EDGE ( 'NONE', *, *, #24698, .F. ) ;
#157094=ORIENTED_EDGE ( 'NONE', *, *, #187841, .F. ) ;
#157106=ORIENTED_EDGE ( 'NONE', *, *, #39019, .F. ) ;
#157125=CARTESIAN_POINT ( 'NONE',  ( -9.719589822879429519, 3.553060291783284974, -6.966707445246908215 ) ) ;
#157128=CARTESIAN_POINT ( 'NONE',  ( -11.41381675112453387, 10.19999999999998153, 3.704697986577180746 ) ) ;
#157161=CARTESIAN_POINT ( 'NONE',  ( -10.84253909858433218, 4.919570308430900596, -5.035411995924089723 ) ) ;
#157163=CARTESIAN_POINT ( 'NONE',  ( 0.000000000000000000, 19.00000000000000000, 0.000000000000000000 ) ) ;
#157187=EDGE_CURVE ( 'NONE', #132416, #14896, #159555, .T. ) ;
#157188=CARTESIAN_POINT ( 'NONE',  ( 10.50000000000000533, 13.50841679891518687, -3.600000000000000533 ) ) ;
#157191=VERTEX_POINT ( 'NONE', #117068 ) ;
#157210=CARTESIAN_POINT ( 'NONE',  ( 9.482679952114482447, 14.00853213111861351, 8.402045824544956076 ) ) ;
#157224=CARTESIAN_POINT ( 'NONE',  ( 11.94105721237523277, 12.69999999999999929, 1.187919463087245386 ) ) ;
#157261=ORIENTED_EDGE ( 'NONE', *, *, #184187, .T. ) ;
#157307=SURFACE_STYLE_FILL_AREA ( #40358 ) ;
#157324=SURFACE_SIDE_STYLE ('',( #44644 ) ) ;
#157336=UNCERTAINTY_MEASURE_WITH_UNIT (LENGTH_MEASURE( 1.000000000000000082E-05 ), #54350, 'distance_accuracy_value', 'NONE');
#157341=CARTESIAN_POINT ( 'NONE',  ( 0.3554123170483105554, 14.00000000000028955, -12.67999999502907649 ) ) ;
#157346=VERTEX_POINT ( 'NONE', #25886 ) ;
#157347=ORIENTED_EDGE ( 'NONE', *, *, #73875, .T. ) ;
#157362=VECTOR ( 'NONE', #121648, 1000.000000000000000 ) ;
#157386=CARTESIAN_POINT ( 'NONE',  ( -10.52284260640670688, 5.420240069097000735, -5.071998063130033430 ) ) ;
#157408=EDGE_CURVE ( 'NONE', #177833, #45474, #77622, .T. ) ;
#157446=CARTESIAN_POINT ( 'NONE',  ( -11.43195036480942051, 11.15524496285257783, -3.649565797774410036 ) ) ;
#157454=DIRECTION ( 'NONE',  ( -0.9486832980505139901, -0.3162277660168373861, 3.312310031615527941E-15 ) ) ;
#157457=CARTESIAN_POINT ( 'NONE',  ( 10.87378820908022625, 9.632687173196126551, -5.088116269538504710 ) ) ;
#157463=CARTESIAN_POINT ( 'NONE',  ( -11.44779964734699540, 13.49810470129609286, 3.599999963171390593 ) ) ;
#157475=CARTESIAN_POINT ( 'NONE',  ( 10.48926859151676005, 8.662495522311813190, -6.550045777748900733 ) ) ;
#157479=CARTESIAN_POINT ( 'NONE',  ( -3.111427826557872756, 14.48006665645140956, -11.59831528793133337 ) ) ;
#157483=ORIENTED_EDGE ( 'NONE', *, *, #140722, .T. ) ;
#157492=FACE_OUTER_BOUND ( 'NONE', #149465, .T. ) ;
#157528=DIRECTION ( 'NONE',  ( 1.000000000000000000, -0.000000000000000000, -0.000000000000000000 ) ) ;
#157553=FACE_OUTER_BOUND ( 'NONE', #48476, .T. ) ;
#157558=AXIS2_PLACEMENT_3D ( 'NONE', #195824, #165448, #98326 ) ;
#157562=SURFACE_STYLE_FILL_AREA ( #120854 ) ;
#157580=CARTESIAN_POINT ( 'NONE',  ( 10.09133975709188213, 13.93637380468759623, 7.385690965161497701 ) ) ;
#157600=CARTESIAN_POINT ( 'NONE',  ( 11.95360554405587017, 9.995550034974165499, 1.059413164304713773 ) ) ;
#157612=CARTESIAN_POINT ( 'NONE',  ( -11.38502332509229831, 5.468749262791421373, -5.576278951475440948 ) ) ;
#157613=ORIENTED_EDGE ( 'NONE', *, *, #47233, .F. ) ;
#157637=CARTESIAN_POINT ( 'NONE',  ( 10.41968677110260089, 10.52501210740200754, 5.960825342340682731 ) ) ;
#157649=CARTESIAN_POINT ( 'NONE',  ( 11.04536101718726293, 13.40000000000000036, 1.099999999999996758 ) ) ;
#157693=B_SPLINE_CURVE_WITH_KNOTS ( 'NONE', 3,
 ( #132068, #129980, #214287, #146170, #51853, #150425 ),
 .UNSPECIFIED., .F., .F.,
 ( 4, 2, 4 ),
 ( 0.001259240562161249421, 0.001573673787268791650, 0.001888107012376333878 ),
 .UNSPECIFIED. ) ;
#157703=AXIS2_PLACEMENT_3D ( 'NONE', #109818, #113019, #81513 ) ;
#157729=CARTESIAN_POINT ( 'NONE',  ( -10.91449010664383223, 5.922815305582411760, 6.336942051301835299 ) ) ;
#157743=EDGE_LOOP ( 'NONE', ( #234, #98419, #176118, #107692 ) ) ;
#157756=CARTESIAN_POINT ( 'NONE',  ( -11.86145016429273014, 10.90000000000000036, -1.100000000000002087 ) ) ;
#157767=CARTESIAN_POINT ( 'NONE',  ( 9.367496997597600128, 3.481540744127370690, 7.500000000000001776 ) ) ;
#157784=COLOUR_RGB ( '', 0.72549020, 0.75294118, 0.79215686) ;
#157787=ADVANCED_FACE ( 'NONE', ( #205705 ), #117439, .F. ) ;
#157796=CARTESIAN_POINT ( 'NONE',  ( -15.75000000000000000, 13.40000000000000036, -1.800000000000001155 ) ) ;
#157801=CARTESIAN_POINT ( 'NONE',  ( -9.409940793360268785, 3.999985931113709814, -6.919963696468023784 ) ) ;
#157806=ORIENTED_EDGE ( 'NONE', *, *, #195600, .F. ) ;
#157818=AXIS2_PLACEMENT_3D ( 'NONE', #101317, #167399, #20054 ) ;
#157826=SURFACE_STYLE_FILL_AREA ( #57110 ) ;
#157868=CARTESIAN_POINT ( 'NONE',  ( 11.44779963594995564, 12.69999999999997797, 3.600000000000075140 ) ) ;
#157870=CARTESIAN_POINT ( 'NONE',  ( 11.75830593302511851, 6.921630077720365648, 2.442185041723917927 ) ) ;
#157883=ORIENTED_EDGE ( 'NONE', *, *, #69142, .F. ) ;
#157886=CARTESIAN_POINT ( 'NONE',  ( 11.91826848330682154, 10.09270354043018436, 1.400000080589831608 ) ) ;
#157903=CARTESIAN_POINT ( 'NONE',  ( 11.97929049433705551, 11.29999999999999893, 0.7046979865771804130 ) ) ;
#157904=CARTESIAN_POINT ( 'NONE',  ( 9.451968220918345764, 11.05088267330476448, -7.322606453075928279 ) ) ;
#157932=CARTESIAN_POINT ( 'NONE',  ( 11.49978884755362252, 9.857291788371890462, 3.429452816445146546 ) ) ;
#157975=MECHANICAL_DESIGN_GEOMETRIC_PRESENTATION_REPRESENTATION('',(#23105),#213280);
#157978=CARTESIAN_POINT ( 'NONE',  ( 0.000000000000000000, 4.000007913748540922, 0.000000000000000000 ) ) ;
#158000=CARTESIAN_POINT ( 'NONE',  ( -11.86145017031048177, 13.50581953513855105, 1.099999999999996980 ) ) ;
#158001=CARTESIAN_POINT ( 'NONE',  ( -10.12531724201500616, 3.239403609407997653, 5.873437370650227862 ) ) ;
#158007=CARTESIAN_POINT ( 'NONE',  ( -11.87815913191725947, 11.30307820631414550, -1.708869976696590465 ) ) ;
#158041=CARTESIAN_POINT ( 'NONE',  ( 1.359357947053562156E-15, 18.91999999999999815, -11.09999999999999964 ) ) ;
#158047=VERTEX_POINT ( 'NONE', #94129 ) ;
#158065=( NAMED_UNIT ( * ) SI_UNIT ( $, .STERADIAN. ) SOLID_ANGLE_UNIT ( ) );
#158068=CARTESIAN_POINT ( 'NONE',  ( -10.47316218909242025, 3.890729455492532018, 5.858813772850529844 ) ) ;
#158097=DIRECTION ( 'NONE',  ( -0.000000000000000000, -1.000000000000000000, -0.000000000000000000 ) ) ;
#158109=CARTESIAN_POINT ( 'NONE',  ( -10.98546401119367566, 9.842594370796488690, 1.592223900679732518 ) ) ;
#158131=CARTESIAN_POINT ( 'NONE',  ( 11.78331023100045627, 11.29999999999998117, 1.799999999999999600 ) ) ;
#158141=CARTESIAN_POINT ( 'NONE',  ( -9.645001968711920171, 4.042125922905831281, 6.587946042608958663 ) ) ;
#158156=( NAMED_UNIT ( * ) PLANE_ANGLE_UNIT ( ) SI_UNIT ( $, .RADIAN. ) );
#158158=MECHANICAL_DESIGN_GEOMETRIC_PRESENTATION_REPRESENTATION('',(#68271),#182395);
#158160=EDGE_LOOP ( 'NONE', ( #9920, #155928, #182080, #67700 ) ) ;
#158166=EDGE_CURVE ( 'NONE', #118849, #51477, #10701, .T. ) ;
#158225=CARTESIAN_POINT ( 'NONE',  ( 10.59781858645781405, 13.79999999999998295, 3.302687032930892830 ) ) ;
#158260=CARTESIAN_POINT ( 'NONE',  ( 11.92619526913699879, 19.00000000000000000, 1.328859060402684644 ) ) ;
#158262=CARTESIAN_POINT ( 'NONE',  ( 0.000000000000000000, 0.08000000000000020983, -12.00000000000000178 ) ) ;
#158278=VECTOR ( 'NONE', #122950, 1000.000000000000000 ) ;
#158286=CARTESIAN_POINT ( 'NONE',  ( -11.89942855770814134, 9.799999999999998934, -0.7000000000000009548 ) ) ;
#158301=CARTESIAN_POINT ( 'NONE',  ( -11.33772463945036968, 13.40000000000000036, -3.600000000000000977 ) ) ;
#158363=FILL_AREA_STYLE_COLOUR ( '', #174229 ) ;
#158372=SURFACE_STYLE_USAGE ( .BOTH. , #73912 ) ;
#158383=CARTESIAN_POINT ( 'NONE',  ( 6.902720145097990034, 15.44736672593548299, 9.761920446463546952 ) ) ;
#158401=CARTESIAN_POINT ( 'NONE',  ( 11.41381675112460847, 10.06983264508522424, 3.704697986577264235 ) ) ;
#158402=VERTEX_POINT ( 'NONE', #16015 ) ;
#158420=AXIS2_PLACEMENT_3D ( 'NONE', #163083, #147895, #50378 ) ;
#158425=CARTESIAN_POINT ( 'NONE',  ( -10.46647149127475451, 4.016265686976439042, 5.778904458337481564 ) ) ;
#158439=CARTESIAN_POINT ( 'NONE',  ( 11.84668730067608244, 13.50636224908217287, 1.399999999999998357 ) ) ;
#158470=CARTESIAN_POINT ( 'NONE',  ( 11.88237264505823987, 11.25677038468308844, -0.9087825512663076921 ) ) ;
#158473=ORIENTED_EDGE ( 'NONE', *, *, #139797, .F. ) ;
#158500=CARTESIAN_POINT ( 'NONE',  ( -11.35573736746281348, 11.11270414413282204, -3.554362808847921773 ) ) ;
#158512=CARTESIAN_POINT ( 'NONE',  ( 12.00020500325193318, 7.639630528669115073, -0.2084710905185198637 ) ) ;
#158519=DIRECTION ( 'NONE',  ( 0.000000000000000000, 0.000000000000000000, 1.000000000000000000 ) ) ;
#158529=CARTESIAN_POINT ( 'NONE',  ( 8.995095802688167552, 12.46245326214662086, -7.469535370069887215 ) ) ;
#158545=CARTESIAN_POINT ( 'NONE',  ( 9.367496997597640984, 4.518459255873318092, -7.499999999999949374 ) ) ;
#158575=CARTESIAN_POINT ( 'NONE',  ( 11.92045683181315141, 12.44724072120514791, -1.382340670101858571 ) ) ;
#158585=CARTESIAN_POINT ( 'NONE',  ( 0.000000000000000000, 13.79999999999999893, 0.000000000000000000 ) ) ;
#158588=CARTESIAN_POINT ( 'NONE',  ( -9.117697077659890681, 14.00000000000575007, 7.299999999991188204 ) ) ;
#158613=EDGE_CURVE ( 'NONE', #23152, #197638, #159801, .T. ) ;
#158619=CARTESIAN_POINT ( 'NONE',  ( -11.41176686791169281, 11.25950803486852081, 3.404018756831824533 ) ) ;
#158631=DIRECTION ( 'NONE',  ( 0.000000000000000000, -1.445602896647338917E-16, 1.000000000000000000 ) ) ;
#158637=CARTESIAN_POINT ( 'NONE',  ( 9.571964790107170273, 13.80900892610533859, 8.297589824372789025 ) ) ;
#158656=CARTESIAN_POINT ( 'NONE',  ( 11.86145016429273191, 10.19999999999999929, 1.099999999999996980 ) ) ;
#158668=MECHANICAL_DESIGN_GEOMETRIC_PRESENTATION_REPRESENTATION('',(#44419),#210440);
#158670=CARTESIAN_POINT ( 'NONE',  ( -11.30310531956832776, 5.150576456239970291, 5.742040133384030298 ) ) ;
#158693=VERTEX_POINT ( 'NONE', #178201 ) ;
#158694=CARTESIAN_POINT ( 'NONE',  ( 11.82867183089590135, 7.768921039415717544, 1.758246007359564933 ) ) ;
#158705=( BOUNDED_SURFACE ( )  B_SPLINE_SURFACE ( 3, 3, ( 
 ( #143487, #26483, #27555, #93651, #159694, #23262, #89374, #190050, #107812, #15551, #13433, #30779, #178089, #81638, #96858, #211624, #162906, #147723 ),
 ( #213740, #65363, #179155, #148778, #348, #14488, #146676, #210567, #212691, #95788, #112088, #131510, #113149, #197513, #80578, #97916, #66421, #64333 ),
 ( #114219, #94720, #82697, #132564, #28633, #130474, #111011, #29707, #163975, #196465, #44903, #31840, #161845, #16616, #45967, #48107, #49157, #115273 ),
 ( #177016, #160763, #181266, #79509, #32892, #145627, #98970, #195404, #165022, #63259, #194325, #12358, #47034, #180218, #78437, #144557, #62201, #128357 ),
 ( #129421, #199636, #2489, #19825, #85910, #200695, #151984, #52346, #186600, #18754, #51282, #37150, #202830, #35007, #54478, #117407, #67488, #17678 ),
 ( #1425, #133634, #102160, #21935, #183403, #53402, #38227, #101078, #68564, #167167, #198565, #182323, #118474, #84838, #150928, #33952, #5686, #134691 ),
 ( #3558, #184459, #104301, #136804, #36077, #116333, #169290, #168228, #166090, #69630, #135739, #201761, #86974, #119540, #149857, #120624, #185525, #103230 ) ),
 .UNSPECIFIED., .T., .F., .T. ) 
 B_SPLINE_SURFACE_WITH_KNOTS ( ( 4, 3, 4 ),
 ( 4, 2, 2, 2, 2, 2, 2, 2, 4 ),
 ( 0.000000000000000000, 0.5000000000000000000, 1.000000000000000000 ),
 ( 0.1651814497726892539, 0.1751754979096289411, 0.1851695460465686560, 0.2051576423204480859, 0.2251452996291458120, 0.2351391282834946750, 0.2401360426106691204, 0.2426344997742563292, 0.2451329569378435380 ),
 .UNSPECIFIED. ) 
 GEOMETRIC_REPRESENTATION_ITEM ( )  RATIONAL_B_SPLINE_SURFACE ( (
 ( 1.000000000000000000, 1.000000000000000000, 1.000000000000000000, 1.000000000000000000, 1.000000000000000000, 1.000000000000000000, 1.000000000000000000, 1.000000000000000000, 1.000000000000000000, 1.000000000000000000, 1.000000000000000000, 1.000000000000000000, 1.000000000000000000, 1.000000000000000000, 1.000000000000000000, 1.000000000000000000, 1.000000000000000000, 1.000000000000000000),
 ( 0.3333333333333333703, 0.3333333333333333703, 0.3333333333333333703, 0.3333333333333333703, 0.3333333333333333703, 0.3333333333333333703, 0.3333333333333333703, 0.3333333333333333703, 0.3333333333333333703, 0.3333333333333333703, 0.3333333333333333703, 0.3333333333333333703, 0.3333333333333333703, 0.3333333333333333703, 0.3333333333333333703, 0.3333333333333333703, 0.3333333333333333703, 0.3333333333333333703),
 ( 0.3333333333333333703, 0.3333333333333333703, 0.3333333333333333703, 0.3333333333333333703, 0.3333333333333333703, 0.3333333333333333703, 0.3333333333333333703, 0.3333333333333333703, 0.3333333333333333703, 0.3333333333333333703, 0.3333333333333333703, 0.3333333333333333703, 0.3333333333333333703, 0.3333333333333333703, 0.3333333333333333703, 0.3333333333333333703, 0.3333333333333333703, 0.3333333333333333703),
 ( 1.000000000000000000, 1.000000000000000000, 1.000000000000000000, 1.000000000000000000, 1.000000000000000000, 1.000000000000000000, 1.000000000000000000, 1.000000000000000000, 1.000000000000000000, 1.000000000000000000, 1.000000000000000000, 1.000000000000000000, 1.000000000000000000, 1.000000000000000000, 1.000000000000000000, 1.000000000000000000, 1.000000000000000000, 1.000000000000000000),
 ( 0.3333333333333333703, 0.3333333333333333703, 0.3333333333333333703, 0.3333333333333333703, 0.3333333333333333703, 0.3333333333333333703, 0.3333333333333333703, 0.3333333333333333703, 0.3333333333333333703, 0.3333333333333333703, 0.3333333333333333703, 0.3333333333333333703, 0.3333333333333333703, 0.3333333333333333703, 0.3333333333333333703, 0.3333333333333333703, 0.3333333333333333703, 0.3333333333333333703),
 ( 0.3333333333333333703, 0.3333333333333333703, 0.3333333333333333703, 0.3333333333333333703, 0.3333333333333333703, 0.3333333333333333703, 0.3333333333333333703, 0.3333333333333333703, 0.3333333333333333703, 0.3333333333333333703, 0.3333333333333333703, 0.3333333333333333703, 0.3333333333333333703, 0.3333333333333333703, 0.3333333333333333703, 0.3333333333333333703, 0.3333333333333333703, 0.3333333333333333703),
 ( 1.000000000000000000, 1.000000000000000000, 1.000000000000000000, 1.000000000000000000, 1.000000000000000000, 1.000000000000000000, 1.000000000000000000, 1.000000000000000000, 1.000000000000000000, 1.000000000000000000, 1.000000000000000000, 1.000000000000000000, 1.000000000000000000, 1.000000000000000000, 1.000000000000000000, 1.000000000000000000, 1.000000000000000000, 1.000000000000000000) ) ) 
 REPRESENTATION_ITEM ( '' )  SURFACE ( )  );
#158706=AXIS2_PLACEMENT_3D ( 'NONE', #17886, #82908, #49363 ) ;
#158740=( LENGTH_UNIT ( ) NAMED_UNIT ( * ) SI_UNIT ( .MILLI., .METRE. ) );
#158748=CARTESIAN_POINT ( 'NONE',  ( 11.94105721237523277, 10.90000000000000036, 1.187919463087248273 ) ) ;
#158752=AXIS2_PLACEMENT_3D ( 'NONE', #85373, #167690, #99496 ) ;
#158765=ORIENTED_EDGE ( 'NONE', *, *, #183072, .F. ) ;
#158767=VERTEX_POINT ( 'NONE', #63374 ) ;
#158773=CARTESIAN_POINT ( 'NONE',  ( -9.587917471435847716, 4.026361754648488223, -6.670783315233271615 ) ) ;
#158781=CARTESIAN_POINT ( 'NONE',  ( -10.78402850230606447, 8.013881820625746499, 4.046242669647421408 ) ) ;
#158786=CARTESIAN_POINT ( 'NONE',  ( 7.322686252399450701, 14.46639250110529673, 9.509740026712064420 ) ) ;
#158798=AXIS2_PLACEMENT_3D ( 'NONE', #193080, #198397, #182148 ) ;
#158806=EDGE_CURVE ( 'NONE', #45318, #201145, #182525, .T. ) ;
#158811=CIRCLE ( 'NONE', #117283, 0.08000000000000020983 ) ;
#158823=SURFACE_STYLE_FILL_AREA ( #58118 ) ;
#158854=CARTESIAN_POINT ( 'NONE',  ( -10.32649671959996596, 5.020010808682577874, -7.354824260697566451 ) ) ;
#158859=DIRECTION ( 'NONE',  ( 0.9885327375000381167, 0.000000000000000000, -0.1510067114093955609 ) ) ;
#158863=CARTESIAN_POINT ( 'NONE',  ( 11.86239285000045740, 12.21999999999998288, 1.812080536912751061 ) ) ;
#158903=VECTOR ( 'NONE', #84084, 1000.000000000000000 ) ;
#158912=ORIENTED_EDGE ( 'NONE', *, *, #9318, .F. ) ;
#158922=CARTESIAN_POINT ( 'NONE',  ( 9.980956060213129533, 9.821313066029905059, 6.688669764353187830 ) ) ;
#158924=STYLED_ITEM ( 'NONE', ( #109553 ), #10376 ) ;
#158936=CARTESIAN_POINT ( 'NONE',  ( 11.80251051724250821, 9.799999999999982947, 1.695257889419128361 ) ) ;
#158942=EDGE_CURVE ( 'NONE', #45474, #118849, #30271, .T. ) ;
#158955=CARTESIAN_POINT ( 'NONE',  ( 11.35777274796318359, 7.533313121839867676, -3.739796408902939628 ) ) ;
#158962=CARTESIAN_POINT ( 'NONE',  ( -9.489836703503209847, 14.79794462677083011, -7.238794765906159334 ) ) ;
#158995=CARTESIAN_POINT ( 'NONE',  ( 9.319929085041183114, 13.69254449485596226, -7.486148048470657734 ) ) ;
#159022=( NAMED_UNIT ( * ) SI_UNIT ( $, .STERADIAN. ) SOLID_ANGLE_UNIT ( ) );
#159046=CARTESIAN_POINT ( 'NONE',  ( 11.60282415082483531, 8.761450460988655209, -2.711552276110228199 ) ) ;
#159070=CARTESIAN_POINT ( 'NONE',  ( 11.92619526913699879, 19.00000000000000000, -1.328859060402686199 ) ) ;
#159075=CARTESIAN_POINT ( 'NONE',  ( -2.232280211084506583, 15.51994262677984082, -11.79897380041492916 ) ) ;
#159103=B_SPLINE_CURVE_WITH_KNOTS ( 'NONE', 3,
 ( #95116, #161165, #144946, #80969, #180598, #179548 ),
 .UNSPECIFIED., .F., .F.,
 ( 4, 2, 4 ),
 ( 0.000000000000000000, 0.0003239988925529257036, 0.0006479977851058514073 ),
 .UNSPECIFIED. ) ;
#159105=DIRECTION ( 'NONE',  ( 0.000000000000000000, -1.000000000000000000, 0.000000000000000000 ) ) ;
#159111=FILL_AREA_STYLE_COLOUR ( '', #201545 ) ;
#159114=CARTESIAN_POINT ( 'NONE',  ( -10.66890663286052465, 4.188823345043420687, 5.493879390884747416 ) ) ;
#159157=CARTESIAN_POINT ( 'NONE',  ( 11.94524591058472041, 7.576283193003019889, -0.4340265584551949996 ) ) ;
#159188=ORIENTED_EDGE ( 'NONE', *, *, #84048, .T. ) ;
#159191=UNCERTAINTY_MEASURE_WITH_UNIT (LENGTH_MEASURE( 1.000000000000000082E-05 ), #22164, 'distance_accuracy_value', 'NONE');
#159234=CARTESIAN_POINT ( 'NONE',  ( 0.1448469644582885130, 14.55305575109302829, 11.95498533988372891 ) ) ;
#159243=DIRECTION ( 'NONE',  ( -0.000000000000000000, 1.000000000000000000, -0.000000000000000000 ) ) ;
#159264=AXIS2_PLACEMENT_3D ( 'NONE', #208599, #79685, #192350 ) ;
#159268=CARTESIAN_POINT ( 'NONE',  ( 11.44779965693254198, 12.60313923201305641, -3.599999932276613634 ) ) ;
#159273=VERTEX_POINT ( 'NONE', #141510 ) ;
#159286=DIRECTION ( 'NONE',  ( 0.000000000000000000, 0.000000000000000000, 1.000000000000000000 ) ) ;
#159302=CARTESIAN_POINT ( 'NONE',  ( -15.75000000000000000, 13.40000000000000036, -1.800000000000001155 ) ) ;
#159307=CARTESIAN_POINT ( 'NONE',  ( -11.89317557362582356, 13.76275843837616542, -1.599935658896116664 ) ) ;
#159333=CARTESIAN_POINT ( 'NONE',  ( -11.96535697748077887, 9.847373329355578520, -0.9148528286455027692 ) ) ;
#159412=PRESENTATION_STYLE_ASSIGNMENT (( #22986 ) ) ;
#159438=CARTESIAN_POINT ( 'NONE',  ( -15.75000000000000000, 10.90000000000000036, 1.099999999999996758 ) ) ;
#159463=VECTOR ( 'NONE', #8423, 1000.000000000000000 ) ;
#159505=CARTESIAN_POINT ( 'NONE',  ( -3.111406510290429139, 14.52977256516549964, -11.59832018432755163 ) ) ;
#159555=B_SPLINE_CURVE_WITH_KNOTS ( 'NONE', 3,
 ( #150590, #149512, #133293, #199299, #50944, #116003, #32558 ),
 .UNSPECIFIED., .F., .F.,
 ( 4, 3, 4 ),
 ( -0.0002318125648490629992, 2.710505431213761085E-20, 0.0004044109710639540861 ),
 .UNSPECIFIED. ) ;
#159560=( GEOMETRIC_REPRESENTATION_CONTEXT ( 3 ) GLOBAL_UNCERTAINTY_ASSIGNED_CONTEXT ( ( #148036 ) ) GLOBAL_UNIT_ASSIGNED_CONTEXT ( ( #49298, #83898, #183534 ) ) REPRESENTATION_CONTEXT ( 'NONE', 'WORKASPACE' ) );
#159569=DIRECTION ( 'NONE',  ( 0.05872483221476459958, 0.000000000000000000, -0.9982742078614211811 ) ) ;
#159572=CARTESIAN_POINT ( 'NONE',  ( 9.979653537509710404, 11.54805711219047382, 6.669254315307292735 ) ) ;
#159590=CARTESIAN_POINT ( 'NONE',  ( 8.433970489975340712, 12.79606745324766059, -8.483499499578806891 ) ) ;
#159624=CARTESIAN_POINT ( 'NONE',  ( -11.33772463945036968, 10.90000000000000036, -3.600000000000002309 ) ) ;
#159627=CARTESIAN_POINT ( 'NONE',  ( -11.96533679318059917, 11.25246011187005202, -0.9151144679398750537 ) ) ;
#159651=CARTESIAN_POINT ( 'NONE',  ( -11.33183379859914552, 6.587777300838509653, -3.814615888199307747 ) ) ;
#159654=CARTESIAN_POINT ( 'NONE',  ( 0.3263184169969229886, 16.00000000000058265, 11.67999999558625213 ) ) ;
#159666=ORIENTED_EDGE ( 'NONE', *, *, #199418, .F. ) ;
#159679=SURFACE_STYLE_FILL_AREA ( #93637 ) ;
#159690=SURFACE_STYLE_USAGE ( .BOTH. , #27551 ) ;
#159694=CARTESIAN_POINT ( 'NONE',  ( 7.948861177221683505, 14.94981965669310853, -9.879624537148666619 ) ) ;
#159697=CARTESIAN_POINT ( 'NONE',  ( 9.163219433650940715, 13.31059121366393860, 9.059053262848197008 ) ) ;
#159731=CARTESIAN_POINT ( 'NONE',  ( -10.97400665845581536, 4.893988168282350948, 4.351071648605314479 ) ) ;
#159756=CARTESIAN_POINT ( 'NONE',  ( 11.99415247035267029, 7.596933813522314338, -0.4356545883255271701 ) ) ;
#159801=LINE ( 'NONE', #128466, #120846 ) ;
#159806=CARTESIAN_POINT ( 'NONE',  ( 0.07968937631763337026, 14.48280408365269345, 11.99973206003984316 ) ) ;
#159808=CARTESIAN_POINT ( 'NONE',  ( 11.96215121607992771, 11.32833553780823799, 0.9565349792967585696 ) ) ;
#159815=CYLINDRICAL_SURFACE ( 'NONE', #40272, 0.3999999999999997446 ) ;
#159831=AXIS2_PLACEMENT_3D ( 'NONE', #2010, #104900, #53997 ) ;
#159845=CARTESIAN_POINT ( 'NONE',  ( -10.02504487015220569, 5.769816241140256707, -5.888073156868665059 ) ) ;
#159850=DIRECTION ( 'NONE',  ( 0.000000000000000000, -1.000000000000000000, -0.000000000000000000 ) ) ;
#159860=VERTEX_POINT ( 'NONE', #183543 ) ;
#159874=CARTESIAN_POINT ( 'NONE',  ( 1.369155121446740960E-15, 1.016439536705160407E-16, -11.18000000000000149 ) ) ;
#159886=CARTESIAN_POINT ( 'NONE',  ( -0.008622056139523381901, 15.44694768828586540, 11.95585894197802013 ) ) ;
#159907=CARTESIAN_POINT ( 'NONE',  ( -11.86145016429273191, 10.19999999999999929, 1.099999999999996758 ) ) ;
#159919=CARTESIAN_POINT ( 'NONE',  ( -10.57449672806501262, 3.061848070889987561, -7.008429158759065913 ) ) ;
#159989=VECTOR ( 'NONE', #191775, 1000.000000000000000 ) ;
#159998=ORIENTED_EDGE ( 'NONE', *, *, #20380, .T. ) ;
#160017=DIRECTION ( 'NONE',  ( 1.000000000000000000, -0.000000000000000000, -0.000000000000000000 ) ) ;
#160019=CARTESIAN_POINT ( 'NONE',  ( 9.005029904505741811, 12.36406115350124502, 7.861980445344781465 ) ) ;
#160023=CARTESIAN_POINT ( 'NONE',  ( -9.960032942013363311, 4.511256714876205720, 6.620518269535303091 ) ) ;
#160027=CARTESIAN_POINT ( 'NONE',  ( -9.351030442090584316, 14.56056703928365259, -7.441731297699171854 ) ) ;
#160029=ORIENTED_EDGE ( 'NONE', *, *, #132358, .T. ) ;
#160054=CARTESIAN_POINT ( 'NONE',  ( 1.250000000000037526, 8.500000000000000000, 11.02939254900286237 ) ) ;
#160057=DIRECTION ( 'NONE',  ( -0.000000000000000000, -1.000000000000000000, -0.000000000000000000 ) ) ;
#160069=MECHANICAL_DESIGN_GEOMETRIC_PRESENTATION_REPRESENTATION('',(#149722),#80605);
#160109=CARTESIAN_POINT ( 'NONE',  ( 10.32808049211214652, 11.37156981856230686, -7.280726186550563028 ) ) ;
#160118=SURFACE_STYLE_USAGE ( .BOTH. , #127714 ) ;
#160126=AXIS2_PLACEMENT_3D ( 'NONE', #90517, #57997, #213555 ) ;
#160141=CARTESIAN_POINT ( 'NONE',  ( -10.39336823037077195, 4.932734307774878424, -5.330979603150785451 ) ) ;
#160181=CARTESIAN_POINT ( 'NONE',  ( -10.85972455493619471, 4.659241855712780378, 5.106971684771559161 ) ) ;
#160224=FACE_OUTER_BOUND ( 'NONE', #181113, .T. ) ;
#160246=CARTESIAN_POINT ( 'NONE',  ( -11.97929049433705373, 12.22000000000000064, 0.7046979865771783036 ) ) ;
#160259=ORIENTED_EDGE ( 'NONE', *, *, #49979, .T. ) ;
#160284=ORIENTED_EDGE ( 'NONE', *, *, #56195, .F. ) ;
#160285=DIRECTION ( 'NONE',  ( -0.9632918427306580433, 0.000000000000000000, 0.2684563758389303945 ) ) ;
#160286=CIRCLE ( 'NONE', #8135, 0.07999999999999998779 ) ;
#160288=AXIS2_PLACEMENT_3D ( 'NONE', #107855, #3843, #206338 ) ;
#160308=CARTESIAN_POINT ( 'NONE',  ( -1.674002081864904623, 14.52982574599248977, 11.91747069027295858 ) ) ;
#160317=DIRECTION ( 'NONE',  ( 0.000000000000000000, 0.000000000000000000, 1.000000000000000000 ) ) ;
#160321=CARTESIAN_POINT ( 'NONE',  ( 11.48806469435255551, 11.33089772872448719, -3.468902948106704631 ) ) ;
#160330=LINE ( 'NONE', #126850, #102113 ) ;
#160342=CARTESIAN_POINT ( 'NONE',  ( 11.91826849282518630, 10.89999999999998082, 1.399999999999996581 ) ) ;
#160359=SURFACE_STYLE_USAGE ( .BOTH. , #9832 ) ;
#160379=ORIENTED_EDGE ( 'NONE', *, *, #23681, .T. ) ;
#160384=ORIENTED_EDGE ( 'NONE', *, *, #178173, .F. ) ;
#160403=CARTESIAN_POINT ( 'NONE',  ( -11.89204169242383458, 9.799999999999998934, -0.8046421800350854747 ) ) ;
#160424=CARTESIAN_POINT ( 'NONE',  ( -10.59782195348455680, 12.30000000000000071, -3.302675849420335652 ) ) ;
#160481=ORIENTED_EDGE ( 'NONE', *, *, #121920, .T. ) ;
#160485=( LENGTH_UNIT ( ) NAMED_UNIT ( * ) SI_UNIT ( .MILLI., .METRE. ) );
#160490=CARTESIAN_POINT ( 'NONE',  ( 0.000000000000000000, 12.30000000000000071, 0.000000000000000000 ) ) ;
#160505=UNCERTAINTY_MEASURE_WITH_UNIT (LENGTH_MEASURE( 1.000000000000000082E-05 ), #102376, 'distance_accuracy_value', 'NONE');
#160571=LINE ( 'NONE', #129240, #139589 ) ;
#160596=AXIS2_PLACEMENT_3D ( 'NONE', #31298, #208945, #178616 ) ;
#160612=SURFACE_STYLE_USAGE ( .BOTH. , #27403 ) ;
#160636=CARTESIAN_POINT ( 'NONE',  ( 1.500000000000053291, 7.750000000000000000, 15.74999999999999289 ) ) ;
#160640=CARTESIAN_POINT ( 'NONE',  ( 10.87278331243690133, 9.634830980282087509, 5.090122543959602730 ) ) ;
#160650=CYLINDRICAL_SURFACE ( 'NONE', #101834, 0.3999999999999996891 ) ;
#160658=COLOUR_RGB ( '', 0.08235294, 0.09019608, 0.10196078) ;
#160663=CARTESIAN_POINT ( 'NONE',  ( 13.00188123086410563, 6.790293321084564404, 2.180131930379270333 ) ) ;
#160667=ORIENTED_EDGE ( 'NONE', *, *, #132306, .F. ) ;
#160716=CARTESIAN_POINT ( 'NONE',  ( -11.41381675112453387, 10.19999999999999929, -3.704697986577184299 ) ) ;
#160719=CARTESIAN_POINT ( 'NONE',  ( -8.065673738755203104, 15.99999998465560758, 8.613976760013509093 ) ) ;
#160748=AXIS2_PLACEMENT_3D ( 'NONE', #171051, #36781, #173214 ) ;
#160759=( NAMED_UNIT ( * ) PLANE_ANGLE_UNIT ( ) SI_UNIT ( $, .RADIAN. ) );
#160763=CARTESIAN_POINT ( 'NONE',  ( 6.861939425476737853, 15.00000000000000000, -9.452896198007838535 ) ) ;
#160766=CARTESIAN_POINT ( 'NONE',  ( 6.743451644395038080, 14.99925532292382790, 9.536680772710601772 ) ) ;
#160773=B_SPLINE_CURVE_WITH_KNOTS ( 'NONE', 3,
 ( #210190, #80201, #93288, #179847, #191804, #61828 ),
 .UNSPECIFIED., .F., .F.,
 ( 4, 2, 4 ),
 ( 0.000000000000000000, 0.0003767643964918267023, 0.0007535287929836531878 ),
 .UNSPECIFIED. ) ;
#160796=AXIS2_PLACEMENT_3D ( 'NONE', #167542, #5006, #17000 ) ;
#160803=CARTESIAN_POINT ( 'NONE',  ( -12.76460961864369814, 7.407083900356914441, 2.164514475593080078 ) ) ;
#160820=CARTESIAN_POINT ( 'NONE',  ( -9.508802380631136586, 15.10175073245280686, 7.212919681869107258 ) ) ;
#160826=ORIENTED_EDGE ( 'NONE', *, *, #101740, .F. ) ;
#160827=CARTESIAN_POINT ( 'NONE',  ( 11.27149238125475428, 8.841068552745543485, 4.121733248070676758 ) ) ;
#160837=( NAMED_UNIT ( * ) PLANE_ANGLE_UNIT ( ) SI_UNIT ( $, .RADIAN. ) );
#160843=EDGE_CURVE ( 'NONE', #201330, #183276, #30706, .T. ) ;
#160853=ADVANCED_FACE ( 'NONE', ( #29633 ), #105755, .T. ) ;
#160879=CARTESIAN_POINT ( 'NONE',  ( -11.94589778161906857, 8.080793008161904822, -0.5292555138636146905 ) ) ;
#160901=ORIENTED_EDGE ( 'NONE', *, *, #181856, .T. ) ;
#160920=CARTESIAN_POINT ( 'NONE',  ( -11.47191357686926771, 5.776505007901941546, -5.393588192467421827 ) ) ;
#160939=FILL_AREA_STYLE ('',( #112252 ) ) ;
#160948=FILL_AREA_STYLE_COLOUR ( '', #128729 ) ;
#160949=CARTESIAN_POINT ( 'NONE',  ( -9.333041836230016486, 15.44694763438214125, 7.472413793098208856 ) ) ;
#160960=CARTESIAN_POINT ( 'NONE',  ( 9.476364159883866378, 3.602179703620744800, 7.289721612074727908 ) ) ;
#160964=AXIS2_PLACEMENT_3D ( 'NONE', #133574, #199580, #193468 ) ;
#160975=DIRECTION ( 'NONE',  ( -0.000000000000000000, -1.000000000000000000, -0.000000000000000000 ) ) ;
#160989=CARTESIAN_POINT ( 'NONE',  ( -10.39336823037077195, 4.932734307774878424, -5.330979603150785451 ) ) ;
#160994=ORIENTED_EDGE ( 'NONE', *, *, #158806, .T. ) ;
#161008=FACE_BOUND ( 'NONE', #40080, .T. ) ;
#161035=DIRECTION ( 'NONE',  ( 0.000000000000000000, 0.000000000000000000, -1.000000000000000000 ) ) ;
#161064=SURFACE_STYLE_USAGE ( .BOTH. , #10525 ) ;
#161070=CARTESIAN_POINT ( 'NONE',  ( -11.92619526913699879, 12.69999999999998153, 1.328859060402684644 ) ) ;
#161072=ORIENTED_EDGE ( 'NONE', *, *, #57679, .T. ) ;
#161095=PLANE ( 'NONE',  #214094 ) ;
#161099=AXIS2_PLACEMENT_3D ( 'NONE', #148896, #468, #132679 ) ;
#161108=CARTESIAN_POINT ( 'NONE',  ( -0.004084902416449302624, 15.44286970158244721, 11.94689474181819122 ) ) ;
#161129=CARTESIAN_POINT ( 'NONE',  ( 7.219375133607416117, 15.46908217912056038, -9.592069343535143844 ) ) ;
#161155=CARTESIAN_POINT ( 'NONE',  ( -9.707245187965476418, 5.109025436760802563, -6.475459982491707400 ) ) ;
#161165=CARTESIAN_POINT ( 'NONE',  ( -11.44791656467458374, 12.29999999999998650, 3.303228920649577294 ) ) ;
#161180=CARTESIAN_POINT ( 'NONE',  ( 10.90672086898367077, 10.32844188227105953, 5.068303158999801994 ) ) ;
#161188=FILL_AREA_STYLE_COLOUR ( '', #144728 ) ;
#161205=FACE_OUTER_BOUND ( 'NONE', #56684, .T. ) ;
#161223=( NAMED_UNIT ( * ) PLANE_ANGLE_UNIT ( ) SI_UNIT ( $, .RADIAN. ) );
#161234=CARTESIAN_POINT ( 'NONE',  ( -15.75000000000000000, 13.40000000000000036, -1.100000000000002087 ) ) ;
#161238=VECTOR ( 'NONE', #193929, 1000.000000000000000 ) ;
#161246=AXIS2_PLACEMENT_3D ( 'NONE', #188477, #120358, #186336 ) ;
#161266=DIRECTION ( 'NONE',  ( 1.000000000000000000, 0.000000000000000000, 0.000000000000000000 ) ) ;
#161282=EDGE_CURVE ( 'NONE', #191009, #58680, #79642, .T. ) ;
#161297=( LENGTH_UNIT ( ) NAMED_UNIT ( * ) SI_UNIT ( .MILLI., .METRE. ) );
#161299=CARTESIAN_POINT ( 'NONE',  ( 11.43209210103587914, 13.65596075983914659, 3.649125173352119944 ) ) ;
#161302=CARTESIAN_POINT ( 'NONE',  ( 11.55950211276791251, 9.719999999999982876, 3.221476510067110777 ) ) ;
#161306=DIRECTION ( 'NONE',  ( -0.000000000000000000, -1.000000000000000000, -0.000000000000000000 ) ) ;
#161323=CARTESIAN_POINT ( 'NONE',  ( -9.497986837693062512, 14.58017599252426066, 7.334206418178426112 ) ) ;
#161331=CARTESIAN_POINT ( 'NONE',  ( 11.97929049433705373, 12.22000000000000064, -0.7046979865771834106 ) ) ;
#161340=UNCERTAINTY_MEASURE_WITH_UNIT (LENGTH_MEASURE( 1.000000000000000082E-05 ), #71720, 'distance_accuracy_value', 'NONE');
#161351=EDGE_LOOP ( 'NONE', ( #175279, #97977, #201005, #1554, #174041, #33826, #200573, #205357 ) ) ;
#161355=ORIENTED_EDGE ( 'NONE', *, *, #56757, .F. ) ;
#161365=AXIS2_PLACEMENT_3D ( 'NONE', #8752, #5519, #171251 ) ;
#161366=CARTESIAN_POINT ( 'NONE',  ( -11.94105721237523099, 12.69999999999999929, 1.187919463087248273 ) ) ;
#161421=CARTESIAN_POINT ( 'NONE',  ( 11.41381675112453031, 12.69999999999999929, -3.704697986577182078 ) ) ;
#161436=CARTESIAN_POINT ( 'NONE',  ( 1.474414414893455261, 7.826756755319739689, 10.64843978026285320 ) ) ;
#161440=( LENGTH_UNIT ( ) NAMED_UNIT ( * ) SI_UNIT ( .MILLI., .METRE. ) );
#161456=FILL_AREA_STYLE_COLOUR ( '', #175175 ) ;
#161461=CARTESIAN_POINT ( 'NONE',  ( -11.84103413958613160, 13.61004478473142676, -1.443924719788764799 ) ) ;
#161504=DIRECTION ( 'NONE',  ( -0.000000000000000000, -1.000000000000000000, -0.000000000000000000 ) ) ;
#161525=CARTESIAN_POINT ( 'NONE',  ( 8.730309718301390021, 13.52954257607862942, 8.166533740197252200 ) ) ;
#161527=ORIENTED_EDGE ( 'NONE', *, *, #12290, .F. ) ;
#161541=CARTESIAN_POINT ( 'NONE',  ( 11.52460864928264783, 12.21999999999998110, 3.346683403123522638 ) ) ;
#161558=CIRCLE ( 'NONE', #67955, 0.07999999999999998779 ) ;
#161587=COLOUR_RGB ( '', 0.08235294, 0.09019608, 0.10196078) ;
#161591=FACE_OUTER_BOUND ( 'NONE', #79267, .T. ) ;
#161627=ORIENTED_EDGE ( 'NONE', *, *, #189888, .T. ) ;
#161657=CARTESIAN_POINT ( 'NONE',  ( -9.702943487419032564, 4.518467169708416442, -7.062559895321285808 ) ) ;
#161664=B_SPLINE_CURVE_WITH_KNOTS ( 'NONE', 3,
 ( #118822, #72125, #184809, #151276, #36438, #204246 ),
 .UNSPECIFIED., .F., .F.,
 ( 4, 2, 4 ),
 ( 0.000000000000000000, 0.0003767643964918265939, 0.0007535287929836531878 ),
 .UNSPECIFIED. ) ;
#161676=ORIENTED_EDGE ( 'NONE', *, *, #166530, .F. ) ;
#161724=CARTESIAN_POINT ( 'NONE',  ( 10.42279406580779444, 10.52049161362584684, -5.955436901484764789 ) ) ;
#161727=COLOUR_RGB ( '', 0.66274510, 0.83137255, 0.94901961) ;
#161732=EDGE_CURVE ( 'NONE', #73245, #108056, #49332, .T. ) ;
#161743=CARTESIAN_POINT ( 'NONE',  ( 10.88220342306020072, 9.708224249340068113, -7.303426440398375519 ) ) ;
#161745=VERTEX_POINT ( 'NONE', #19995 ) ;
#161747=EDGE_LOOP ( 'NONE', ( #7149, #110890, #146985, #122007 ) ) ;
#161760=CARTESIAN_POINT ( 'NONE',  ( 11.78331023100045627, 12.30000000000000071, -1.800000000000001155 ) ) ;
#161795=CARTESIAN_POINT ( 'NONE',  ( -11.51804212353614609, 7.080072447566390537, 3.210211610704029717 ) ) ;
#161821=EDGE_CURVE ( 'NONE', #45616, #72859, #13900, .T. ) ;
#161826=VECTOR ( 'NONE', #24258, 1000.000000000000000 ) ;
#161841=CARTESIAN_POINT ( 'NONE',  ( -10.96648295346442126, 6.136757939018690600, -4.903056198141964472 ) ) ;
#161845=CARTESIAN_POINT ( 'NONE',  ( 9.177312029184088615, 14.07967752687478757, -6.957318393903204168 ) ) ;
#161848=CARTESIAN_POINT ( 'NONE',  ( 7.441609955141260002, 14.00158514652465591, 10.27059997516222190 ) ) ;
#161856=CARTESIAN_POINT ( 'NONE',  ( -11.33772463945036968, 10.90000000000000036, -3.600000000000002309 ) ) ;
#161866=CARTESIAN_POINT ( 'NONE',  ( -10.28478851095648849, 4.808147343396361961, -6.103030503883996261 ) ) ;
#161881=CARTESIAN_POINT ( 'NONE',  ( -11.50450067106337571, 6.429220943216678030, -3.050492100467481205 ) ) ;
#161907=CARTESIAN_POINT ( 'NONE',  ( 11.97450891632845327, 7.629227029099267199, 0.8948425641056547697 ) ) ;
#161955=CARTESIAN_POINT ( 'NONE',  ( -11.77541522617479508, 7.697538928213582210, 2.075964864015985345 ) ) ;
#161956=EDGE_CURVE ( 'NONE', #115502, #199511, #128140, .T. ) ;
#161964=CARTESIAN_POINT ( 'NONE',  ( -10.66277494340078746, 5.899681303200420501, -5.512943113908496784 ) ) ;
#161979=ORIENTED_EDGE ( 'NONE', *, *, #3283, .F. ) ;
#161988=CARTESIAN_POINT ( 'NONE',  ( 10.62873463776380056, 9.799999999999998934, -3.200000000000001510 ) ) ;
#161995=CARTESIAN_POINT ( 'NONE',  ( -12.40359606095370992, 6.583381993447835256, -3.463844519762692364 ) ) ;
#162014=CARTESIAN_POINT ( 'NONE',  ( -11.87815913191726480, 12.29692179368583282, 1.708869976696563819 ) ) ;
#162016=CARTESIAN_POINT ( 'NONE',  ( 11.33772465723203915, 13.50868300734825844, -3.600000000000076472 ) ) ;
#162033=CARTESIAN_POINT ( 'NONE',  ( 9.601932014265653237, 4.115787152683171080, 7.121345992675207626 ) ) ;
#162058=CARTESIAN_POINT ( 'NONE',  ( 0.005768037945334394262, 14.55305234682519533, 11.95586101163397963 ) ) ;
#162068=ORIENTED_EDGE ( 'NONE', *, *, #198514, .F. ) ;
#162075=ADVANCED_FACE ( 'NONE', ( #136977 ), #201925, .F. ) ;
#162083=DIRECTION ( 'NONE',  ( -0.000000000000000000, -1.000000000000000000, -0.000000000000000000 ) ) ;
#162091=EDGE_CURVE ( 'NONE', #96092, #96576, #177177, .T. ) ;
#162128=DIRECTION ( 'NONE',  ( -0.000000000000000000, -1.000000000000000000, -0.000000000000000000 ) ) ;
#162137=ADVANCED_FACE ( 'NONE', ( #26406 ), #117744, .T. ) ;
#162157=ORIENTED_EDGE ( 'NONE', *, *, #109604, .T. ) ;
#162162=SURFACE_STYLE_USAGE ( .BOTH. , #79823 ) ;
#162165=MECHANICAL_DESIGN_GEOMETRIC_PRESENTATION_REPRESENTATION('',(#103387),#127616);
#162166=CARTESIAN_POINT ( 'NONE',  ( -10.41415007634638989, 5.040604921122249671, 5.873056126304751601 ) ) ;
#162182=CARTESIAN_POINT ( 'NONE',  ( -10.50059885609813115, 5.377696206510352184, -5.808392519734754345 ) ) ;
#162226=CARTESIAN_POINT ( 'NONE',  ( -11.00592740523952351, 11.11020242468316788, 1.444008943503716225 ) ) ;
#162227=CARTESIAN_POINT ( 'NONE',  ( -9.979823206198361163, 5.589814398814591634, -5.978750339097100408 ) ) ;
#162232=CARTESIAN_POINT ( 'NONE',  ( -10.50000000000000000, 10.19999999999999929, -3.600000000000000977 ) ) ;
#162240=CARTESIAN_POINT ( 'NONE',  ( 6.928203230275524760, 14.48154074412737202, -9.797958971132702644 ) ) ;
#162247=DIRECTION ( 'NONE',  ( 0.000000000000000000, 0.000000000000000000, -1.000000000000000000 ) ) ;
#162248=CARTESIAN_POINT ( 'NONE',  ( 12.00693267275518572, 8.237831693621128437, -3.583085096157309302 ) ) ;
#162249=CARTESIAN_POINT ( 'NONE',  ( -10.43230948805442893, 5.066484524551064794, 5.254757398418679060 ) ) ;
#162253=VECTOR ( 'NONE', #29399, 1000.000000000000000 ) ;
#162273=CARTESIAN_POINT ( 'NONE',  ( -11.86145016429273014, 10.19999999999999929, -1.100000000000000311 ) ) ;
#162275=PRESENTATION_STYLE_ASSIGNMENT (( #196892 ) ) ;
#162279=CARTESIAN_POINT ( 'NONE',  ( -10.41986968326957808, 5.020773655391575829, -5.279272669861445166 ) ) ;
#162290=CARTESIAN_POINT ( 'NONE',  ( -9.386220697865741869, 15.51845925627288203, -7.476614105868906179 ) ) ;
#162299=STYLED_ITEM ( 'NONE', ( #37465 ), #22947 ) ;
#162305=FILL_AREA_STYLE ('',( #48559 ) ) ;
#162317=COLOUR_RGB ( '', 0.08235294, 0.09019608, 0.10196078) ;
#162350=UNCERTAINTY_MEASURE_WITH_UNIT (LENGTH_MEASURE( 1.000000000000000082E-05 ), #46512, 'distance_accuracy_value', 'NONE');
#162369=CARTESIAN_POINT ( 'NONE',  ( 11.41381675112453564, 13.53005666089991443, 3.704697986577181190 ) ) ;
#162372=CARTESIAN_POINT ( 'NONE',  ( -15.75000000000000000, 13.40000000000000036, 1.099999999999996758 ) ) ;
#162395=( NAMED_UNIT ( * ) SI_UNIT ( $, .STERADIAN. ) SOLID_ANGLE_UNIT ( ) );
#162402=CARTESIAN_POINT ( 'NONE',  ( 0.001355176523862845501, 14.56276549857873093, 11.93721147252166048 ) ) ;
#162409=CARTESIAN_POINT ( 'NONE',  ( -9.569358774130435563, 3.553060279300347180, -7.167287524826059020 ) ) ;
#162420=DIRECTION ( 'NONE',  ( -0.000000000000000000, -1.000000000000000000, -0.000000000000000000 ) ) ;
#162441=DIRECTION ( 'NONE',  ( 0.2684563758389304500, 5.821219718043054220E-15, 0.9632918427306581544 ) ) ;
#162460=CARTESIAN_POINT ( 'NONE',  ( 8.753616243065934555, 13.39305056715447861, 8.208245953058789013 ) ) ;
#162500=ORIENTED_EDGE ( 'NONE', *, *, #170541, .F. ) ;
#162506=DIRECTION ( 'NONE',  ( 0.000000000000000000, 1.000000000000000000, 0.000000000000000000 ) ) ;
#162524=DIRECTION ( 'NONE',  ( -0.05872483221476459958, -0.000000000000000000, -0.9982742078614211811 ) ) ;
#162533=SURFACE_SIDE_STYLE ('',( #100705 ) ) ;
#162549=DIRECTION ( 'NONE',  ( -0.05872483221476467591, 7.952201780260630618E-17, -0.9982742078614211811 ) ) ;
#162588=EDGE_LOOP ( 'NONE', ( #99669, #201664, #30105, #42464 ) ) ;
#162594=CARTESIAN_POINT ( 'NONE',  ( -10.50059885609814536, 5.377696206510357513, -5.808392519734771220 ) ) ;
#162603=CARTESIAN_POINT ( 'NONE',  ( 11.43204722947019825, 12.44407245973824239, 3.649275849833181429 ) ) ;
#162605=CARTESIAN_POINT ( 'NONE',  ( 0.000000000000000000, 11.37999999999999901, 0.000000000000000000 ) ) ;
#162612=CARTESIAN_POINT ( 'NONE',  ( 11.89942855770814312, 13.79999999999999893, 0.6999999999999992895 ) ) ;
#162616=EDGE_CURVE ( 'NONE', #7772, #72818, #56024, .T. ) ;
#162627=( LENGTH_UNIT ( ) NAMED_UNIT ( * ) SI_UNIT ( .MILLI., .METRE. ) );
#162633=VECTOR ( 'NONE', #188982, 1000.000000000000000 ) ;
#162639=EDGE_LOOP ( 'NONE', ( #91133, #79110, #24243, #154493 ) ) ;
#162705=CARTESIAN_POINT ( 'NONE',  ( -11.33772463945036968, 10.90000000000000036, -3.600000000000002309 ) ) ;
#162722=CARTESIAN_POINT ( 'NONE',  ( 11.44779964734654598, 10.99810470129597917, -3.599999963171534478 ) ) ;
#162751=CARTESIAN_POINT ( 'NONE',  ( 11.97929049433705373, 13.88000000000000078, 0.7046979865771783036 ) ) ;
#162753=CARTESIAN_POINT ( 'NONE',  ( 11.89942855770814312, 11.29999999999999893, -0.7000000000000009548 ) ) ;
#162756=VERTEX_POINT ( 'NONE', #118950 ) ;
#162798=SURFACE_SIDE_STYLE ('',( #46922 ) ) ;
#162809=CARTESIAN_POINT ( 'NONE',  ( 13.13868652300558715, 6.588164048981460574, -1.077943021382721245 ) ) ;
#162813=EDGE_LOOP ( 'NONE', ( #181970, #202290, #138289, #13244 ) ) ;
#162815=EDGE_LOOP ( 'NONE', ( #32769, #20881, #187568, #160826 ) ) ;
#162820=CARTESIAN_POINT ( 'NONE',  ( 10.97030176249251099, 9.799999999999982947, 1.695215491223429183 ) ) ;
#162836=AXIS2_PLACEMENT_3D ( 'NONE', #39248, #120580, #188696 ) ;
#162839=CARTESIAN_POINT ( 'NONE',  ( -11.97929049433705373, 11.37999999999999901, -0.7046979865771821894 ) ) ;
#162902=CARTESIAN_POINT ( 'NONE',  ( -11.30177626766236365, 6.974151656887320527, -4.150880038395990290 ) ) ;
#162906=CARTESIAN_POINT ( 'NONE',  ( 9.673880494682652653, 13.47554395514287684, -8.174421919205036247 ) ) ;
#162909=CARTESIAN_POINT ( 'NONE',  ( 9.143844951682952527, 13.34121998047297808, 9.071981315083665010 ) ) ;
#162916=ADVANCED_FACE ( 'NONE', ( #143443 ), #110965, .T. ) ;
#162942=CARTESIAN_POINT ( 'NONE',  ( -10.96041802301306944, 4.843384909922287207, -4.379099270644332798 ) ) ;
#162957=DIRECTION ( 'NONE',  ( 0.000000000000000000, 1.000000000000000000, 0.000000000000000000 ) ) ;
#162970=CARTESIAN_POINT ( 'NONE',  ( 11.80845508765946050, 7.960079180001382149, 2.175004853915265546 ) ) ;
#162976=VECTOR ( 'NONE', #116468, 1000.000000000000000 ) ;
#163018=CARTESIAN_POINT ( 'NONE',  ( -11.50347174040005527, 6.904995786113715006, 3.422550450347928486 ) ) ;
#163044=EDGE_CURVE ( 'NONE', #93441, #60282, #149056, .T. ) ;
#163060=CARTESIAN_POINT ( 'NONE',  ( -11.82196040793749425, 4.889518425415825931, 4.884593937341564107 ) ) ;
#163079=CARTESIAN_POINT ( 'NONE',  ( -11.91826849282518630, 12.69999999999997975, 1.399999999999996581 ) ) ;
#163083=CARTESIAN_POINT ( 'NONE',  ( 9.243799147819517614, 13.41009114453062345, -7.924839666318222342 ) ) ;
#163089=CARTESIAN_POINT ( 'NONE',  ( -3.535343422797964763, 15.44796817926509291, 11.42948407163687286 ) ) ;
#163100=CARTESIAN_POINT ( 'NONE',  ( 9.651540038386141163, 3.878167290971874959, 7.130941910101068260 ) ) ;
#163109=EDGE_LOOP ( 'NONE', ( #40844, #187682, #46798, #165172 ) ) ;
#163115=CARTESIAN_POINT ( 'NONE',  ( -15.75000000000000000, 12.30000000000000071, -3.200000000000001510 ) ) ;
#163119=DIRECTION ( 'NONE',  ( 0.000000000000000000, 0.000000000000000000, -1.000000000000000000 ) ) ;
#163121=LINE ( 'NONE', #92801, #18689 ) ;
#163136=DIRECTION ( 'NONE',  ( 1.000000000000000000, 0.000000000000000000, -0.000000000000000000 ) ) ;
#163138=CIRCLE ( 'NONE', #170066, 0.5000000000000005551 ) ;
#163166=SURFACE_STYLE_FILL_AREA ( #113412 ) ;
#163185=( GEOMETRIC_REPRESENTATION_CONTEXT ( 3 ) GLOBAL_UNCERTAINTY_ASSIGNED_CONTEXT ( ( #78181 ) ) GLOBAL_UNIT_ASSIGNED_CONTEXT ( ( #23589, #53975, #171997 ) ) REPRESENTATION_CONTEXT ( 'NONE', 'WORKASPACE' ) );
#163206=CARTESIAN_POINT ( 'NONE',  ( 0.000000000000000000, 11.37999999999999901, 0.000000000000000000 ) ) ;
#163230=CARTESIAN_POINT ( 'NONE',  ( 10.51582573219069694, 12.48709141521726984, 3.554376768052132540 ) ) ;
#163234=CARTESIAN_POINT ( 'NONE',  ( -0.08053691275167716712, 15.51846456562902965, 11.99972973886013961 ) ) ;
#163236=CARTESIAN_POINT ( 'NONE',  ( 9.333041836208478159, 3.553060279300227275, -7.472413793088525935 ) ) ;
#163263=CARTESIAN_POINT ( 'NONE',  ( 8.929730105901844794, 14.71341541692550514, -8.017539274085800471 ) ) ;
#163273=( GEOMETRIC_REPRESENTATION_CONTEXT ( 3 ) GLOBAL_UNCERTAINTY_ASSIGNED_CONTEXT ( ( #67796 ) ) GLOBAL_UNIT_ASSIGNED_CONTEXT ( ( #49934, #100805, #98692 ) ) REPRESENTATION_CONTEXT ( 'NONE', 'WORKASPACE' ) );
#163282=EDGE_CURVE ( 'NONE', #138322, #48473, #72823, .T. ) ;
#163302=CARTESIAN_POINT ( 'NONE',  ( 8.790438134619867228, 13.29428800202396133, -8.101059483297383679 ) ) ;
#163308=ORIENTED_EDGE ( 'NONE', *, *, #193079, .F. ) ;
#163310=SURFACE_STYLE_FILL_AREA ( #97256 ) ;
#163311=CARTESIAN_POINT ( 'NONE',  ( 12.43511541931632891, 7.569548269842172772, -1.878403980710225518 ) ) ;
#163314=VERTEX_POINT ( 'NONE', #132525 ) ;
#163325=EDGE_LOOP ( 'NONE', ( #196316, #44069, #207086, #197486 ) ) ;
#163369=CARTESIAN_POINT ( 'NONE',  ( -9.604686356149279902, 3.481548657788669843, -7.193747284969073341 ) ) ;
#163386=PRESENTATION_STYLE_ASSIGNMENT (( #31255 ) ) ;
#163445=LINE ( 'NONE', #165564, #174434 ) ;
#163457=EDGE_CURVE ( 'NONE', #198860, #120109, #133074, .T. ) ;
#163458=CARTESIAN_POINT ( 'NONE',  ( -9.439063866441687267, 15.48793654326890490, 7.409881740265291228 ) ) ;
#163490=ADVANCED_FACE ( 'NONE', ( #115233 ), #7794, .F. ) ;
#163521=CARTESIAN_POINT ( 'NONE',  ( 8.202753408314407579, 14.20975653142720319, 8.698399028645537712 ) ) ;
#163545=CARTESIAN_POINT ( 'NONE',  ( 11.44786932348528907, 12.30000000000000071, -3.303370173849653035 ) ) ;
#163546=CARTESIAN_POINT ( 'NONE',  ( 0.000000000000000000, 7.980384757729337863, 0.000000000000000000 ) ) ;
#163582=DIRECTION ( 'NONE',  ( 1.000000000000000000, -0.000000000000000000, -0.000000000000000000 ) ) ;
#163584=CARTESIAN_POINT ( 'NONE',  ( -9.356550365033111660, 14.56579225990834736, 7.432331899221528815 ) ) ;
#163612=CARTESIAN_POINT ( 'NONE',  ( -11.52515587343483539, 8.148303942382858267, 3.187149427615555197 ) ) ;
#163682=CARTESIAN_POINT ( 'NONE',  ( -11.86145016429273014, 13.40000000000000036, -1.100000000000000533 ) ) ;
#163694=CARTESIAN_POINT ( 'NONE',  ( -10.50000000000000000, 10.19999999999998153, 3.599999999999999201 ) ) ;
#163702=STYLED_ITEM ( 'NONE', ( #163386 ), #111806 ) ;
#163720=CIRCLE ( 'NONE', #59951, 11.09999999999999964 ) ;
#163726=CARTESIAN_POINT ( 'NONE',  ( 11.48243876534946217, 13.79999999999999893, -3.200000000000001510 ) ) ;
#163756=ADVANCED_FACE ( 'NONE', ( #13691 ), #50465, .F. ) ;
#163784=CARTESIAN_POINT ( 'NONE',  ( -11.86145016429273191, 13.40000000000000036, 1.099999999999996758 ) ) ;
#163809=DIRECTION ( 'NONE',  ( -0.5773502691896238437, 0.000000000000000000, 0.8164965809277274778 ) ) ;
#163814=FACE_OUTER_BOUND ( 'NONE', #129297, .T. ) ;
#163821=B_SPLINE_CURVE_WITH_KNOTS ( 'NONE', 3,
 ( #23509, #205462, #74418, #43003, #76533, #174073 ),
 .UNSPECIFIED., .F., .F.,
 ( 4, 2, 4 ),
 ( 0.000000000000000000, 0.0003239988925529258120, 0.0006479977851058516241 ),
 .UNSPECIFIED. ) ;
#163825=VERTEX_POINT ( 'NONE', #182579 ) ;
#163845=EDGE_CURVE ( 'NONE', #213513, #175384, #50169, .T. ) ;
#163847=ORIENTED_EDGE ( 'NONE', *, *, #120283, .T. ) ;
#163878=CARTESIAN_POINT ( 'NONE',  ( 9.704905176613070950, 13.32621205788646002, -8.135614888031417635 ) ) ;
#163891=LINE ( 'NONE', #145539, #139313 ) ;
#163917=CARTESIAN_POINT ( 'NONE',  ( 11.48243876534946217, 9.799999999999998934, -3.200000000000001510 ) ) ;
#163929=CARTESIAN_POINT ( 'NONE',  ( -11.63140583992382560, 7.361097535320459961, -2.771579487483898596 ) ) ;
#163938=CARTESIAN_POINT ( 'NONE',  ( -11.78331023100045627, 11.29999999999998117, 1.799999999999999600 ) ) ;
#163975=CARTESIAN_POINT ( 'NONE',  ( 8.736508494932113678, 15.13472907373737186, -7.593571698007603565 ) ) ;
#164007=CARTESIAN_POINT ( 'NONE',  ( -11.13243988973272636, 5.430794512910079419, -4.010128837087161280 ) ) ;
#164031=ORIENTED_EDGE ( 'NONE', *, *, #188144, .T. ) ;
#164042=DIRECTION ( 'NONE',  ( 0.000000000000000000, 1.000000000000000000, 0.000000000000000000 ) ) ;
#164050=CARTESIAN_POINT ( 'NONE',  ( 11.84668730067608600, 10.19999999999999929, -1.400000000000001910 ) ) ;
#164065=DIRECTION ( 'NONE',  ( 0.000000000000000000, 0.000000000000000000, 1.000000000000000000 ) ) ;
#164071=CARTESIAN_POINT ( 'NONE',  ( 0.000000000000000000, 4.518467169708413778, 0.000000000000000000 ) ) ;
#164081=CYLINDRICAL_SURFACE ( 'NONE', #167749, 0.3999999999999997446 ) ;
#164085=CARTESIAN_POINT ( 'NONE',  ( -11.86402016121722269, 7.774204713095177688, -1.819606832628274384 ) ) ;
#164093=CARTESIAN_POINT ( 'NONE',  ( -11.56582117199599224, 8.167499266818545323, -3.209445363707945198 ) ) ;
#164098=ORIENTED_EDGE ( 'NONE', *, *, #82220, .T. ) ;
#164103=EDGE_LOOP ( 'NONE', ( #52968, #82993, #171181, #134809 ) ) ;
#164124=DIRECTION ( 'NONE',  ( 0.000000000000000000, 0.000000000000000000, -1.000000000000000000 ) ) ;
#164167=ORIENTED_EDGE ( 'NONE', *, *, #91785, .F. ) ;
#164169=VECTOR ( 'NONE', #211379, 1000.000000000000000 ) ;
#164196=CARTESIAN_POINT ( 'NONE',  ( -15.75000000000000000, 10.90000000000000036, -3.600000000000002309 ) ) ;
#164223=DIRECTION ( 'NONE',  ( 0.000000000000000000, 1.000000000000000000, 0.000000000000000000 ) ) ;
#164225=UNCERTAINTY_MEASURE_WITH_UNIT (LENGTH_MEASURE( 1.000000000000000082E-05 ), #31959, 'distance_accuracy_value', 'NONE');
#164248=CARTESIAN_POINT ( 'NONE',  ( 11.43209210103587914, 9.944039240160840620, -3.649125173352125273 ) ) ;
#164281=( NAMED_UNIT ( * ) PLANE_ANGLE_UNIT ( ) SI_UNIT ( $, .RADIAN. ) );
#164316=CARTESIAN_POINT ( 'NONE',  ( 11.86685672517501899, 9.990810821401886699, -1.056525322636012065 ) ) ;
#164324=LINE ( 'NONE', #197872, #208966 ) ;
#164332=( BOUNDED_SURFACE ( )  B_SPLINE_SURFACE ( 3, 2, ( 
 ( #196583, #80706, #129539 ),
 ( #61247, #161964, #195520 ),
 ( #113273, #130594, #13555 ),
 ( #62316, #11416, #128475 ),
 ( #47157, #143610, #213861 ),
 ( #131631, #210688, #48226 ),
 ( #81761, #178211, #28752 ),
 ( #179278, #164093, #145745 ),
 ( #197630, #96978, #15674 ),
 ( #79626, #209603, #49275 ),
 ( #211746, #30902, #114338 ),
 ( #12482, #180333, #194443 ),
 ( #127404, #46085, #146796 ),
 ( #78556, #29827, #115396 ),
 ( #212812, #181389, #144674 ),
 ( #112204, #95910, #94836 ),
 ( #31956, #45021, #64449 ),
 ( #193377, #98040, #33012 ),
 ( #177135, #152099, #2611 ),
 ( #66538, #18869, #182442 ),
 ( #69746, #3670, #199757 ),
 ( #52460, #169407, #87089 ),
 ( #68680, #67603, #183516 ),
 ( #135852, #168344, #84953 ),
 ( #86025, #153159, #4734 ),
 ( #201874, #134804, #185641 ),
 ( #133749, #198685, #36193 ),
 ( #200810, #118586, #83881 ) ),
 .UNSPECIFIED., .F., .F., .F. ) 
 B_SPLINE_SURFACE_WITH_KNOTS ( ( 4, 2, 2, 2, 2, 2, 2, 2, 2, 2, 2, 2, 2, 4 ),
 ( 3, 3 ),
 ( 8.673617379884035472E-19, 0.001863568725704640170, 0.002795353088556959929, 0.003727137451409279472, 0.004658921814261599015, 0.005590706177113918991, 0.007454274902818558077, 0.008386059265670878921, 0.009317843628523198030, 0.01024962799137551714, 0.01118141235422783625, 0.01211319671708015536, 0.01304498107993247620, 0.01490854980563711615 ),
 ( 0.000000000000000000, 1.000000000000000000 ),
 .UNSPECIFIED. ) 
 GEOMETRIC_REPRESENTATION_ITEM ( )  RATIONAL_B_SPLINE_SURFACE ( (
 ( 1.000000000000000000, 0.8462382765735652068, 1.000000000000000000),
 ( 1.000000000000000000, 0.8465420404195402870, 1.000000000000000000),
 ( 1.000000000000000000, 0.8466805660004343981, 1.000000000000000000),
 ( 1.000000000000000000, 0.8469123506191252870, 1.000000000000000000),
 ( 1.000000000000000000, 0.8470220173784553941, 1.000000000000000000),
 ( 1.000000000000000000, 0.8471957003534210662, 1.000000000000000000),
 ( 1.000000000000000000, 0.8472535244121295328, 1.000000000000000000),
 ( 1.000000000000000000, 0.8472797654243715559, 1.000000000000000000),
 ( 1.000000000000000000, 0.8469106832326384060, 1.000000000000000000),
 ( 1.000000000000000000, 0.8463026754876442626, 1.000000000000000000),
 ( 1.000000000000000000, 0.8460620800516406304, 1.000000000000000000),
 ( 1.000000000000000000, 0.8460269503523500934, 1.000000000000000000),
 ( 1.000000000000000000, 0.8472022497197664315, 1.000000000000000000),
 ( 1.000000000000000000, 0.8472231902808619042, 1.000000000000000000),
 ( 1.000000000000000000, 0.8468169758819515947, 1.000000000000000000),
 ( 1.000000000000000000, 0.8461442878182255933, 1.000000000000000000),
 ( 1.000000000000000000, 0.8458919886175331193, 1.000000000000000000),
 ( 1.000000000000000000, 0.8458966812448689421, 1.000000000000000000),
 ( 1.000000000000000000, 0.8461525964263839628, 1.000000000000000000),
 ( 1.000000000000000000, 0.8468439809311968380, 1.000000000000000000),
 ( 1.000000000000000000, 0.8472723393077549181, 1.000000000000000000),
 ( 1.000000000000000000, 0.8472611234995456320, 1.000000000000000000),
 ( 1.000000000000000000, 0.8471603390332783645, 1.000000000000000000),
 ( 1.000000000000000000, 0.8469206950638731302, 1.000000000000000000),
 ( 1.000000000000000000, 0.8467815351080468789, 1.000000000000000000),
 ( 1.000000000000000000, 0.8465568167268769928, 1.000000000000000000),
 ( 1.000000000000000000, 0.8465337723686136018, 1.000000000000000000),
 ( 1.000000000000000000, 0.8462384754710241541, 1.000000000000000000) ) ) 
 REPRESENTATION_ITEM ( '' )  SURFACE ( )  );
#164335=AXIS2_PLACEMENT_3D ( 'NONE', #119408, #150795, #99900 ) ;
#164337=ORIENTED_EDGE ( 'NONE', *, *, #54609, .T. ) ;
#164340=EDGE_LOOP ( 'NONE', ( #8626, #164899, #91322, #60976 ) ) ;
#164348=CARTESIAN_POINT ( 'NONE',  ( -9.912197829101469182, 5.385002637010017246, -6.113573717307969169 ) ) ;
#164353=CIRCLE ( 'NONE', #143535, 11.92000000000000171 ) ;
#164364=CARTESIAN_POINT ( 'NONE',  ( 8.810048391696772896, 13.28851571758704253, -8.147727092588480602 ) ) ;
#164373=CARTESIAN_POINT ( 'NONE',  ( 8.831150071590936790, 13.23551488323715830, -7.656846099933870775 ) ) ;
#164392=EDGE_CURVE ( 'NONE', #116972, #55552, #127753, .T. ) ;
#164408=VERTEX_POINT ( 'NONE', #94597 ) ;
#164477=DIRECTION ( 'NONE',  ( -0.000000000000000000, -1.000000000000000000, 0.000000000000000000 ) ) ;
#164554=EDGE_CURVE ( 'NONE', #37173, #66261, #93530, .T. ) ;
#164578=CARTESIAN_POINT ( 'NONE',  ( 8.568388180517228392, 13.84533258836909475, 8.337145738167963671 ) ) ;
#164604=DIRECTION ( 'NONE',  ( 0.000000000000000000, -1.000000000000000000, 0.000000000000000000 ) ) ;
#164619=CARTESIAN_POINT ( 'NONE',  ( 11.80235830595198543, 9.799999999999998934, -1.696088231482801856 ) ) ;
#164635=SURFACE_STYLE_FILL_AREA ( #197125 ) ;
#164659=DIRECTION ( 'NONE',  ( -0.000000000000000000, -1.000000000000000000, -0.000000000000000000 ) ) ;
#164668=( LENGTH_UNIT ( ) NAMED_UNIT ( * ) SI_UNIT ( .MILLI., .METRE. ) );
#164719=CARTESIAN_POINT ( 'NONE',  ( -11.55950211276791251, 12.22000000000000064, -3.221476510067115662 ) ) ;
#164730=DIRECTION ( 'NONE',  ( -0.000000000000000000, 1.000000000000000000, 0.000000000000000000 ) ) ;
#164743=SURFACE_STYLE_FILL_AREA ( #113942 ) ;
#164751=AXIS2_PLACEMENT_3D ( 'NONE', #55376, #204795, #174485 ) ;
#164771=CARTESIAN_POINT ( 'NONE',  ( 11.89197369110779334, 12.30000000000000249, 0.8056055387119843703 ) ) ;
#164779=CARTESIAN_POINT ( 'NONE',  ( -9.429696025003076798, 5.003427382976973981, 6.891771494149568689 ) ) ;
#164794=AXIS2_PLACEMENT_3D ( 'NONE', #133498, #117269, #199501 ) ;
#164810=CARTESIAN_POINT ( 'NONE',  ( -9.417646481058939756, 15.36155943915161259, -7.338279069507036567 ) ) ;
#164824=ADVANCED_FACE ( 'NONE', ( #199516 ), #67082, .T. ) ;
#164837=CARTESIAN_POINT ( 'NONE',  ( 11.55950211276791251, 11.29999999999999893, -3.221476510067115662 ) ) ;
#164842=DIRECTION ( 'NONE',  ( 0.000000000000000000, 0.000000000000000000, 1.000000000000000000 ) ) ;
#164852=CARTESIAN_POINT ( 'NONE',  ( -0.07999999999999847511, 19.00000000000000000, 11.91973154060107376 ) ) ;
#164864=ORIENTED_EDGE ( 'NONE', *, *, #95230, .F. ) ;
#164871=EDGE_LOOP ( 'NONE', ( #80479, #83218, #12213, #143773 ) ) ;
#164895=EDGE_LOOP ( 'NONE', ( #195186, #179536, #133683, #93552 ) ) ;
#164899=ORIENTED_EDGE ( 'NONE', *, *, #82708, .F. ) ;
#164901=FACE_OUTER_BOUND ( 'NONE', #170836, .T. ) ;
#164904=CARTESIAN_POINT ( 'NONE',  ( -11.86239285000045918, 9.719999999999998863, -1.812080536912753059 ) ) ;
#164910=AXIS2_PLACEMENT_3D ( 'NONE', #53062, #201423, #183064 ) ;
#164922=CARTESIAN_POINT ( 'NONE',  ( 12.05321605296785492, 8.347302252938671785, -5.364299177381870898 ) ) ;
#164995=ORIENTED_EDGE ( 'NONE', *, *, #143394, .F. ) ;
#165022=CARTESIAN_POINT ( 'NONE',  ( 8.399998182892758791, 14.34039879828830522, -8.119840057749129869 ) ) ;
#165044=CARTESIAN_POINT ( 'NONE',  ( 11.87828357749917529, 13.80310252740378907, -1.708055325888794496 ) ) ;
#165060=CARTESIAN_POINT ( 'NONE',  ( 9.277806814877628483, 13.85436241318128125, -7.538798676216699413 ) ) ;
#165086=CARTESIAN_POINT ( 'NONE',  ( 9.397879144821104092, 13.53129603721547447, -7.462055881301289162 ) ) ;
#165099=CARTESIAN_POINT ( 'NONE',  ( 11.89839339040395316, 12.27122531596078403, -1.560885614203536997 ) ) ;
#165120=DIRECTION ( 'NONE',  ( 0.000000000000000000, 1.000000000000000000, 0.000000000000000000 ) ) ;
#165133=CARTESIAN_POINT ( 'NONE',  ( -11.94105721839855327, 12.57301656658875544, -1.187919402540362768 ) ) ;
#165135=CARTESIAN_POINT ( 'NONE',  ( -11.93214369018126142, 7.875338098606396109, -1.299425011414485187 ) ) ;
#165143=CARTESIAN_POINT ( 'NONE',  ( -10.50000000000000000, 0.000000000000000000, 3.599999999999999201 ) ) ;
#165159=CARTESIAN_POINT ( 'NONE',  ( -15.75000000000000000, 13.40000000000000036, -1.400000000000001910 ) ) ;
#165162=CARTESIAN_POINT ( 'NONE',  ( -11.01135777277262129, 0.000000000000000000, -1.400000000000001910 ) ) ;
#165172=ORIENTED_EDGE ( 'NONE', *, *, #174500, .F. ) ;
#165191=CARTESIAN_POINT ( 'NONE',  ( 11.41381676900473430, 13.53041960022391343, -3.704697931490291918 ) ) ;
#165199=EDGE_CURVE ( 'NONE', #195013, #130986, #57830, .T. ) ;
#165200=PRESENTATION_STYLE_ASSIGNMENT (( #19996 ) ) ;
#165219=ORIENTED_EDGE ( 'NONE', *, *, #97745, .F. ) ;
#165236=AXIS2_PLACEMENT_3D ( 'NONE', #95862, #178163, #114293 ) ;
#165258=DIRECTION ( 'NONE',  ( -0.05872483221476459958, 0.000000000000000000, 0.9982742078614211811 ) ) ;
#165304=CARTESIAN_POINT ( 'NONE',  ( -3.796053574490726223, 16.00000000000285993, -12.24940615670100463 ) ) ;
#165334=UNCERTAINTY_MEASURE_WITH_UNIT (LENGTH_MEASURE( 1.000000000000000082E-05 ), #158740, 'distance_accuracy_value', 'NONE');
#165347=AXIS2_PLACEMENT_3D ( 'NONE', #72761, #138860, #188653 ) ;
#165367=SURFACE_STYLE_USAGE ( .BOTH. , #112428 ) ;
#165376=LINE ( 'NONE', #15907, #86376 ) ;
#165421=CARTESIAN_POINT ( 'NONE',  ( 9.281915779689660084, 11.43972118546268213, -7.608961053593318979 ) ) ;
#165427=ORIENTED_EDGE ( 'NONE', *, *, #69515, .F. ) ;
#165431=CARTESIAN_POINT ( 'NONE',  ( 10.78928497238454476, 8.180547903054934622, -2.738679714801448561 ) ) ;
#165441=CARTESIAN_POINT ( 'NONE',  ( 7.872831621983168660, 14.31746563593600285, -9.057160014918840929 ) ) ;
#165448=DIRECTION ( 'NONE',  ( -0.6250000000000002220, 1.408756634010579298E-16, -0.7806247497997996776 ) ) ;
#165455=SURFACE_STYLE_USAGE ( .BOTH. , #181691 ) ;
#165488=CARTESIAN_POINT ( 'NONE',  ( 0.000000000000000000, 12.21999999999998288, 0.000000000000000000 ) ) ;
#165505=AXIS2_PLACEMENT_3D ( 'NONE', #67971, #87473, #204381 ) ;
#165518=FILL_AREA_STYLE_COLOUR ( '', #172084 ) ;
#165548=EDGE_LOOP ( 'NONE', ( #126866, #152794, #6920, #45877 ) ) ;
#165564=CARTESIAN_POINT ( 'NONE',  ( -11.04536101718726293, 0.000000000000000000, -1.100000000000002087 ) ) ;
#165565=ORIENTED_EDGE ( 'NONE', *, *, #69142, .T. ) ;
#165590=FILL_AREA_STYLE_COLOUR ( '', #16336 ) ;
#165602=CARTESIAN_POINT ( 'NONE',  ( -9.407146676474797076, 14.61749904134098266, -7.348982780145471239 ) ) ;
#165615=CARTESIAN_POINT ( 'NONE',  ( 11.48767021851167414, 11.33004227463828961, 3.470194894594677226 ) ) ;
#165652=AXIS2_PLACEMENT_3D ( 'NONE', #169493, #9131, #54676 ) ;
#165693=CARTESIAN_POINT ( 'NONE',  ( -11.41381675112453564, 12.56994333910004791, 3.704697986577180302 ) ) ;
#165699=( NAMED_UNIT ( * ) PLANE_ANGLE_UNIT ( ) SI_UNIT ( $, .RADIAN. ) );
#165701=AXIS2_PLACEMENT_3D ( 'NONE', #111334, #12675, #62506 ) ;
#165716=ADVANCED_FACE ( 'NONE', ( #46652 ), #15178, .F. ) ;
#165738=EDGE_LOOP ( 'NONE', ( #149144, #21847, #74086, #61031 ) ) ;
#165748=( LENGTH_UNIT ( ) NAMED_UNIT ( * ) SI_UNIT ( .MILLI., .METRE. ) );
#165762=CARTESIAN_POINT ( 'NONE',  ( -9.367496996949647325, 15.51845925588232333, 7.500000000809289524 ) ) ;
#165777=ORIENTED_EDGE ( 'NONE', *, *, #37327, .F. ) ;
#165787=CARTESIAN_POINT ( 'NONE',  ( 10.62873463776380056, 13.79999999999998295, 3.199999999999997957 ) ) ;
#165791=CARTESIAN_POINT ( 'NONE',  ( -11.41381675112459781, 12.69999999999998863, -3.704697986577260682 ) ) ;
#165801=CARTESIAN_POINT ( 'NONE',  ( -8.158817897275659092, 15.51988520119759762, 8.845126866080887496 ) ) ;
#165846=CARTESIAN_POINT ( 'NONE',  ( -10.44369227015510404, 5.112964020592959180, 5.232143560358712087 ) ) ;
#165854=ORIENTED_EDGE ( 'NONE', *, *, #187238, .F. ) ;
#165857=COLOUR_RGB ( '', 0.66274510, 0.83137255, 0.94901961) ;
#165897=ORIENTED_EDGE ( 'NONE', *, *, #178287, .F. ) ;
#165931=CARTESIAN_POINT ( 'NONE',  ( 0.000000000000000000, 18.91999999999999815, 0.000000000000000000 ) ) ;
#165980=SURFACE_SIDE_STYLE ('',( #65256 ) ) ;
#165981=DIRECTION ( 'NONE',  ( 0.000000000000000000, 0.000000000000000000, -1.000000000000000000 ) ) ;
#165992=CARTESIAN_POINT ( 'NONE',  ( 11.99987416209243385, 8.248970243831804439, 3.607522456176011971 ) ) ;
#166005=CARTESIAN_POINT ( 'NONE',  ( -9.367496997601305608, 14.48154074412967596, 7.499999999995371702 ) ) ;
#166008=LINE ( 'NONE', #21850, #199965 ) ;
#166033=FACE_OUTER_BOUND ( 'NONE', #132713, .T. ) ;
#166044=CARTESIAN_POINT ( 'NONE',  ( -9.348561386899501002, 3.999985931113709814, -7.001914024221969512 ) ) ;
#166045=CARTESIAN_POINT ( 'NONE',  ( -9.915825940873133959, 4.173851563286998356, 6.175246223022227809 ) ) ;
#166090=CARTESIAN_POINT ( 'NONE',  ( 9.167121402339585501, 14.44227982134217569, -8.755495446810726889 ) ) ;
#166111=CIRCLE ( 'NONE', #38104, 12.00000000000000355 ) ;
#166149=CARTESIAN_POINT ( 'NONE',  ( 11.94980361058168938, 13.40000000000000036, -1.100000000000000311 ) ) ;
#166168=ADVANCED_FACE ( 'NONE', ( #22628 ), #24731, .T. ) ;
#166194=CARTESIAN_POINT ( 'NONE',  ( -10.91033749632886973, 4.885617943545218722, -4.996452313011734425 ) ) ;
#166217=ORIENTED_EDGE ( 'NONE', *, *, #213665, .F. ) ;
#166222=PRESENTATION_STYLE_ASSIGNMENT (( #202967 ) ) ;
#166223=SURFACE_SIDE_STYLE ('',( #149987 ) ) ;
#166255=CARTESIAN_POINT ( 'NONE',  ( -0.08053691275167716712, 15.51846456562902965, 11.99972973886013961 ) ) ;
#166256=CARTESIAN_POINT ( 'NONE',  ( 11.48243876534946217, 13.88000000000000078, -3.200000000000001510 ) ) ;
#166317=AXIS2_PLACEMENT_3D ( 'NONE', #113927, #179923, #60834 ) ;
#166324=SURFACE_STYLE_USAGE ( .BOTH. , #36309 ) ;
#166345=UNCERTAINTY_MEASURE_WITH_UNIT (LENGTH_MEASURE( 1.000000000000000082E-05 ), #173248, 'distance_accuracy_value', 'NONE');
#166373=CARTESIAN_POINT ( 'NONE',  ( -10.93392920578941485, 5.995216197940580471, 6.296921006145307587 ) ) ;
#166384=ORIENTED_EDGE ( 'NONE', *, *, #107473, .T. ) ;
#166414=CIRCLE ( 'NONE', #73008, 0.07999999999999971023 ) ;
#166422=ADVANCED_FACE ( 'NONE', ( #95137 ), #119683, .T. ) ;
#166459=CARTESIAN_POINT ( 'NONE',  ( -10.91033920341459051, 4.885615726745599297, 4.996448585388897357 ) ) ;
#166474=CARTESIAN_POINT ( 'NONE',  ( -10.14898710519052649, 3.000029897349846930, -7.601419320309957151 ) ) ;
#166486=FILL_AREA_STYLE_COLOUR ( '', #25955 ) ;
#166492=CARTESIAN_POINT ( 'NONE',  ( 11.96807573623599552, 6.670661610224271953, 1.000409426482763875 ) ) ;
#166496=VERTEX_POINT ( 'NONE', #6121 ) ;
#166503=CARTESIAN_POINT ( 'NONE',  ( 9.553970131394970977, 11.68474399595152136, -6.135158682309066691 ) ) ;
#166515=CARTESIAN_POINT ( 'NONE',  ( 8.810048391696781778, 13.28851571758703720, -8.147727092588498365 ) ) ;
#166529=CARTESIAN_POINT ( 'NONE',  ( -15.75000000000000000, 12.30000000000000071, 0.6999999999999992895 ) ) ;
#166530=EDGE_CURVE ( 'NONE', #172216, #105059, #197068, .T. ) ;
#166534=LINE ( 'NONE', #66856, #202309 ) ;
#166548=CARTESIAN_POINT ( 'NONE',  ( -9.585712968046856020, 14.76505204444259256, -7.219336745274212319 ) ) ;
#166629=DIRECTION ( 'NONE',  ( 0.000000000000000000, 1.000000000000000000, 0.000000000000000000 ) ) ;
#166634=AXIS2_PLACEMENT_3D ( 'NONE', #7940, #203988, #56711 ) ;
#166636=B_SPLINE_CURVE_WITH_KNOTS ( 'NONE', 3,
 ( #74810, #144120, #160321, #110572, #189614, #43389 ),
 .UNSPECIFIED., .F., .F.,
 ( 4, 2, 4 ),
 ( 0.000000000000000000, 0.0003845013059668469482, 0.0007690026119336938965 ),
 .UNSPECIFIED. ) ;
#166642=CARTESIAN_POINT ( 'NONE',  ( -10.59752019245792987, 11.30000000000000071, -3.303678142506601745 ) ) ;
#166673=CARTESIAN_POINT ( 'NONE',  ( -9.367496997601184816, 15.42330868760440410, -7.413898975931886959 ) ) ;
#166685=( NAMED_UNIT ( * ) SI_UNIT ( $, .STERADIAN. ) SOLID_ANGLE_UNIT ( ) );
#166714=CARTESIAN_POINT ( 'NONE',  ( 8.627766630430368622, 13.75162864925633244, 8.275246034657209648 ) ) ;
#166754=CARTESIAN_POINT ( 'NONE',  ( 11.78331023100045627, 9.799999999999998934, -1.800000000000001155 ) ) ;
#166770=DIRECTION ( 'NONE',  ( -0.8164965809277262565, 8.702247276351162783E-15, 0.5773502691896256200 ) ) ;
#166771=CARTESIAN_POINT ( 'NONE',  ( -11.00592740523952351, 13.61020242468316432, 1.444008943503716225 ) ) ;
#166772=CARTESIAN_POINT ( 'NONE',  ( -9.644676237148278375, 5.067654118421841325, 6.575762993896887565 ) ) ;
#166782=CARTESIAN_POINT ( 'NONE',  ( -11.33772465723237666, 11.00868300734826910, 3.600000000000073364 ) ) ;
#166816=FACE_OUTER_BOUND ( 'NONE', #208551, .T. ) ;
#166823=AXIS2_PLACEMENT_3D ( 'NONE', #105095, #102944, #106195 ) ;
#166841=LINE ( 'NONE', #131206, #144695 ) ;
#166848=FACE_OUTER_BOUND ( 'NONE', #128967, .T. ) ;
#166849=DIRECTION ( 'NONE',  ( 0.000000000000000000, 0.000000000000000000, 1.000000000000000000 ) ) ;
#166866=CARTESIAN_POINT ( 'NONE',  ( 11.86239285000045918, 11.30000000000000249, -1.812080536912752837 ) ) ;
#166885=CARTESIAN_POINT ( 'NONE',  ( -11.07790593930098311, 12.30000000000000071, 0.6999999999999992895 ) ) ;
#166886=SURFACE_SIDE_STYLE ('',( #21651 ) ) ;
#166920=FACE_OUTER_BOUND ( 'NONE', #132210, .T. ) ;
#166952=CARTESIAN_POINT ( 'NONE',  ( -9.586287156395091102, 15.23335157185452893, -7.218579095505596399 ) ) ;
#166974=FACE_OUTER_BOUND ( 'NONE', #187732, .T. ) ;
#166980=CARTESIAN_POINT ( 'NONE',  ( -10.42522259430890763, 5.087348912241797194, -5.944660150690117106 ) ) ;
#167032=CARTESIAN_POINT ( 'NONE',  ( 11.86686399458719698, 11.10928729775336876, 1.056461745586970258 ) ) ;
#167034=DIRECTION ( 'NONE',  ( -0.6250000000000005551, 0.000000000000000000, 0.7806247497997993445 ) ) ;
#167054=CARTESIAN_POINT ( 'NONE',  ( -11.87992086682929660, 5.100687730227392969, -4.764507118098673111 ) ) ;
#167066=CARTESIAN_POINT ( 'NONE',  ( 12.43309052428753070, 7.572468744233063376, 1.895192891247173606 ) ) ;
#167084=CARTESIAN_POINT ( 'NONE',  ( 11.86145017354043674, 12.59514365543877012, -1.100000000000000533 ) ) ;
#167099=AXIS2_PLACEMENT_3D ( 'NONE', #79791, #145905, #15838 ) ;
#167110=( NAMED_UNIT ( * ) PLANE_ANGLE_UNIT ( ) SI_UNIT ( $, .RADIAN. ) );
#167139=VERTEX_POINT ( 'NONE', #145325 ) ;
#167167=CARTESIAN_POINT ( 'NONE',  ( 9.027736952715539331, 13.49050362732109143, -9.153502459270221436 ) ) ;
#167182=CARTESIAN_POINT ( 'NONE',  ( 11.91294103507080848, 13.61460089956416297, -1.446263142085534747 ) ) ;
#167194=CARTESIAN_POINT ( 'NONE',  ( -10.71030397718323890, 6.055815897892919075, -4.668189396100475008 ) ) ;
#167196=ADVANCED_FACE ( 'NONE', ( #147421 ), #197737, .T. ) ;
#167226=CARTESIAN_POINT ( 'NONE',  ( 11.89197369110779512, 11.30000000000000071, -0.8056055387119873679 ) ) ;
#167250=VECTOR ( 'NONE', #3527, 1000.000000000000000 ) ;
#167265=CARTESIAN_POINT ( 'NONE',  ( -3.099815351088664794, 14.55179009333156159, -11.55525895789692292 ) ) ;
#167300=CARTESIAN_POINT ( 'NONE',  ( 0.000000000000000000, 13.88000000000000078, 0.000000000000000000 ) ) ;
#167324=ORIENTED_EDGE ( 'NONE', *, *, #38452, .T. ) ;
#167330=CARTESIAN_POINT ( 'NONE',  ( -10.50000000000000355, 12.59281572507203606, 3.599999999999998312 ) ) ;
#167376=DIRECTION ( 'NONE',  ( 0.000000000000000000, 1.000000000000000000, 0.000000000000000000 ) ) ;
#167396=CARTESIAN_POINT ( 'NONE',  ( -11.86239285000045740, 13.79999999999998472, 1.812080536912751061 ) ) ;
#167399=DIRECTION ( 'NONE',  ( 0.000000000000000000, -1.000000000000000000, -9.023263958591317418E-17 ) ) ;
#167421=DIRECTION ( 'NONE',  ( 0.8003905296791061774, 0.000000000000000000, -0.5994789404140897782 ) ) ;
#167446=CARTESIAN_POINT ( 'NONE',  ( -10.02511099414689077, 5.770000865873268658, 5.887978427067937837 ) ) ;
#167473=ORIENTED_EDGE ( 'NONE', *, *, #140577, .T. ) ;
#167474=UNCERTAINTY_MEASURE_WITH_UNIT (LENGTH_MEASURE( 1.000000000000000082E-05 ), #30665, 'distance_accuracy_value', 'NONE');
#167481=DIRECTION ( 'NONE',  ( 0.000000000000000000, 1.000000000000000000, 0.000000000000000000 ) ) ;
#167533=ORIENTED_EDGE ( 'NONE', *, *, #107860, .F. ) ;
#167537=ORIENTED_EDGE ( 'NONE', *, *, #35147, .T. ) ;
#167542=CARTESIAN_POINT ( 'NONE',  ( 0.000000000000000000, 7.000000000000000000, 0.000000000000000000 ) ) ;
#167543=CARTESIAN_POINT ( 'NONE',  ( -11.55090974143167060, 4.033601484819619110, -5.407241547083907918 ) ) ;
#167545=CIRCLE ( 'NONE', #74169, 11.92000000000000171 ) ;
#167550=DIRECTION ( 'NONE',  ( -0.000000000000000000, -1.000000000000000000, -0.000000000000000000 ) ) ;
#167554=CARTESIAN_POINT ( 'NONE',  ( -10.78227258717170578, 6.269840026405313793, 4.500979083849748541 ) ) ;
#167557=CIRCLE ( 'NONE', #115829, 10.75000000000000000 ) ;
#167561=CARTESIAN_POINT ( 'NONE',  ( 11.96846072664349769, 6.616964094891172543, -0.9998397279549741112 ) ) ;
#167573=CARTESIAN_POINT ( 'NONE',  ( 9.258966325506428063, 13.63624071251986081, -6.830021722722439570 ) ) ;
#167576=ORIENTED_EDGE ( 'NONE', *, *, #5717, .T. ) ;
#167580=MECHANICAL_DESIGN_GEOMETRIC_PRESENTATION_REPRESENTATION('',(#112307),#63839);
#167584=CARTESIAN_POINT ( 'NONE',  ( 7.679631683607862414, 14.45130440965375662, -9.163852989591987352 ) ) ;
#167585=CARTESIAN_POINT ( 'NONE',  ( -8.804225388950451148, 15.46908216042836060, -8.203526012298418379 ) ) ;
#167586=CARTESIAN_POINT ( 'NONE',  ( -11.89835103415199313, 12.27106914167534057, -1.561208891256348652 ) ) ;
#167590=COLOUR_RGB ( '', 0.40784314, 0.44705882, 0.49803922) ;
#167592=CARTESIAN_POINT ( 'NONE',  ( -11.86145016429273014, 12.69999999999999929, -1.100000000000000311 ) ) ;
#167623=LINE ( 'NONE', #181716, #70623 ) ;
#167647=ORIENTED_EDGE ( 'NONE', *, *, #96671, .T. ) ;
#167655=( NAMED_UNIT ( * ) PLANE_ANGLE_UNIT ( ) SI_UNIT ( $, .RADIAN. ) );
#167678=CARTESIAN_POINT ( 'NONE',  ( -10.50000000000000000, 13.40000000000000036, -3.600000000000002309 ) ) ;
#167690=DIRECTION ( 'NONE',  ( 0.000000000000000000, 1.000000000000000000, 0.000000000000000000 ) ) ;
#167697=CIRCLE ( 'NONE', #39843, 0.08000000000000020983 ) ;
#167711=CARTESIAN_POINT ( 'NONE',  ( -9.585712967628772674, 15.23494795713225436, 7.219336745831919977 ) ) ;
#167720=CIRCLE ( 'NONE', #185014, 11.68000000000000149 ) ;
#167726=VERTEX_POINT ( 'NONE', #107455 ) ;
#167734=EDGE_CURVE ( 'NONE', #148685, #18470, #163138, .T. ) ;
#167747=DIRECTION ( 'NONE',  ( -0.6249999999999993339, 2.638740015698311463E-15, 0.7806247497998004548 ) ) ;
#167749=AXIS2_PLACEMENT_3D ( 'NONE', #68668, #84941, #147830 ) ;
#167754=EDGE_CURVE ( 'NONE', #147625, #30835, #31750, .T. ) ;
#167768=CARTESIAN_POINT ( 'NONE',  ( 9.367496997597594799, 3.481548657788670731, -7.500000000000007105 ) ) ;
#167796=ORIENTED_EDGE ( 'NONE', *, *, #64145, .T. ) ;
#167830=CARTESIAN_POINT ( 'NONE',  ( -15.75000000000000000, 12.69999999999999929, -1.800000000000001155 ) ) ;
#167842=CARTESIAN_POINT ( 'NONE',  ( -11.55950211276791073, 11.29999999999998295, 3.221476510067111665 ) ) ;
#167855=B_SPLINE_CURVE_WITH_KNOTS ( 'NONE', 3,
 ( #64878, #182896, #183962, #197015, #48651, #83254 ),
 .UNSPECIFIED., .F., .F.,
 ( 4, 2, 4 ),
 ( 0.000000000000000000, 0.0003172254002810710651, 0.0006344508005621421302 ),
 .UNSPECIFIED. ) ;
#167858=CARTESIAN_POINT ( 'NONE',  ( -11.55950211276791428, 11.37999999999999901, -3.221476510067114329 ) ) ;
#167868=ORIENTED_EDGE ( 'NONE', *, *, #44567, .T. ) ;
#167882=DIRECTION ( 'NONE',  ( 0.000000000000000000, 0.000000000000000000, 1.000000000000000000 ) ) ;
#167887=CARTESIAN_POINT ( 'NONE',  ( -11.06299035296667732, 9.843162956239048356, -0.9087041361035911313 ) ) ;
#167911=ORIENTED_EDGE ( 'NONE', *, *, #63078, .T. ) ;
#167912=CIRCLE ( 'NONE', #74538, 0.08000000000000020983 ) ;
#167938=DIRECTION ( 'NONE',  ( -0.9885327375000381167, 0.000000000000000000, 0.1510067114093955609 ) ) ;
#167954=ORIENTED_EDGE ( 'NONE', *, *, #7569, .T. ) ;
#167980=UNCERTAINTY_MEASURE_WITH_UNIT (LENGTH_MEASURE( 1.000000000000000082E-05 ), #193242, 'distance_accuracy_value', 'NONE');
#167985=ORIENTED_EDGE ( 'NONE', *, *, #85069, .T. ) ;
#168029=CARTESIAN_POINT ( 'NONE',  ( -10.56742348559178879, 4.157028815770352104, -5.593809627444244370 ) ) ;
#168035=EDGE_CURVE ( 'NONE', #180190, #58569, #128275, .T. ) ;
#168037=CARTESIAN_POINT ( 'NONE',  ( -11.89844258446856529, 12.27147310670038571, -1.560502987793169094 ) ) ;
#168093=ORIENTED_EDGE ( 'NONE', *, *, #151057, .F. ) ;
#168102=ORIENTED_EDGE ( 'NONE', *, *, #74664, .F. ) ;
#168103=CARTESIAN_POINT ( 'NONE',  ( 11.04536101718726293, 12.69999999999999929, -1.100000000000000311 ) ) ;
#168111=CARTESIAN_POINT ( 'NONE',  ( 11.00605293250196226, 13.60925261358443095, -1.443095658425808114 ) ) ;
#168117=CARTESIAN_POINT ( 'NONE',  ( -10.91672646594461327, 4.673612064222224305, 4.467269497407427181 ) ) ;
#168127=CARTESIAN_POINT ( 'NONE',  ( 10.81425746553161460, 10.30853785568457326, -6.489671246970442731 ) ) ;
#168140=CARTESIAN_POINT ( 'NONE',  ( 11.97178994924802353, 12.22000006202794609, -0.8322011300497145214 ) ) ;
#168178=CARTESIAN_POINT ( 'NONE',  ( -11.92619526913700057, 19.00000000000000000, -1.328859060402686199 ) ) ;
#168183=CARTESIAN_POINT ( 'NONE',  ( -11.13994541198518640, 5.786402032167232257, -4.475860200623921870 ) ) ;
#168226=EDGE_CURVE ( 'NONE', #77503, #134499, #62461, .T. ) ;
#168228=CARTESIAN_POINT ( 'NONE',  ( 8.964365016547233722, 14.59103508737832300, -8.971863053630826812 ) ) ;
#168234=ORIENTED_EDGE ( 'NONE', *, *, #171794, .T. ) ;
#168243=CARTESIAN_POINT ( 'NONE',  ( -9.953865251629775202, 4.532720649454268447, -6.624712979280865888 ) ) ;
#168259=CARTESIAN_POINT ( 'NONE',  ( 7.188044520085388633, 15.44694694233605148, -9.560164038293452293 ) ) ;
#168266=EDGE_CURVE ( 'NONE', #63230, #18446, #145542, .T. ) ;
#168274=CARTESIAN_POINT ( 'NONE',  ( 8.220324289656684158, 15.16505199276374150, 8.682849841995956552 ) ) ;
#168275=CARTESIAN_POINT ( 'NONE',  ( -11.92619526913699879, 13.39999999999998259, 1.328859060402684644 ) ) ;
#168278=EDGE_CURVE ( 'NONE', #146971, #129573, #176576, .T. ) ;
#168286=ADVANCED_FACE ( 'NONE', ( #46667 ), #61435, .T. ) ;
#168289=CARTESIAN_POINT ( 'NONE',  ( 11.97929049433706084, 13.79999999999999893, -0.7046979865771820783 ) ) ;
#168297=ORIENTED_EDGE ( 'NONE', *, *, #14021, .F. ) ;
#168315=CARTESIAN_POINT ( 'NONE',  ( 0.000000000000000000, 18.91999999999999815, 11.92000000000000171 ) ) ;
#168320=CIRCLE ( 'NONE', #78479, 0.5000000000000004441 ) ;
#168344=CARTESIAN_POINT ( 'NONE',  ( -11.16790076368576834, 7.276266301664604086, 4.397334502061439387 ) ) ;
#168349=VECTOR ( 'NONE', #2903, 1000.000000000000000 ) ;
#168360=CARTESIAN_POINT ( 'NONE',  ( -11.94655611907589865, 9.947990554530955265, -1.134828163062138628 ) ) ;
#168364=VERTEX_POINT ( 'NONE', #167858 ) ;
#168389=CARTESIAN_POINT ( 'NONE',  ( -10.29915967087783102, 4.864502100071391943, 6.165526146199510116 ) ) ;
#168435=CARTESIAN_POINT ( 'NONE',  ( 11.84668730067608244, 10.19999999999998153, 1.319999999999998286 ) ) ;
#168439=ORIENTED_EDGE ( 'NONE', *, *, #171367, .T. ) ;
#168477=UNCERTAINTY_MEASURE_WITH_UNIT (LENGTH_MEASURE( 1.000000000000000082E-05 ), #97201, 'distance_accuracy_value', 'NONE');
#168478=CARTESIAN_POINT ( 'NONE',  ( -10.56513397747884397, 11.25900096514340198, 3.405015282931166620 ) ) ;
#168502=CARTESIAN_POINT ( 'NONE',  ( -8.752560982292409975, 14.99999996918461775, -9.356054898121708874 ) ) ;
#168504=CARTESIAN_POINT ( 'NONE',  ( -11.40891844150367618, 9.366729182080655747, 1.257950088934312705 ) ) ;
#168505=CIRCLE ( 'NONE', #102800, 0.07999999999999986289 ) ;
#168516=STYLED_ITEM ( 'NONE', ( #42 ), #145158 ) ;
#168548=FILL_AREA_STYLE_COLOUR ( '', #77116 ) ;
#168594=ORIENTED_EDGE ( 'NONE', *, *, #75095, .F. ) ;
#168599=EDGE_LOOP ( 'NONE', ( #131674, #17439, #159188, #170112, #147694 ) ) ;
#168606=CARTESIAN_POINT ( 'NONE',  ( -10.21576913194658864, 4.000029896383376027, -7.512182378973799146 ) ) ;
#168615=PLANE ( 'NONE',  #109066 ) ;
#168621=CARTESIAN_POINT ( 'NONE',  ( 11.96769518616268080, 6.617733873879387829, 1.006560610218020679 ) ) ;
#168630=ORIENTED_EDGE ( 'NONE', *, *, #126323, .T. ) ;
#168632=( NAMED_UNIT ( * ) PLANE_ANGLE_UNIT ( ) SI_UNIT ( $, .RADIAN. ) );
#168633=CARTESIAN_POINT ( 'NONE',  ( 8.825993893598074180, 13.26473029764630773, -7.662602092427571954 ) ) ;
#168646=CIRCLE ( 'NONE', #19903, 11.92000000000000171 ) ;
#168648=EDGE_CURVE ( 'NONE', #210028, #30243, #106586, .T. ) ;
#168659=CIRCLE ( 'NONE', #75288, 0.07999999999999998779 ) ;
#168688=DIRECTION ( 'NONE',  ( -0.1510067114093955887, 0.000000000000000000, 0.9885327375000383388 ) ) ;
#168724=EDGE_CURVE ( 'NONE', #121123, #29604, #142592, .T. ) ;
#168748=AXIS2_PLACEMENT_3D ( 'NONE', #100994, #149766, #183316 ) ;
#168756=PRESENTATION_STYLE_ASSIGNMENT (( #199090 ) ) ;
#168805=AXIS2_PLACEMENT_3D ( 'NONE', #71637, #171292, #22884 ) ;
#168814=CARTESIAN_POINT ( 'NONE',  ( 11.55950211276791428, 13.87999999999998302, 3.221476510067112109 ) ) ;
#168820=DIRECTION ( 'NONE',  ( -0.000000000000000000, -1.000000000000000000, 0.000000000000000000 ) ) ;
#168841=CIRCLE ( 'NONE', #3226, 0.08000000000000020983 ) ;
#168889=EDGE_CURVE ( 'NONE', #11196, #198793, #54110, .T. ) ;
#168902=CARTESIAN_POINT ( 'NONE',  ( -11.33772463945043718, 10.89999999999999147, 3.600000000000075140 ) ) ;
#168908=CIRCLE ( 'NONE', #86039, 0.5000000000000011102 ) ;
#168933=CARTESIAN_POINT ( 'NONE',  ( 11.92619526913699879, 10.89999999999998259, 1.328859060402684644 ) ) ;
#168979=CARTESIAN_POINT ( 'NONE',  ( 11.52463353791760703, 11.37999999999998302, 3.346594096177640587 ) ) ;
#168987=STYLED_ITEM ( 'NONE', ( #80926 ), #39677 ) ;
#169027=FILL_AREA_STYLE ('',( #154923 ) ) ;
#169038=CARTESIAN_POINT ( 'NONE',  ( -10.81659190237994395, 5.544392656652913587, 6.534142543513654644 ) ) ;
#169039=ORIENTED_EDGE ( 'NONE', *, *, #98945, .F. ) ;
#169041=CARTESIAN_POINT ( 'NONE',  ( -1.249999999999964695, 8.500000000000000000, 10.97907099895069294 ) ) ;
#169055=VERTEX_POINT ( 'NONE', #114394 ) ;
#169085=ORIENTED_EDGE ( 'NONE', *, *, #127184, .F. ) ;
#169091=CARTESIAN_POINT ( 'NONE',  ( 11.78331023100045627, 11.37999999999998302, 1.799999999999999600 ) ) ;
#169122=CARTESIAN_POINT ( 'NONE',  ( -7.090393287529871635, 15.44810098017736166, -9.636374456359583007 ) ) ;
#169150=ORIENTED_EDGE ( 'NONE', *, *, #68660, .F. ) ;
#169161=ORIENTED_EDGE ( 'NONE', *, *, #21226, .F. ) ;
#169168=CIRCLE ( 'NONE', #182918, 0.5000000000000008882 ) ;
#169175=CARTESIAN_POINT ( 'NONE',  ( -10.97409330344778944, 4.894225957061862253, -4.351021568302368969 ) ) ;
#169202=CARTESIAN_POINT ( 'NONE',  ( 11.86685672517501899, 12.49081082140188670, -1.056525322636012065 ) ) ;
#169204=ADVANCED_FACE ( 'NONE', ( #95968 ), #197688, .T. ) ;
#169237=VERTEX_POINT ( 'NONE', #159874 ) ;
#169242=CARTESIAN_POINT ( 'NONE',  ( -9.587704862635016312, 4.026159954882873926, 6.671158199369250141 ) ) ;
#169250=ADVANCED_FACE ( 'NONE', ( #11479 ), #100483, .T. ) ;
#169290=CARTESIAN_POINT ( 'NONE',  ( 8.523031442321446605, 14.76712986476217715, -9.394111251778250349 ) ) ;
#169296=ADVANCED_FACE ( 'NONE', ( #21046 ), #184630, .T. ) ;
#169339=( NAMED_UNIT ( * ) SI_UNIT ( $, .STERADIAN. ) SOLID_ANGLE_UNIT ( ) );
#169346=DIRECTION ( 'NONE',  ( 7.993605777301127091E-15, 0.000000000000000000, 1.000000000000000000 ) ) ;
#169407=CARTESIAN_POINT ( 'NONE',  ( -11.41492544888517990, 7.843637262818779377, 3.710592433486775921 ) ) ;
#169424=DIRECTION ( 'NONE',  ( -0.000000000000000000, -1.000000000000000000, -0.000000000000000000 ) ) ;
#169434=ADVANCED_FACE ( 'NONE', ( #124480 ), #86889, .F. ) ;
#169459=CARTESIAN_POINT ( 'NONE',  ( -10.81391327432222838, 6.436729623570534464, -5.219172391766678132 ) ) ;
#169477=EDGE_CURVE ( 'NONE', #6177, #181174, #31340, .T. ) ;
#169485=CARTESIAN_POINT ( 'NONE',  ( 10.95308175811721085, 13.79999999999999893, -1.800000000000001155 ) ) ;
#169493=CARTESIAN_POINT ( 'NONE',  ( -11.33772463945036968, 10.90000000000000036, -3.680000000000001048 ) ) ;
#169511=CARTESIAN_POINT ( 'NONE',  ( 11.33772463945037146, 13.39999999999998259, 3.599999999999999201 ) ) ;
#169520=SURFACE_SIDE_STYLE ('',( #198797 ) ) ;
#169537=CARTESIAN_POINT ( 'NONE',  ( 11.86145016429273191, 10.90000000000000036, -1.100000000000002087 ) ) ;
#169572=CARTESIAN_POINT ( 'NONE',  ( -9.997759874121660673, 5.662387697485826266, 5.943071269081472430 ) ) ;
#169589=LINE ( 'NONE', #105691, #211602 ) ;
#169591=CARTESIAN_POINT ( 'NONE',  ( -10.20548264327394428, 4.735695117630401185, 6.229399736498809403 ) ) ;
#169596=VERTEX_POINT ( 'NONE', #214113 ) ;
#169601=ORIENTED_EDGE ( 'NONE', *, *, #70447, .T. ) ;
#169604=FILL_AREA_STYLE_COLOUR ( '', #165857 ) ;
#169613=DIRECTION ( 'NONE',  ( -0.000000000000000000, -1.000000000000000000, -0.000000000000000000 ) ) ;
#169628=CARTESIAN_POINT ( 'NONE',  ( 11.04536101718726293, 10.19999999999999929, 1.099999999999996758 ) ) ;
#169640=ORIENTED_EDGE ( 'NONE', *, *, #22794, .F. ) ;
#169674=CARTESIAN_POINT ( 'NONE',  ( -9.348596576284975868, 2.999985932080179829, -7.001940380475246251 ) ) ;
#169684=CARTESIAN_POINT ( 'NONE',  ( -10.71026998871754721, 6.055660674263378951, 4.667787751035539223 ) ) ;
#169688=ORIENTED_EDGE ( 'NONE', *, *, #74664, .T. ) ;
#169690=CARTESIAN_POINT ( 'NONE',  ( 10.93263675336509522, 8.268585769907408789, -4.963831765784436634 ) ) ;
#169692=ORIENTED_EDGE ( 'NONE', *, *, #35147, .F. ) ;
#169695=EDGE_LOOP ( 'NONE', ( #19871, #103957, #81250, #175645 ) ) ;
#169713=CARTESIAN_POINT ( 'NONE',  ( -6.723453079147375000, 15.44785978006343896, -9.895885313386967752 ) ) ;
#169715=ORIENTED_EDGE ( 'NONE', *, *, #23547, .F. ) ;
#169743=( NAMED_UNIT ( * ) SI_UNIT ( $, .STERADIAN. ) SOLID_ANGLE_UNIT ( ) );
#169754=AXIS2_PLACEMENT_3D ( 'NONE', #63403, #180352, #129556 ) ;
#169785=FACE_OUTER_BOUND ( 'NONE', #68443, .T. ) ;
#169815=COLOUR_RGB ( '', 0.09019608, 0.27058824, 0.51372549) ;
#169827=CARTESIAN_POINT ( 'NONE',  ( 11.43190902327452108, 12.44477871742131825, 3.649704988378163595 ) ) ;
#169829=DIRECTION ( 'NONE',  ( 1.000000000000000000, -0.000000000000000000, -0.000000000000000000 ) ) ;
#169842=FACE_OUTER_BOUND ( 'NONE', #28764, .T. ) ;
#169853=CARTESIAN_POINT ( 'NONE',  ( 11.97929049433705373, 13.88000000000000078, 0.7046979865771783036 ) ) ;
#169870=SURFACE_STYLE_USAGE ( .BOTH. , #67012 ) ;
#169871=AXIS2_PLACEMENT_3D ( 'NONE', #101408, #167481, #27360 ) ;
#169884=EDGE_CURVE ( 'NONE', #45649, #1299, #79911, .T. ) ;
#169903=CARTESIAN_POINT ( 'NONE',  ( -11.81900460097218186, 9.842428651258600780, 1.592493057836596115 ) ) ;
#169940=CARTESIAN_POINT ( 'NONE',  ( -11.87815913191726480, 9.796921793685831048, 1.708869976696563597 ) ) ;
#169954=FACE_BOUND ( 'NONE', #139091, .T. ) ;
#169955=CARTESIAN_POINT ( 'NONE',  ( -9.399990540229763880, 5.000000000000003553, 6.933248713717822476 ) ) ;
#170006=FILL_AREA_STYLE_COLOUR ( '', #47275 ) ;
#170009=DIRECTION ( 'NONE',  ( -0.000000000000000000, -1.000000000000000000, 0.000000000000000000 ) ) ;
#170050=CARTESIAN_POINT ( 'NONE',  ( -9.367496996949647325, 15.51845925588232689, 7.500000000809292189 ) ) ;
#170066=AXIS2_PLACEMENT_3D ( 'NONE', #136699, #25059, #56508 ) ;
#170099=CARTESIAN_POINT ( 'NONE',  ( -11.66902918085182250, 4.335764935525111774, 5.185761432613135824 ) ) ;
#170107=ORIENTED_EDGE ( 'NONE', *, *, #137597, .F. ) ;
#170112=ORIENTED_EDGE ( 'NONE', *, *, #161732, .T. ) ;
#170113=FILL_AREA_STYLE ('',( #153884 ) ) ;
#170132=CARTESIAN_POINT ( 'NONE',  ( -9.438074503189328723, 14.51398094803501060, -7.411038319754888803 ) ) ;
#170157=DIRECTION ( 'NONE',  ( -0.8003905296791066215, 0.000000000000000000, 0.5994789404140892231 ) ) ;
#170164=CARTESIAN_POINT ( 'NONE',  ( 11.33772463945036790, 13.50911576511426304, -3.600000000000000089 ) ) ;
#170169=DIRECTION ( 'NONE',  ( 1.000000000000000000, -0.000000000000000000, -0.000000000000000000 ) ) ;
#170182=CARTESIAN_POINT ( 'NONE',  ( -6.723431022862452089, 15.44785976354745749, -9.895899930522206844 ) ) ;
#170184=AXIS2_PLACEMENT_3D ( 'NONE', #107337, #174429, #160285 ) ;
#170192=ADVANCED_FACE ( 'NONE', ( #37543 ), #153437, .F. ) ;
#170217=TOROIDAL_SURFACE ( 'NONE', #24860, 11.18000000000000149, 0.08000000000000000167 ) ;
#170218=SURFACE_SIDE_STYLE ('',( #70556 ) ) ;
#170228=ORIENTED_EDGE ( 'NONE', *, *, #163457, .F. ) ;
#170238=CARTESIAN_POINT ( 'NONE',  ( -10.96041802301306944, 4.843384909922287207, -4.379099270644332798 ) ) ;
#170250=( BOUNDED_SURFACE ( )  B_SPLINE_SURFACE ( 3, 2, ( 
 ( #37932, #104006, #170050 ),
 ( #68268, #5390, #149549 ),
 ( #49918, #133334, #165801 ),
 ( #190561, #23797, #137580 ),
 ( #90964, #89902, #157029 ),
 ( #139723, #122476, #42217 ),
 ( #174353, #8616, #138644 ),
 ( #22717, #203598, #171123 ),
 ( #188437, #155954, #40071 ),
 ( #74698, #55250, #140802 ),
 ( #187370, #106182, #58447 ),
 ( #41152, #108333, #121397 ),
 ( #205746, #88831, #206813 ),
 ( #141871, #107261, #92040 ) ),
 .UNSPECIFIED., .F., .F., .T. ) 
 B_SPLINE_SURFACE_WITH_KNOTS ( ( 4, 2, 2, 2, 2, 2, 4 ),
 ( 3, 3 ),
 ( 0.01742726433212075238, 0.02010289811550490524, 0.02144071500719698167, 0.02277853189888905810, 0.02411634879058113454, 0.02545416568227321097, 0.02812979946565736036 ),
 ( 0.000000000000000000, 1.000000000000000000 ),
 .UNSPECIFIED. ) 
 GEOMETRIC_REPRESENTATION_ITEM ( )  RATIONAL_B_SPLINE_SURFACE ( (
 ( 1.000000000000000000, 0.8509629433930189224, 1.000000000000000000),
 ( 1.000000000000000000, 0.8507262248946917405, 1.000000000000000000),
 ( 1.000000000000000000, 0.8494479596845089242, 1.000000000000000000),
 ( 1.000000000000000000, 0.8495361673793808688, 1.000000000000000000),
 ( 1.000000000000000000, 0.8498393499228069636, 1.000000000000000000),
 ( 1.000000000000000000, 0.8505768930579380438, 1.000000000000000000),
 ( 1.000000000000000000, 0.8510027784581069010, 1.000000000000000000),
 ( 1.000000000000000000, 0.8509174126978680253, 1.000000000000000000),
 ( 1.000000000000000000, 0.8504342006050041869, 1.000000000000000000),
 ( 1.000000000000000000, 0.8496654783626688134, 1.000000000000000000),
 ( 1.000000000000000000, 0.8493814140782459665, 1.000000000000000000),
 ( 1.000000000000000000, 0.8494163377631810397, 1.000000000000000000),
 ( 1.000000000000000000, 0.8508375213763882394, 1.000000000000000000),
 ( 1.000000000000000000, 0.8509612879365336946, 1.000000000000000000) ) ) 
 REPRESENTATION_ITEM ( '' )  SURFACE ( )  );
#170264=LINE ( 'NONE', #39206, #193017 ) ;
#170288=SURFACE_STYLE_FILL_AREA ( #104242 ) ;
#170318=VERTEX_POINT ( 'NONE', #206439 ) ;
#170349=CARTESIAN_POINT ( 'NONE',  ( 0.000000000000000000, 4.518459255872631530, 0.000000000000000000 ) ) ;
#170350=DIRECTION ( 'NONE',  ( 0.000000000000000000, 0.000000000000000000, 1.000000000000000000 ) ) ;
#170356=ORIENTED_EDGE ( 'NONE', *, *, #173988, .T. ) ;
#170368=CARTESIAN_POINT ( 'NONE',  ( 11.41381675112453387, 10.19999999999998153, 3.704697986577180746 ) ) ;
#170392=ORIENTED_EDGE ( 'NONE', *, *, #208132, .F. ) ;
#170399=CARTESIAN_POINT ( 'NONE',  ( -9.367496997601914899, 15.46908218389976497, 7.499999999994665600 ) ) ;
#170403=CARTESIAN_POINT ( 'NONE',  ( 8.717716733090741243, 13.27471476138783224, 8.129441245349513068 ) ) ;
#170472=ORIENTED_EDGE ( 'NONE', *, *, #91659, .T. ) ;
#170479=CIRCLE ( 'NONE', #49435, 0.08000000000000014044 ) ;
#170509=VERTEX_POINT ( 'NONE', #45043 ) ;
#170522=CARTESIAN_POINT ( 'NONE',  ( -11.32603390678133159, 7.709074399366075525, 3.972318804447378504 ) ) ;
#170541=EDGE_CURVE ( 'NONE', #188369, #117790, #70026, .T. ) ;
#170560=LINE ( 'NONE', #22143, #6072 ) ;
#170591=CARTESIAN_POINT ( 'NONE',  ( 8.662992978453381454, 14.42103047445972308, -8.321347630537264450 ) ) ;
#170598=CARTESIAN_POINT ( 'NONE',  ( -11.89829993707161648, 13.82919228251126142, -1.561606677374349772 ) ) ;
#170621=B_SPLINE_CURVE_WITH_KNOTS ( 'NONE', 3,
 ( #45426, #162369, #161299, #145083, #96314, #208949 ),
 .UNSPECIFIED., .F., .F.,
 ( 4, 2, 4 ),
 ( 0.000000000000000000, 0.0003844267940947826553, 0.0007688535881895653106 ),
 .UNSPECIFIED. ) ;
#170633=CARTESIAN_POINT ( 'NONE',  ( -10.50659947519749693, 5.359800460605414152, -5.105385958519358169 ) ) ;
#170635=VECTOR ( 'NONE', #89672, 1000.000000000000000 ) ;
#170643=FILL_AREA_STYLE ('',( #124129 ) ) ;
#170661=CARTESIAN_POINT ( 'NONE',  ( -15.75000000000000000, 10.90000000000000036, -1.100000000000002087 ) ) ;
#170695=CARTESIAN_POINT ( 'NONE',  ( -11.01135777277262129, 0.000000000000000000, 1.399999999999998579 ) ) ;
#170713=EDGE_CURVE ( 'NONE', #71097, #147625, #145694, .T. ) ;
#170727=AXIS2_PLACEMENT_3D ( 'NONE', #153148, #207224, #108736 ) ;
#170729=STYLED_ITEM ( 'NONE', ( #144626 ), #55927 ) ;
#170736=ORIENTED_EDGE ( 'NONE', *, *, #108972, .T. ) ;
#170742=AXIS2_PLACEMENT_3D ( 'NONE', #87792, #54229, #43075 ) ;
#170745=CARTESIAN_POINT ( 'NONE',  ( -10.37923916842784422, 4.890109552615133026, -5.358306740738790097 ) ) ;
#170754=CARTESIAN_POINT ( 'NONE',  ( -10.99878419127389684, 6.872217442641685103, 3.961452310287494338 ) ) ;
#170760=CARTESIAN_POINT ( 'NONE',  ( 11.08329605692676623, 7.955792042383879270, 4.620896497113651691 ) ) ;
#170771=B_SPLINE_CURVE_WITH_KNOTS ( 'NONE', 3,
 ( #164050, #130547, #97992, #81716, #31914, #13509 ),
 .UNSPECIFIED., .F., .F.,
 ( 4, 2, 4 ),
 ( 0.000000000000000000, 0.0003172254002810696557, 0.0006344508005621393113 ),
 .UNSPECIFIED. ) ;
#170779=CARTESIAN_POINT ( 'NONE',  ( -9.356506676016417501, 15.43424542432546787, 7.432410969269082734 ) ) ;
#170782=CARTESIAN_POINT ( 'NONE',  ( -5.580126084947876208, 15.44693018518439054, -10.58314212524266296 ) ) ;
#170797=PRESENTATION_STYLE_ASSIGNMENT (( #104749 ) ) ;
#170826=DIRECTION ( 'NONE',  ( 0.000000000000000000, 0.000000000000000000, 1.000000000000000000 ) ) ;
#170830=CARTESIAN_POINT ( 'NONE',  ( -11.66942904513850543, 4.336835040752899495, -5.185078083676367910 ) ) ;
#170836=EDGE_LOOP ( 'NONE', ( #49925, #191678, #173728, #91417 ) ) ;
#170855=CYLINDRICAL_SURFACE ( 'NONE', #68301, 0.3999999999999996891 ) ;
#170910=ORIENTED_EDGE ( 'NONE', *, *, #174500, .T. ) ;
#170925=FILL_AREA_STYLE ('',( #23598 ) ) ;
#170940=CYLINDRICAL_SURFACE ( 'NONE', #16322, 0.3999999999999996336 ) ;
#170987=ORIENTED_EDGE ( 'NONE', *, *, #139910, .T. ) ;
#171010=CARTESIAN_POINT ( 'NONE',  ( -11.89317557362571698, 9.837241561624070485, 1.599935658896036283 ) ) ;
#171025=SURFACE_STYLE_USAGE ( .BOTH. , #5290 ) ;
#171026=CARTESIAN_POINT ( 'NONE',  ( -10.96276904610368597, 4.385383195573210102, 6.374211443005175504 ) ) ;
#171051=CARTESIAN_POINT ( 'NONE',  ( 0.000000000000000000, 3.481540744127368914, 0.000000000000000000 ) ) ;
#171052=CARTESIAN_POINT ( 'NONE',  ( -8.804383207025272995, 15.51845922978708181, -8.203328898748138087 ) ) ;
#171071=PRESENTATION_STYLE_ASSIGNMENT (( #137530 ) ) ;
#171072=CARTESIAN_POINT ( 'NONE',  ( -11.04536101718726293, 12.69999999999999929, 1.099999999999996758 ) ) ;
#171086=EDGE_CURVE ( 'NONE', #31644, #95942, #117539, .T. ) ;
#171089=CIRCLE ( 'NONE', #133100, 11.92000000000000171 ) ;
#171095=AXIS2_PLACEMENT_3D ( 'NONE', #117292, #34894, #184349 ) ;
#171123=CARTESIAN_POINT ( 'NONE',  ( -4.767792892813339733, 15.51850240610817444, 11.02130865604331689 ) ) ;
#171133=CARTESIAN_POINT ( 'NONE',  ( -11.89942855770814134, 9.799999999999998934, -0.7000000000000009548 ) ) ;
#171146=AXIS2_PLACEMENT_3D ( 'NONE', #15039, #36636, #148279 ) ;
#171161=CYLINDRICAL_SURFACE ( 'NONE', #85642, 0.3999999999999993006 ) ;
#171171=LINE ( 'NONE', #184210, #37065 ) ;
#171172=CARTESIAN_POINT ( 'NONE',  ( -10.14895191633106819, 2.999999999999999112, 7.601392964450658596 ) ) ;
#171181=ORIENTED_EDGE ( 'NONE', *, *, #161821, .F. ) ;
#171225=ADVANCED_FACE ( 'NONE', ( #102284 ), #181405, .F. ) ;
#171228=CARTESIAN_POINT ( 'NONE',  ( -11.88168509644349058, 9.719999999999982876, 1.685788023084328513 ) ) ;
#171251=DIRECTION ( 'NONE',  ( 0.000000000000000000, 0.000000000000000000, 1.000000000000000000 ) ) ;
#171286=FILL_AREA_STYLE_COLOUR ( '', #71373 ) ;
#171292=DIRECTION ( 'NONE',  ( -0.2275915169919967007, 0.8825604524983418075, -0.4114476261679050340 ) ) ;
#171306=CARTESIAN_POINT ( 'NONE',  ( -11.19349454483825212, 5.612381422204108183, 3.868266946477203927 ) ) ;
#171321=ORIENTED_EDGE ( 'NONE', *, *, #76523, .T. ) ;
#171330=CARTESIAN_POINT ( 'NONE',  ( -11.00605293250196226, 9.990747386415566922, -1.443095658425808114 ) ) ;
#171367=EDGE_CURVE ( 'NONE', #188409, #130695, #7392, .T. ) ;
#171372=CARTESIAN_POINT ( 'NONE',  ( -1.271070482942027180, 8.436788551174039696, -10.93994114196923384 ) ) ;
#171403=FACE_OUTER_BOUND ( 'NONE', #139372, .T. ) ;
#171405=CIRCLE ( 'NONE', #19094, 0.5000000000000015543 ) ;
#171421=CARTESIAN_POINT ( 'NONE',  ( 8.874816357151750879, 14.67092918096089527, 8.013384896292299331 ) ) ;
#171434=DIRECTION ( 'NONE',  ( 0.000000000000000000, 0.000000000000000000, -1.000000000000000000 ) ) ;
#171442=CARTESIAN_POINT ( 'NONE',  ( 10.51595811585101004, 12.48659653991854945, -3.553980774159643197 ) ) ;
#171447=VECTOR ( 'NONE', #59968, 1000.000000000000000 ) ;
#171518=FACE_OUTER_BOUND ( 'NONE', #148138, .T. ) ;
#171536=CARTESIAN_POINT ( 'NONE',  ( -11.44779965693221335, 10.99686076798700007, -3.599999932276613190 ) ) ;
#171545=CARTESIAN_POINT ( 'NONE',  ( 9.427850895902817996, 13.54474674066948481, 7.423989997610750180 ) ) ;
#171566=CARTESIAN_POINT ( 'NONE',  ( -5.601522619460554075, 14.48156018096324971, -10.62176275871059694 ) ) ;
#171583=CARTESIAN_POINT ( 'NONE',  ( -0.06840433871349645145, 15.50637188434422420, 11.99962847080720074 ) ) ;
#171636=ORIENTED_EDGE ( 'NONE', *, *, #82182, .T. ) ;
#171646=ORIENTED_EDGE ( 'NONE', *, *, #184187, .F. ) ;
#171659=EDGE_CURVE ( 'NONE', #181928, #188409, #35070, .T. ) ;
#171661=CARTESIAN_POINT ( 'NONE',  ( 11.18117232051588594, 8.274016526874332200, -4.422333253022389776 ) ) ;
#171688=CARTESIAN_POINT ( 'NONE',  ( 11.94980361058169116, 10.19999999999999929, 1.099999999999994982 ) ) ;
#171701=CARTESIAN_POINT ( 'NONE',  ( -11.80098439192703097, 4.809115636342174760, 4.927210371565812430 ) ) ;
#171743=FACE_BOUND ( 'NONE', #192737, .T. ) ;
#171746=MECHANICAL_DESIGN_GEOMETRIC_PRESENTATION_REPRESENTATION('',(#202798),#140563);
#171782=LINE ( 'NONE', #104663, #89467 ) ;
#171794=EDGE_CURVE ( 'NONE', #202127, #213959, #414, .T. ) ;
#171810=EDGE_CURVE ( 'NONE', #30835, #163314, #121607, .T. ) ;
#171811=ORIENTED_EDGE ( 'NONE', *, *, #78415, .T. ) ;
#171825=CARTESIAN_POINT ( 'NONE',  ( -10.07159190936562432, 5.946254181132138328, -5.792974557957699666 ) ) ;
#171829=VERTEX_POINT ( 'NONE', #56745 ) ;
#171830=VECTOR ( 'NONE', #28496, 1000.000000000000000 ) ;
#171832=CARTESIAN_POINT ( 'NONE',  ( 8.433927911510377129, 13.95651121305023601, 8.536819633252605399 ) ) ;
#171854=ORIENTED_EDGE ( 'NONE', *, *, #191572, .T. ) ;
#171901=CARTESIAN_POINT ( 'NONE',  ( -9.707245187965476418, 5.109025436760802563, -6.475459982491707400 ) ) ;
#171909=ORIENTED_EDGE ( 'NONE', *, *, #33178, .F. ) ;
#171914=AXIS2_PLACEMENT_3D ( 'NONE', #199971, #51619, #68893 ) ;
#171924=LINE ( 'NONE', #92831, #29852 ) ;
#171944=B_SPLINE_CURVE_WITH_KNOTS ( 'NONE', 3,
 ( #136589, #143821, #177348, #91853, #92916, #61453, #86756, #59320, #125477, #54263, #109218, #120399, #186374, #104083, #21715, #163234 ),
 .UNSPECIFIED., .F., .F.,
 ( 4, 2, 2, 2, 2, 2, 2, 4 ),
 ( 0.000000000000000000, 0.001339152797105230700, 0.002678305594210461400, 0.004017458391315694051, 0.005356611188420927136, 0.006695763985526160221, 0.008034916782631393306, 0.01071322237684185948 ),
 .UNSPECIFIED. ) ;
#171967=DIRECTION ( 'NONE',  ( 0.6250000000000057732, 7.952367169259533937E-16, 0.7806247497997951257 ) ) ;
#171988=CARTESIAN_POINT ( 'NONE',  ( -15.75000000000000000, 13.40000000000000036, -1.400000000000001910 ) ) ;
#171997=( NAMED_UNIT ( * ) SI_UNIT ( $, .STERADIAN. ) SOLID_ANGLE_UNIT ( ) );
#172007=CARTESIAN_POINT ( 'NONE',  ( 11.94980361058169116, 10.89999999999999858, 1.099999999999994982 ) ) ;
#172014=B_SPLINE_CURVE_WITH_KNOTS ( 'NONE', 3,
 ( #128769, #213113, #179578, #97274, #208848, #210980 ),
 .UNSPECIFIED., .F., .F.,
 ( 4, 2, 4 ),
 ( 0.001251957608719239234, 0.001565178843344208022, 0.001878400077969176376 ),
 .UNSPECIFIED. ) ;
#172030=B_SPLINE_CURVE_WITH_KNOTS ( 'NONE', 3,
 ( #50104, #53297, #186488, #116224, #182216, #17567 ),
 .UNSPECIFIED., .F., .F.,
 ( 4, 2, 4 ),
 ( 0.000000000000000000, 0.0003239988925529258120, 0.0006479977851058516241 ),
 .UNSPECIFIED. ) ;
#172053=DIRECTION ( 'NONE',  ( 1.000000000000000000, -0.000000000000000000, -0.000000000000000000 ) ) ;
#172084=COLOUR_RGB ( '', 0.66274510, 0.83137255, 0.94901961) ;
#172106=CARTESIAN_POINT ( 'NONE',  ( 0.006200025029510404170, 14.55606717504231362, 11.95073768095064004 ) ) ;
#172108=CARTESIAN_POINT ( 'NONE',  ( -9.915825940873133959, 4.173851563286998356, 6.175246223022227809 ) ) ;
#172135=CARTESIAN_POINT ( 'NONE',  ( -5.600682673023330338, 15.51843887165996705, -10.62222671273976538 ) ) ;
#172161=CARTESIAN_POINT ( 'NONE',  ( -6.730388996436583504, 14.55213502910268453, 9.891260588912654583 ) ) ;
#172174=SURFACE_STYLE_USAGE ( .BOTH. , #106150 ) ;
#172178=CARTESIAN_POINT ( 'NONE',  ( -11.94105721237523277, 10.90000000000000036, 1.187919463087245386 ) ) ;
#172207=CARTESIAN_POINT ( 'NONE',  ( -11.33772463945037146, 10.19999999999998153, 3.599999999999999201 ) ) ;
#172216=VERTEX_POINT ( 'NONE', #178404 ) ;
#172246=FILL_AREA_STYLE ('',( #8657 ) ) ;
#172254=CARTESIAN_POINT ( 'NONE',  ( -9.420034542028389524, 2.999999999999999556, 6.906487091023606695 ) ) ;
#172272=EDGE_LOOP ( 'NONE', ( #126412, #185292, #124287, #111191 ) ) ;
#172293=CARTESIAN_POINT ( 'NONE',  ( 11.89942855770813956, 13.79999999999999893, 0.6999999999999992895 ) ) ;
#172302=CARTESIAN_POINT ( 'NONE',  ( -8.762930527791271018, 14.55305236194923602, 8.184482591177637545 ) ) ;
#172307=CARTESIAN_POINT ( 'NONE',  ( 11.87828357750012209, 12.29689747259587129, 1.708055325888913289 ) ) ;
#172327=ORIENTED_EDGE ( 'NONE', *, *, #22937, .T. ) ;
#172338=AXIS2_PLACEMENT_3D ( 'NONE', #136481, #56287, #202504 ) ;
#172355=B_SPLINE_CURVE_WITH_KNOTS ( 'NONE', 3,
 ( #176307, #78781, #156862, #143844, #28983, #95069 ),
 .UNSPECIFIED., .F., .F.,
 ( 4, 2, 4 ),
 ( 0.000000000000000000, 0.0003168911866439334617, 0.0006337823732878669234 ),
 .UNSPECIFIED. ) ;
#172369=CARTESIAN_POINT ( 'NONE',  ( 11.43195036480942051, 9.944755037147421817, -3.649565797774410036 ) ) ;
#172372=ORIENTED_EDGE ( 'NONE', *, *, #69227, .F. ) ;
#172384=COLOUR_RGB ( '', 0.66274510, 0.83137255, 0.94901961) ;
#172390=CARTESIAN_POINT ( 'NONE',  ( -11.69243366784185945, 8.407932920124673970, 1.097391832464843286 ) ) ;
#172392=CARTESIAN_POINT ( 'NONE',  ( -11.44779963594988814, 10.19999999999998153, 3.600000000000001421 ) ) ;
#172406=VERTEX_POINT ( 'NONE', #113463 ) ;
#172407=CARTESIAN_POINT ( 'NONE',  ( 1.469576158976824144E-15, 4.518459255872630642, 12.00000000000000178 ) ) ;
#172416=MECHANICAL_DESIGN_GEOMETRIC_PRESENTATION_REPRESENTATION('',(#168987),#127506);
#172418=CARTESIAN_POINT ( 'NONE',  ( -15.75000000000000000, 13.79999999999999893, -1.800000000000001155 ) ) ;
#172458=CARTESIAN_POINT ( 'NONE',  ( 11.44789321844504215, 9.799999999999982947, 3.303298730975393838 ) ) ;
#172486=( NAMED_UNIT ( * ) PLANE_ANGLE_UNIT ( ) SI_UNIT ( $, .RADIAN. ) );
#172502=CARTESIAN_POINT ( 'NONE',  ( 8.384960142880849787, 15.11786449873486582, 8.585919489561741003 ) ) ;
#172507=DIRECTION ( 'NONE',  ( 0.000000000000000000, -1.000000000000000000, -9.023263958591317418E-17 ) ) ;
#172513=ORIENTED_EDGE ( 'NONE', *, *, #195893, .F. ) ;
#172523=CIRCLE ( 'NONE', #193376, 11.09999999999999964 ) ;
#172565=CARTESIAN_POINT ( 'NONE',  ( -5.601522606845680485, 14.48156018084685925, -10.62176276536360398 ) ) ;
#172584=B_SPLINE_CURVE_WITH_KNOTS ( 'NONE', 3,
 ( #63711, #162290, #195852, #31226, #148177, #115718, #97300, #17070, #127750, #193707, #166548, #202216, #52791, #118930, #36534, #102621 ),
 .UNSPECIFIED., .F., .F.,
 ( 4, 2, 2, 2, 2, 2, 2, 4 ),
 ( 0.000000000000000000, 8.859500144023226638E-05, 0.0001771900028804645328, 0.0003543800057609234819, 0.0007087600115218431690, 0.001063140017282762856, 0.001240330020163218959, 0.001417520023043675279 ),
 .UNSPECIFIED. ) ;
#172606=DIRECTION ( 'NONE',  ( 0.6249999999996046496, -1.550603090070706853E-14, -0.7806247498001163132 ) ) ;
#172615=CARTESIAN_POINT ( 'NONE',  ( -11.86145017354119879, 12.59514365543876124, 1.099999999999996980 ) ) ;
#172633=EDGE_CURVE ( 'NONE', #159273, #121309, #123090, .T. ) ;
#172642=( LENGTH_UNIT ( ) NAMED_UNIT ( * ) SI_UNIT ( .MILLI., .METRE. ) );
#172643=DIRECTION ( 'NONE',  ( -0.000000000000000000, -1.000000000000000000, -0.000000000000000000 ) ) ;
#172654=CARTESIAN_POINT ( 'NONE',  ( 11.69539920569646618, 6.979297235929839083, 4.155077259296042769 ) ) ;
#172657=ORIENTED_EDGE ( 'NONE', *, *, #117363, .T. ) ;
#172658=CARTESIAN_POINT ( 'NONE',  ( -11.35569630219380777, 9.987315607086337366, -3.554478010595065296 ) ) ;
#172668=CARTESIAN_POINT ( 'NONE',  ( 9.367496997597635655, 4.469082183885419113, -7.499999999999953815 ) ) ;
#172678=SURFACE_STYLE_USAGE ( .BOTH. , #105556 ) ;
#172706=FACE_OUTER_BOUND ( 'NONE', #194846, .T. ) ;
#172714=DIRECTION ( 'NONE',  ( 0.000000000000000000, 0.000000000000000000, 1.000000000000000000 ) ) ;
#172744=B_SPLINE_CURVE_WITH_KNOTS ( 'NONE', 3,
 ( #152951, #68475, #120529, #104211, #21843, #87951 ),
 .UNSPECIFIED., .F., .F.,
 ( 4, 2, 4 ),
 ( 0.001279092382393100377, 0.001599469101539997178, 0.001919845820686893979 ),
 .UNSPECIFIED. ) ;
#172751=CARTESIAN_POINT ( 'NONE',  ( 0.000000000000000000, 3.999999999999996447, 0.000000000000000000 ) ) ;
#172758=CARTESIAN_POINT ( 'NONE',  ( 7.449721630645223414, 15.00158243878686726, 10.26201403118819044 ) ) ;
#172781=TOROIDAL_SURFACE ( 'NONE', #117479, -0.1799999999926198968, 0.5000000000000013323 ) ;
#172793=CARTESIAN_POINT ( 'NONE',  ( -10.87631885467295945, 5.775928357311673089, -6.414435785039473537 ) ) ;
#172797=CARTESIAN_POINT ( 'NONE',  ( -11.01135777277262129, 12.69999999999999929, -1.400000000000001910 ) ) ;
#172800=CARTESIAN_POINT ( 'NONE',  ( 11.00592705432737972, 11.11019307346892759, 1.444010445236424856 ) ) ;
#172802=ORIENTED_EDGE ( 'NONE', *, *, #95954, .T. ) ;
#172807=LINE ( 'NONE', #191156, #48996 ) ;
#172809=CARTESIAN_POINT ( 'NONE',  ( -15.75000000000000000, 9.799999999999998934, -1.800000000000001155 ) ) ;
#172813=ORIENTED_EDGE ( 'NONE', *, *, #51382, .T. ) ;
#172827=( GEOMETRIC_REPRESENTATION_CONTEXT ( 3 ) GLOBAL_UNCERTAINTY_ASSIGNED_CONTEXT ( ( #133888 ) ) GLOBAL_UNIT_ASSIGNED_CONTEXT ( ( #81990, #128706, #31134 ) ) REPRESENTATION_CONTEXT ( 'NONE', 'WORKASPACE' ) );
#172873=CARTESIAN_POINT ( 'NONE',  ( -9.333041836230696831, 14.55305236563169302, -7.472413793098840351 ) ) ;
#172887=EDGE_LOOP ( 'NONE', ( #54485, #212918, #37094, #122784 ) ) ;
#172902=ADVANCED_FACE ( 'NONE', ( #1405 ), #17660, .F. ) ;
#172911=CARTESIAN_POINT ( 'NONE',  ( -10.87631885467295945, 5.775928357311673089, -6.414435785039473537 ) ) ;
#172917=CARTESIAN_POINT ( 'NONE',  ( 8.730775170176714894, 13.51259826081505899, 8.232739887797778877 ) ) ;
#172929=( NAMED_UNIT ( * ) SI_UNIT ( $, .STERADIAN. ) SOLID_ANGLE_UNIT ( ) );
#172932=CARTESIAN_POINT ( 'NONE',  ( -11.86239285000045918, 12.29999999999997939, 1.812080536912751283 ) ) ;
#172986=CARTESIAN_POINT ( 'NONE',  ( -11.23979429089589033, 4.930458577253933328, -5.866063493660276684 ) ) ;
#173010=DIRECTION ( 'NONE',  ( 0.000000000000000000, 0.000000000000000000, -1.000000000000000000 ) ) ;
#173049=CARTESIAN_POINT ( 'NONE',  ( 10.37944572521833742, 9.120024990325399372, 6.075587282785552823 ) ) ;
#173058=DIRECTION ( 'NONE',  ( -0.000000000000000000, 0.000000000000000000, -1.000000000000000000 ) ) ;
#173071=ORIENTED_EDGE ( 'NONE', *, *, #137433, .F. ) ;
#173075=SURFACE_STYLE_FILL_AREA ( #154678 ) ;
#173084=CARTESIAN_POINT ( 'NONE',  ( -15.75000000000000000, 13.40000000000000036, -0.7000000000000009548 ) ) ;
#173104=CARTESIAN_POINT ( 'NONE',  ( 11.33772463945036790, 12.69999999999999929, -3.600000000000000977 ) ) ;
#173114=CARTESIAN_POINT ( 'NONE',  ( 11.48784849554594345, 9.769504728180750774, 3.469614872287801521 ) ) ;
#173118=ADVANCED_FACE ( 'NONE', ( #171403 ), #141086, .F. ) ;
#173123=SURFACE_STYLE_USAGE ( .BOTH. , #40989 ) ;
#173138=EDGE_CURVE ( 'NONE', #188369, #210693, #83632, .T. ) ;
#173182=VERTEX_POINT ( 'NONE', #59788 ) ;
#173185=FILL_AREA_STYLE ('',( #88731 ) ) ;
#173186=CARTESIAN_POINT ( 'NONE',  ( -11.30310531956832598, 5.150576456239967627, 5.742040133384030298 ) ) ;
#173214=DIRECTION ( 'NONE',  ( 0.000000000000000000, 7.228014483236694583E-17, -1.000000000000000000 ) ) ;
#173220=ORIENTED_EDGE ( 'NONE', *, *, #136253, .T. ) ;
#173243=CARTESIAN_POINT ( 'NONE',  ( 0.000000000000000000, 7.980384757729337863, 0.000000000000000000 ) ) ;
#173248=( LENGTH_UNIT ( ) NAMED_UNIT ( * ) SI_UNIT ( .MILLI., .METRE. ) );
#173252=PLANE ( 'NONE',  #187949 ) ;
#173255=CARTESIAN_POINT ( 'NONE',  ( -10.18412789821966413, 3.641746037092307819, 6.362472743772858763 ) ) ;
#173258=VERTEX_POINT ( 'NONE', #195126 ) ;
#173265=CARTESIAN_POINT ( 'NONE',  ( -11.04985331135689108, 11.10920893529997855, 1.056514597312212755 ) ) ;
#173281=DIRECTION ( 'NONE',  ( 0.000000000000000000, 0.000000000000000000, -1.000000000000000000 ) ) ;
#173290=EDGE_LOOP ( 'NONE', ( #202238, #92434, #8233, #5039, #206880, #132932, #131426, #117286 ) ) ;
#173298=EDGE_CURVE ( 'NONE', #52465, #164408, #130200, .T. ) ;
#173301=EDGE_CURVE ( 'NONE', #193391, #77381, #156322, .T. ) ;
#173304=AXIS2_PLACEMENT_3D ( 'NONE', #90156, #21896, #202792 ) ;
#173330=CARTESIAN_POINT ( 'NONE',  ( -10.57368757801325820, 3.061359382655743033, 7.009609602318408683 ) ) ;
#173379=CARTESIAN_POINT ( 'NONE',  ( -6.689742616953707532, 14.55216527438033225, 9.919101817088241901 ) ) ;
#173383=CARTESIAN_POINT ( 'NONE',  ( 9.305047017613608418, 3.481540744127370690, -7.450000000000005507 ) ) ;
#173388=CARTESIAN_POINT ( 'NONE',  ( -11.92045683181315674, 9.947240721205131919, 1.382340670101856350 ) ) ;
#173402=VECTOR ( 'NONE', #87104, 1000.000000000000000 ) ;
#173403=DIRECTION ( 'NONE',  ( 0.000000000000000000, 1.000000000000000000, 0.000000000000000000 ) ) ;
#173429=DIRECTION ( 'NONE',  ( -0.000000000000000000, 1.000000000000000000, -0.000000000000000000 ) ) ;
#173451=CARTESIAN_POINT ( 'NONE',  ( 0.000000000000000000, 3.553060279300227275, 0.000000000000000000 ) ) ;
#173456=VERTEX_POINT ( 'NONE', #14208 ) ;
#173472=CARTESIAN_POINT ( 'NONE',  ( -10.57232049882948388, 5.599334429189661400, -4.968988939937085014 ) ) ;
#173473=AXIS2_PLACEMENT_3D ( 'NONE', #136903, #172606, #152081 ) ;
#173474=ADVANCED_FACE ( 'NONE', ( #85627 ), #170217, .T. ) ;
#173493=ORIENTED_EDGE ( 'NONE', *, *, #125681, .T. ) ;
#173494=CARTESIAN_POINT ( 'NONE',  ( -10.62873463776380056, 13.79999999999999893, -3.200000000000001510 ) ) ;
#173498=CARTESIAN_POINT ( 'NONE',  ( -11.41381678389388377, 13.52879418241074561, -3.704697885617973530 ) ) ;
#173507=DIRECTION ( 'NONE',  ( 0.000000000000000000, 0.000000000000000000, -1.000000000000000000 ) ) ;
#173523=DIRECTION ( 'NONE',  ( 0.000000000000000000, -1.000000000000000000, -0.000000000000000000 ) ) ;
#173529=CARTESIAN_POINT ( 'NONE',  ( -11.04536101718726293, 0.000000000000000000, 1.099999999999996758 ) ) ;
#173534=ORIENTED_EDGE ( 'NONE', *, *, #120795, .F. ) ;
#173564=ORIENTED_EDGE ( 'NONE', *, *, #128408, .F. ) ;
#173565=FACE_OUTER_BOUND ( 'NONE', #185391, .T. ) ;
#173608=CARTESIAN_POINT ( 'NONE',  ( -1.878313713275499675, 13.99999999999846167, -12.68000002627077905 ) ) ;
#173649=CARTESIAN_POINT ( 'NONE',  ( -10.78237064342727791, 6.270194388237658956, -4.501389708959286473 ) ) ;
#173652=CARTESIAN_POINT ( 'NONE',  ( 0.000000000000000000, 15.51845925587262798, 0.000000000000000000 ) ) ;
#173653=CARTESIAN_POINT ( 'NONE',  ( -4.779943825041865324, 14.55303459918272679, -10.96777621109715462 ) ) ;
#173654=CARTESIAN_POINT ( 'NONE',  ( -11.89942855770814134, 9.799999999999998934, -0.7000000000000009548 ) ) ;
#173658=CARTESIAN_POINT ( 'NONE',  ( -11.48243876534946040, 13.79999999999999893, -3.200000000000001510 ) ) ;
#173690=( NAMED_UNIT ( * ) SI_UNIT ( $, .STERADIAN. ) SOLID_ANGLE_UNIT ( ) );
#173700=ADVANCED_FACE ( 'NONE', ( #32449 ), #83309, .T. ) ;
#173711=DIRECTION ( 'NONE',  ( 0.000000000000000000, 0.4363663110634622977, 0.8997691051424613340 ) ) ;
#173713=AXIS2_PLACEMENT_3D ( 'NONE', #186310, #152757, #135456 ) ;
#173724=CARTESIAN_POINT ( 'NONE',  ( -11.35569630219380777, 13.61268439291364274, 3.554478010595060411 ) ) ;
#173725=DIRECTION ( 'NONE',  ( 0.2684563758389248433, 0.000000000000000000, -0.9632918427306597087 ) ) ;
#173728=ORIENTED_EDGE ( 'NONE', *, *, #50025, .F. ) ;
#173735=CARTESIAN_POINT ( 'NONE',  ( 9.053228077256719075, 12.24160320938252333, 7.401071681518285317 ) ) ;
#173739=APPLICATION_CONTEXT ( 'automotive_design' ) ;
#173763=CARTESIAN_POINT ( 'NONE',  ( -11.63101921567910324, 8.358080680206626312, -2.966213382291108758 ) ) ;
#173794=CARTESIAN_POINT ( 'NONE',  ( -9.348561386651960348, 4.000000000000000888, 7.001914024036570261 ) ) ;
#173809=ORIENTED_EDGE ( 'NONE', *, *, #70476, .T. ) ;
#173823=PRESENTATION_STYLE_ASSIGNMENT (( #174888 ) ) ;
#173839=CARTESIAN_POINT ( 'NONE',  ( 8.738814790737972515, 15.13806168530491902, 7.596998062084875158 ) ) ;
#173864=CARTESIAN_POINT ( 'NONE',  ( -15.75000000000000000, 12.29999999999998295, 3.199999999999997957 ) ) ;
#173872=EDGE_CURVE ( 'NONE', #211004, #33851, #23193, .T. ) ;
#173875=CARTESIAN_POINT ( 'NONE',  ( -11.15867860892636365, 6.757705308438493041, -5.812542620506402358 ) ) ;
#173903=CARTESIAN_POINT ( 'NONE',  ( 10.24561425425348382, 10.82119614928647877, 6.253163089680928266 ) ) ;
#173917=CARTESIAN_POINT ( 'NONE',  ( -11.97929049433705373, 11.37999999999999901, 0.7046979865771783036 ) ) ;
#173918=( BOUNDED_SURFACE ( )  B_SPLINE_SURFACE ( 3, 2, ( 
 ( #166754, #33545, #201350 ),
 ( #164619, #199221, #67080 ),
 ( #213345, #82286, #49799 ),
 ( #116990, #182990, #115925 ),
 ( #118065, #34607, #133215 ),
 ( #113813, #17273, #131122 ) ),
 .UNSPECIFIED., .F., .F., .T. ) 
 B_SPLINE_SURFACE_WITH_KNOTS ( ( 4, 2, 4 ),
 ( 3, 3 ),
 ( 0.000000000000000000, 0.0003766405729503174787, 0.0007532811459006349573 ),
 ( 0.000000000000000000, 1.000000000000000000 ),
 .UNSPECIFIED. ) 
 GEOMETRIC_REPRESENTATION_ITEM ( )  RATIONAL_B_SPLINE_SURFACE ( (
 ( 1.000000000000000000, 0.7071067811865551223, 1.000000000000000000),
 ( 1.000000000000000000, 0.7211294902953824248, 1.000000000000000000),
 ( 1.000000000000000000, 0.7311181975230335306, 1.000000000000000000),
 ( 1.000000000000000000, 0.7429553055061443034, 1.000000000000000000),
 ( 1.000000000000000000, 0.7451698531058310593, 1.000000000000000000),
 ( 1.000000000000000000, 0.7452309222762957264, 1.000000000000000000) ) ) 
 REPRESENTATION_ITEM ( '' )  SURFACE ( )  );
#173960=CARTESIAN_POINT ( 'NONE',  ( 11.92619526913699879, 10.19999999999998153, 1.328859060402684644 ) ) ;
#173974=VERTEX_POINT ( 'NONE', #4178 ) ;
#173983=CARTESIAN_POINT ( 'NONE',  ( -9.917242840447775265, 4.174869238508773783, -6.172972641688763140 ) ) ;
#173988=EDGE_CURVE ( 'NONE', #79400, #152913, #212223, .T. ) ;
#173993=CARTESIAN_POINT ( 'NONE',  ( -12.36781821011106963, 9.649948393628900334, 1.413879826568002152 ) ) ;
#173998=( LENGTH_UNIT ( ) NAMED_UNIT ( * ) SI_UNIT ( .MILLI., .METRE. ) );
#174010=FILL_AREA_STYLE ('',( #206466 ) ) ;
#174032=( NAMED_UNIT ( * ) SI_UNIT ( $, .STERADIAN. ) SOLID_ANGLE_UNIT ( ) );
#174041=ORIENTED_EDGE ( 'NONE', *, *, #61508, .T. ) ;
#174060=CARTESIAN_POINT ( 'NONE',  ( -11.33772463945036968, 10.19999999999999929, -3.680000000000002824 ) ) ;
#174064=CARTESIAN_POINT ( 'NONE',  ( -11.69084473744764097, 4.401359152538248054, -5.144113628910231384 ) ) ;
#174073=CARTESIAN_POINT ( 'NONE',  ( 11.33772463945037146, 10.89999999999998259, 3.599999999999999201 ) ) ;
#174081=ORIENTED_EDGE ( 'NONE', *, *, #163457, .T. ) ;
#174095=CIRCLE ( 'NONE', #208676, 0.07999999999999998779 ) ;
#174131=CARTESIAN_POINT ( 'NONE',  ( 11.83929459711652932, 6.804233087161206228, -1.971914732669066472 ) ) ;
#174164=CARTESIAN_POINT ( 'NONE',  ( 11.95359438121989371, 11.10421899708699200, 1.059536798430487314 ) ) ;
#174183=( NAMED_UNIT ( * ) SI_UNIT ( $, .STERADIAN. ) SOLID_ANGLE_UNIT ( ) );
#174192=CARTESIAN_POINT ( 'NONE',  ( 11.52901446936746588, 9.805744725324114341, 3.330874149801137829 ) ) ;
#174229=COLOUR_RGB ( '', 0.66274510, 0.83137255, 0.94901961) ;
#174232=CARTESIAN_POINT ( 'NONE',  ( -11.04536101718726293, 10.90000000000000036, -1.100000000000002087 ) ) ;
#174253=DIRECTION ( 'NONE',  ( 0.000000000000000000, 0.000000000000000000, -1.000000000000000000 ) ) ;
#174259=CARTESIAN_POINT ( 'NONE',  ( -10.67000816626867810, 5.238978589329153834, 6.814456324518622488 ) ) ;
#174304=DIRECTION ( 'NONE',  ( 0.000000000000000000, 0.000000000000000000, 1.000000000000000000 ) ) ;
#174310=CARTESIAN_POINT ( 'NONE',  ( -8.120005463787672184, 14.55205930359461242, 8.786303532376779302 ) ) ;
#174316=CARTESIAN_POINT ( 'NONE',  ( 10.62873463776380056, 9.799999999999982947, 3.199999999999997957 ) ) ;
#174353=CARTESIAN_POINT ( 'NONE',  ( -5.556597592091960358, 15.44691531748820168, 10.59560191213078717 ) ) ;
#174367=CARTESIAN_POINT ( 'NONE',  ( 11.92619526913699524, 11.02780024161490324, -1.328859060402685976 ) ) ;
#174368=CARTESIAN_POINT ( 'NONE',  ( 11.22789937895645096, 8.808731784781956620, -4.106656770659993683 ) ) ;
#174372=CARTESIAN_POINT ( 'NONE',  ( 11.88168329227127096, 12.21999999999998288, 1.685799833707125606 ) ) ;
#174378=ORIENTED_EDGE ( 'NONE', *, *, #43445, .F. ) ;
#174391=CARTESIAN_POINT ( 'NONE',  ( 11.80248046418316044, 11.29999999999998117, 1.695421849633139466 ) ) ;
#174404=UNCERTAINTY_MEASURE_WITH_UNIT (LENGTH_MEASURE( 1.000000000000000082E-05 ), #188796, 'distance_accuracy_value', 'NONE');
#174417=SURFACE_STYLE_FILL_AREA ( #170113 ) ;
#174429=DIRECTION ( 'NONE',  ( -0.2684563758389304500, 0.000000000000000000, -0.9632918427306581544 ) ) ;
#174434=VECTOR ( 'NONE', #113692, 1000.000000000000000 ) ;
#174451=CARTESIAN_POINT ( 'NONE',  ( -4.723354487065243745, 14.48146267970840384, 11.04057532931312835 ) ) ;
#174456=CARTESIAN_POINT ( 'NONE',  ( -11.88172094500854037, 11.37999994398404269, 1.685553348215819369 ) ) ;
#174459=CARTESIAN_POINT ( 'NONE',  ( -11.00593736619310725, 11.11000507135410409, -1.443925800506596469 ) ) ;
#174471=DIRECTION ( 'NONE',  ( -0.000000000000000000, -1.000000000000000000, -0.000000000000000000 ) ) ;
#174472=B_SPLINE_CURVE_WITH_KNOTS ( 'NONE', 3,
 ( #127689, #156915, #43174, #206704, #90851, #107145 ),
 .UNSPECIFIED., .F., .F.,
 ( 4, 2, 4 ),
 ( 0.000000000000000000, 0.0003239988925529257036, 0.0006479977851058514073 ),
 .UNSPECIFIED. ) ;
#174478=ORIENTED_EDGE ( 'NONE', *, *, #3774, .F. ) ;
#174485=DIRECTION ( 'NONE',  ( 1.224646797963766027E-16, -4.396526966619892032E-05, 0.9999999990335275424 ) ) ;
#174500=EDGE_CURVE ( 'NONE', #83422, #30243, #28289, .T. ) ;
#174503=CARTESIAN_POINT ( 'NONE',  ( 0.000000000000000000, 15.00000000000000000, 0.000000000000000000 ) ) ;
#174521=CARTESIAN_POINT ( 'NONE',  ( -11.81905481421901705, 9.842643443827332916, -1.592167362352180593 ) ) ;
#174523=CARTESIAN_POINT ( 'NONE',  ( -11.91826848676326378, 13.50833707238768078, -1.400000051401918855 ) ) ;
#174542=CARTESIAN_POINT ( 'NONE',  ( -11.45846087878765296, 10.00688399218595492, 3.566076377698180089 ) ) ;
#174543=CARTESIAN_POINT ( 'NONE',  ( 1.734723475976807094E-15, 14.99962766111844736, 11.68000013863625774 ) ) ;
#174566=CARTESIAN_POINT ( 'NONE',  ( -11.52888687719588745, 13.79423125105035730, -3.331331986263487366 ) ) ;
#174572=DIRECTION ( 'NONE',  ( 1.000000000000000000, -0.000000000000000000, -0.000000000000000000 ) ) ;
#174599=STYLED_ITEM ( 'NONE', ( #206772 ), #157787 ) ;
#174627=VERTEX_POINT ( 'NONE', #211969 ) ;
#174637=CIRCLE ( 'NONE', #81220, 0.08000000000000020983 ) ;
#174640=ORIENTED_EDGE ( 'NONE', *, *, #58112, .T. ) ;
#174650=CARTESIAN_POINT ( 'NONE',  ( 6.928203230275514990, 15.51887838114830309, 9.797958971132707973 ) ) ;
#174661=ORIENTED_EDGE ( 'NONE', *, *, #22794, .T. ) ;
#174663=UNCERTAINTY_MEASURE_WITH_UNIT (LENGTH_MEASURE( 1.000000000000000082E-05 ), #124382, 'distance_accuracy_value', 'NONE');
#174672=CARTESIAN_POINT ( 'NONE',  ( 11.48806469435255551, 9.769102271275494687, 3.468902948106700190 ) ) ;
#174673=ORIENTED_EDGE ( 'NONE', *, *, #169884, .F. ) ;
#174689=AXIS2_PLACEMENT_3D ( 'NONE', #3508, #102107, #39243 ) ;
#174708=ORIENTED_EDGE ( 'NONE', *, *, #146979, .F. ) ;
#174710=( BOUNDED_CURVE ( )  B_SPLINE_CURVE ( 3, ( #7519, #190542, #124582, #56296, #207860, #106161, #105065 ),
 .UNSPECIFIED., .F., .T. ) 
 B_SPLINE_CURVE_WITH_KNOTS ( ( 4, 3, 4 ),
 ( 0.001053980190856398762, 0.001563073325492780842, 0.001563600248854528623 ),
 .UNSPECIFIED. ) 
 CURVE ( )  GEOMETRIC_REPRESENTATION_ITEM ( )  RATIONAL_B_SPLINE_CURVE ( ( 0.5394211213094468604, 0.6067365765767515073, 0.7602628694736025539, 1.000000000000000000, 0.9997518664343353345, 0.9995038252240703303, 0.9992558763692048762 ) ) 
 REPRESENTATION_ITEM ( '' )  );
#174713=CARTESIAN_POINT ( 'NONE',  ( -10.78227258717170578, 6.269840026405313793, 4.500979083849748541 ) ) ;
#174724=CARTESIAN_POINT ( 'NONE',  ( -15.75000000000000000, 12.29999999999998295, 1.799999999999999600 ) ) ;
#174725=ORIENTED_EDGE ( 'NONE', *, *, #123817, .F. ) ;
#174747=B_SPLINE_CURVE_WITH_KNOTS ( 'NONE', 3,
 ( #96075, #148009, #192463, #77659 ),
 .UNSPECIFIED., .F., .F.,
 ( 4, 4 ),
 ( 0.000000000000000000, 8.045963024324400998E-05 ),
 .UNSPECIFIED. ) ;
#174756=PRESENTATION_STYLE_ASSIGNMENT (( #160612 ) ) ;
#174782=CARTESIAN_POINT ( 'NONE',  ( 9.844850794264569771, 11.91743369232944616, -6.864440167955208949 ) ) ;
#174788=COLOUR_RGB ( '', 0.31764706, 0.68627451, 0.89019608) ;
#174802=CARTESIAN_POINT ( 'NONE',  ( 12.32921881676780806, 6.000999082531765616, -1.082566570140983675 ) ) ;
#174805=VERTEX_POINT ( 'NONE', #199350 ) ;
#174816=EDGE_LOOP ( 'NONE', ( #145857, #89927, #16300, #64804, #204864, #11463 ) ) ;
#174817=CARTESIAN_POINT ( 'NONE',  ( -1.790873115444854946, 15.44822087383597875, -11.85388518076883457 ) ) ;
#174839=AXIS2_PLACEMENT_3D ( 'NONE', #135680, #2430, #68507 ) ;
#174852=ADVANCED_FACE ( 'NONE', ( #15275 ), #17396, .T. ) ;
#174860=CARTESIAN_POINT ( 'NONE',  ( 1.050790385995008513, 16.00000000000000000, 12.64745918785790302 ) ) ;
#174875=EDGE_LOOP ( 'NONE', ( #8755, #45655, #114949, #121190 ) ) ;
#174888=SURFACE_STYLE_USAGE ( .BOTH. , #108862 ) ;
#174900=CARTESIAN_POINT ( 'NONE',  ( 11.46478114675041127, 7.823431138067391544, 3.656553153322682714 ) ) ;
#174906=CARTESIAN_POINT ( 'NONE',  ( 8.493624849120759990, 15.84268045232546918, 9.435489967669033362 ) ) ;
#174938=CARTESIAN_POINT ( 'NONE',  ( -10.91435215633265621, 5.922423255477170301, -6.337208484649258899 ) ) ;
#174952=DIRECTION ( 'NONE',  ( 1.000000000000000000, -0.000000000000000000, -0.000000000000000000 ) ) ;
#174962=CARTESIAN_POINT ( 'NONE',  ( 9.501543970383670157, 13.11825151260853417, 7.330405911628732341 ) ) ;
#174971=( LENGTH_UNIT ( ) NAMED_UNIT ( * ) SI_UNIT ( .MILLI., .METRE. ) );
#174990=CARTESIAN_POINT ( 'NONE',  ( 11.06297021485807264, 9.843306985125275688, 0.9089447062504968367 ) ) ;
#174992=VECTOR ( 'NONE', #26272, 1000.000000000000000 ) ;
#175007=CARTESIAN_POINT ( 'NONE',  ( -9.367496997601184816, 15.42330868760440410, -7.413898975931886959 ) ) ;
#175023=COLOUR_RGB ( '', 0.72549020, 0.75294118, 0.79215686) ;
#175025=VERTEX_POINT ( 'NONE', #166885 ) ;
#175033=ORIENTED_EDGE ( 'NONE', *, *, #106403, .T. ) ;
#175049=CARTESIAN_POINT ( 'NONE',  ( -11.50715376448619764, 7.744667295756731740, 4.958460396591308772 ) ) ;
#175088=DIRECTION ( 'NONE',  ( 1.000000000000000000, -0.000000000000000000, -0.000000000000000000 ) ) ;
#175117=DIRECTION ( 'NONE',  ( -0.000000000000000000, -1.000000000000000000, 0.000000000000000000 ) ) ;
#175119=( BOUNDED_SURFACE ( )  B_SPLINE_SURFACE ( 3, 2, ( 
 ( #52406, #168289, #100088 ),
 ( #184516, #38287, #199698 ),
 ( #118533, #134748, #200757 ),
 ( #54537, #132623, #53466 ),
 ( #101138, #51343, #18812 ),
 ( #150986, #166149, #68625 ) ),
 .UNSPECIFIED., .F., .F., .F. ) 
 B_SPLINE_SURFACE_WITH_KNOTS ( ( 4, 2, 4 ),
 ( 3, 3 ),
 ( 0.000000000000000000, 0.0003754689591423961527, 0.0007509379182847923054 ),
 ( 0.000000000000000000, 1.000000000000000000 ),
 .UNSPECIFIED. ) 
 GEOMETRIC_REPRESENTATION_ITEM ( )  RATIONAL_B_SPLINE_SURFACE ( (
 ( 1.000000000000000000, 0.7071067811865475727, 1.000000000000000000),
 ( 1.000000000000000000, 0.7018599272024023117, 1.000000000000000000),
 ( 1.000000000000000000, 0.6927733177260293473, 1.000000000000000000),
 ( 1.000000000000000000, 0.6772007068873806546, 1.000000000000000000),
 ( 1.000000000000000000, 0.6709974581636959368, 1.000000000000000000),
 ( 1.000000000000000000, 0.6711954675835484219, 1.000000000000000000) ) ) 
 REPRESENTATION_ITEM ( '' )  SURFACE ( )  );
#175122=CARTESIAN_POINT ( 'NONE',  ( -10.24056286296518614, 5.004077596833054642, -7.476959758773280562 ) ) ;
#175134=AXIS2_PLACEMENT_3D ( 'NONE', #148621, #189, #211463 ) ;
#175138=AXIS2_PLACEMENT_3D ( 'NONE', #41651, #25367, #140226 ) ;
#175175=COLOUR_RGB ( '', 0.08235294, 0.09019608, 0.10196078) ;
#175193=ADVANCED_FACE ( 'NONE', ( #52064 ), #34727, .F. ) ;
#175204=CARTESIAN_POINT ( 'NONE',  ( -11.89829993707161471, 12.27080771748872046, 1.561606677374347552 ) ) ;
#175213=CARTESIAN_POINT ( 'NONE',  ( -15.75000000000000000, 10.90000000000000036, -1.800000000000001155 ) ) ;
#175215=DIRECTION ( 'NONE',  ( 0.05872483221476467591, 7.952201780260630618E-17, 0.9982742078614211811 ) ) ;
#175217=ORIENTED_EDGE ( 'NONE', *, *, #23157, .T. ) ;
#175222=CARTESIAN_POINT ( 'NONE',  ( 11.70600796652113829, 7.005607364824809835, -2.416925703268587355 ) ) ;
#175225=CARTESIAN_POINT ( 'NONE',  ( -10.52211811376581707, 5.354010262649191887, 5.769489279399182102 ) ) ;
#175229=CARTESIAN_POINT ( 'NONE',  ( -9.333041836230190569, 14.55305236562365145, -7.472413793097476109 ) ) ;
#175249=DIRECTION ( 'NONE',  ( 0.000000000000000000, 7.254698431505021095E-17, -1.000000000000000000 ) ) ;
#175260=CARTESIAN_POINT ( 'NONE',  ( 8.733437601049905297, 14.92147133172287354, -8.230922393287746885 ) ) ;
#175279=ORIENTED_EDGE ( 'NONE', *, *, #128500, .T. ) ;
#175283=AXIS2_PLACEMENT_3D ( 'NONE', #87022, #150973, #52394 ) ;
#175296=CARTESIAN_POINT ( 'NONE',  ( -11.92619526913699879, 12.69999999999999929, -1.328859060402686199 ) ) ;
#175311=CARTESIAN_POINT ( 'NONE',  ( 10.81425746553161460, 10.30853785568457326, -6.489671246970442731 ) ) ;
#175312=CARTESIAN_POINT ( 'NONE',  ( -10.71692179555930302, 5.308633586712264041, 6.728550107195007790 ) ) ;
#175326=CARTESIAN_POINT ( 'NONE',  ( -15.75000000000000000, 12.69999999999998153, 3.599999999999999201 ) ) ;
#175333=EDGE_CURVE ( 'NONE', #29327, #33454, #177185, .T. ) ;
#175337=STYLED_ITEM ( 'NONE', ( #183116 ), #143840 ) ;
#175345=CARTESIAN_POINT ( 'NONE',  ( -3.531379743775235003, 15.51966450452909640, -11.47742191263038336 ) ) ;
#175378=CYLINDRICAL_SURFACE ( 'NONE', #128995, 0.3999999999999997446 ) ;
#175384=VERTEX_POINT ( 'NONE', #54193 ) ;
#175428=CARTESIAN_POINT ( 'NONE',  ( 11.92046840572485777, 12.44747875205727894, 1.382231356234940867 ) ) ;
#175448=SURFACE_STYLE_USAGE ( .BOTH. , #191659 ) ;
#175451=CARTESIAN_POINT ( 'NONE',  ( 11.43209210103587914, 12.44403924016084240, -3.649125173352125273 ) ) ;
#175458=ORIENTED_EDGE ( 'NONE', *, *, #55489, .T. ) ;
#175506=CARTESIAN_POINT ( 'NONE',  ( -7.085023742657587498, 14.52988328832284814, 9.695690332251523103 ) ) ;
#175511=CARTESIAN_POINT ( 'NONE',  ( -11.87828357749969754, 11.30310252740409283, 1.708055325888841569 ) ) ;
#175512=CARTESIAN_POINT ( 'NONE',  ( 11.86239285000045740, 12.21999999999998288, 1.812080536912751283 ) ) ;
#175514=LINE ( 'NONE', #193870, #143176 ) ;
#175518=PRESENTATION_STYLE_ASSIGNMENT (( #125772 ) ) ;
#175539=CARTESIAN_POINT ( 'NONE',  ( 11.86239285000045918, 11.37999999999998302, 1.812080536912751283 ) ) ;
#175542=ORIENTED_EDGE ( 'NONE', *, *, #163282, .F. ) ;
#175551=CYLINDRICAL_SURFACE ( 'NONE', #32200, 0.07999999999999998779 ) ;
#175553=EDGE_CURVE ( 'NONE', #106547, #175025, #83778, .T. ) ;
#175596=CARTESIAN_POINT ( 'NONE',  ( 8.518320732998095224, 14.76619040281040718, 9.398253358897362020 ) ) ;
#175602=DIRECTION ( 'NONE',  ( 1.776356839400250465E-14, 0.000000000000000000, -1.000000000000000000 ) ) ;
#175610=CARTESIAN_POINT ( 'NONE',  ( 11.86145016429273191, 12.69999999999999929, 1.099999999999996980 ) ) ;
#175615=VERTEX_POINT ( 'NONE', #92052 ) ;
#175620=CARTESIAN_POINT ( 'NONE',  ( 11.41381675112453742, 19.00000000000000000, 3.704697986577180746 ) ) ;
#175645=ORIENTED_EDGE ( 'NONE', *, *, #81658, .F. ) ;
#175653=EDGE_LOOP ( 'NONE', ( #81862, #165777, #211468, #149875 ) ) ;
#175655=EDGE_LOOP ( 'NONE', ( #142314, #200459, #75137, #211594, #112837 ) ) ;
#175701=CARTESIAN_POINT ( 'NONE',  ( 7.217521757037772545, 15.46950125388860364, 9.593379878448720532 ) ) ;
#175704=( NAMED_UNIT ( * ) SI_UNIT ( $, .STERADIAN. ) SOLID_ANGLE_UNIT ( ) );
#175706=CARTESIAN_POINT ( 'NONE',  ( -11.88237951145550042, 12.34319347378714937, -0.9087114598430712231 ) ) ;
#175725=ORIENTED_EDGE ( 'NONE', *, *, #180960, .F. ) ;
#175747=AXIS2_PLACEMENT_3D ( 'NONE', #1116, #67178, #199317 ) ;
#175765=ORIENTED_EDGE ( 'NONE', *, *, #68124, .T. ) ;
#175771=CARTESIAN_POINT ( 'NONE',  ( -4.797597452551693564, 14.53090166595112365, -11.00826955084990111 ) ) ;
#175772=DIRECTION ( 'NONE',  ( 0.000000000000000000, 0.000000000000000000, -1.000000000000000000 ) ) ;
#175810=DIRECTION ( 'NONE',  ( 0.9486832980505138790, -0.3162277660168376636, -3.312310031615527152E-15 ) ) ;
#175819=CARTESIAN_POINT ( 'NONE',  ( -11.96533679318059917, 12.34753988812995296, 0.9151144679398905968 ) ) ;
#175831=DIRECTION ( 'NONE',  ( 0.000000000000000000, 0.000000000000000000, -1.000000000000000000 ) ) ;
#175848=( NAMED_UNIT ( * ) PLANE_ANGLE_UNIT ( ) SI_UNIT ( $, .RADIAN. ) );
#175851=ADVANCED_FACE ( 'NONE', ( #160224 ), #193778, .F. ) ;
#175858=EDGE_CURVE ( 'NONE', #140091, #8935, #211084, .T. ) ;
#175860=CARTESIAN_POINT ( 'NONE',  ( 11.62299063338605087, 6.986215174415851159, 1.907829974770760328 ) ) ;
#175868=ORIENTED_EDGE ( 'NONE', *, *, #12933, .F. ) ;
#175878=CARTESIAN_POINT ( 'NONE',  ( 1.459778984583645340E-15, 0.08000000000000020983, -11.92000000000000171 ) ) ;
#175882=AXIS2_PLACEMENT_3D ( 'NONE', #137280, #9392, #154588 ) ;
#175915=LINE ( 'NONE', #124035, #2216 ) ;
#175925=CARTESIAN_POINT ( 'NONE',  ( -11.48243876534946217, 11.37999999999998302, 3.199999999999997957 ) ) ;
#175932=VERTEX_POINT ( 'NONE', #125673 ) ;
#175935=STYLED_ITEM ( 'NONE', ( #98085 ), #154563 ) ;
#175955=CARTESIAN_POINT ( 'NONE',  ( 0.000000000000000000, 3.999999999999994671, 12.00000000000000355 ) ) ;
#175963=CARTESIAN_POINT ( 'NONE',  ( 9.224544533040779370, 13.18315223404453107, 9.019998505197957428 ) ) ;
#175998=CARTESIAN_POINT ( 'NONE',  ( -11.50715376448619764, 7.744667295756731740, 4.958460396591308772 ) ) ;
#175999=EDGE_CURVE ( 'NONE', #24518, #8935, #64844, .T. ) ;
#176010=( LENGTH_UNIT ( ) NAMED_UNIT ( * ) SI_UNIT ( .MILLI., .METRE. ) );
#176022=VERTEX_POINT ( 'NONE', #150281 ) ;
#176023=CARTESIAN_POINT ( 'NONE',  ( 11.62784165634802136, 8.211123330874524839, -2.995123467788005200 ) ) ;
#176070=CARTESIAN_POINT ( 'NONE',  ( -11.31484017231561445, 6.389126039234806598, 4.001117297664503525 ) ) ;
#176074=CARTESIAN_POINT ( 'NONE',  ( 0.008622031262369225790, 14.55347103577515000, 11.95585889282743253 ) ) ;
#176093=ORIENTED_EDGE ( 'NONE', *, *, #12933, .T. ) ;
#176099=( LENGTH_UNIT ( ) NAMED_UNIT ( * ) SI_UNIT ( .MILLI., .METRE. ) );
#176110=CARTESIAN_POINT ( 'NONE',  ( -10.61989522411177944, 7.619981102720494448, -4.513857952992439415 ) ) ;
#176115=ADVANCED_FACE ( 'NONE', ( #188090 ), #50649, .T. ) ;
#176118=ORIENTED_EDGE ( 'NONE', *, *, #213502, .F. ) ;
#176167=LINE ( 'NONE', #99971, #57218 ) ;
#176183=CARTESIAN_POINT ( 'NONE',  ( -10.41986968326957808, 5.020773655391575829, -5.279272669861445166 ) ) ;
#176202=FACE_BOUND ( 'NONE', #88343, .T. ) ;
#176237=ORIENTED_EDGE ( 'NONE', *, *, #184968, .F. ) ;
#176247=CARTESIAN_POINT ( 'NONE',  ( 12.00011339110129605, 6.571252426151665382, -0.4971413739769103834 ) ) ;
#176279=FACE_OUTER_BOUND ( 'NONE', #112059, .T. ) ;
#176286=CARTESIAN_POINT ( 'NONE',  ( -9.453965130556928997, 14.52925576243678130, -7.390745083414802075 ) ) ;
#176289=ORIENTED_EDGE ( 'NONE', *, *, #123836, .T. ) ;
#176307=CARTESIAN_POINT ( 'NONE',  ( -11.78331023100045627, 11.29999999999998117, 1.799999999999999600 ) ) ;
#176318=CARTESIAN_POINT ( 'NONE',  ( 8.266499440872674853, 15.18128111188595675, -8.700183093162271675 ) ) ;
#176346=EDGE_CURVE ( 'NONE', #127758, #187716, #126121, .T. ) ;
#176363=CARTESIAN_POINT ( 'NONE',  ( 11.91826848676304706, 13.50833707238735570, 1.400000051402189971 ) ) ;
#176365=EDGE_LOOP ( 'NONE', ( #58128, #153265, #161627 ) ) ;
#176368=CARTESIAN_POINT ( 'NONE',  ( 9.781847885788174324, 12.99548848723393490, -8.037988007782987054 ) ) ;
#176372=( BOUNDED_SURFACE ( )  B_SPLINE_SURFACE ( 3, 3, ( 
 ( #115551, #3832, #100305, #99256, #199921, #52620, #168502, #153321 ),
 ( #132843, #119821, #101366, #118748, #165304, #16899, #82980, #17963 ),
 ( #184731, #84050, #36357, #150138, #19038, #149053, #198847, #50494 ),
 ( #182609, #67764, #1710, #51568, #20101, #117693, #183685, #86189 ),
 ( #69906, #202029, #85116, #152258, #2773, #200972, #136016, #53689 ),
 ( #137084, #91282, #157341, #173608, #26241, #8929, #75010, #141119 ),
 ( #207130, #28387, #58756, #12126, #11051, #94483, #176772, #124908 ) ),
 .UNSPECIFIED., .T., .F., .T. ) 
 B_SPLINE_SURFACE_WITH_KNOTS ( ( 4, 3, 4 ),
 ( 4, 2, 2, 4 ),
 ( 0.000000000000000000, 0.5000000000000000000, 1.000000000000000000 ),
 ( 0.000000000000000000, 0.08643212109064271620, 0.5432160605453213442, 1.000000000000000000 ),
 .UNSPECIFIED. ) 
 GEOMETRIC_REPRESENTATION_ITEM ( )  RATIONAL_B_SPLINE_SURFACE ( (
 ( 1.000000000000000000, 1.000000000000000000, 1.000000000000000000, 1.000000000000000000, 1.000000000000000000, 1.000000000000000000, 1.000000000000000000, 1.000000000000000000),
 ( 0.3333333333333333703, 0.3333333333333333703, 0.3333333333333333703, 0.3333333333333333703, 0.3333333333333333703, 0.3333333333333333703, 0.3333333333333333703, 0.3333333333333333703),
 ( 0.3333333333333333703, 0.3333333333333333703, 0.3333333333333333703, 0.3333333333333333703, 0.3333333333333333703, 0.3333333333333333703, 0.3333333333333333703, 0.3333333333333333703),
 ( 1.000000000000000000, 1.000000000000000000, 1.000000000000000000, 1.000000000000000000, 1.000000000000000000, 1.000000000000000000, 1.000000000000000000, 1.000000000000000000),
 ( 0.3333333333333333703, 0.3333333333333333703, 0.3333333333333333703, 0.3333333333333333703, 0.3333333333333333703, 0.3333333333333333703, 0.3333333333333333703, 0.3333333333333333703),
 ( 0.3333333333333333703, 0.3333333333333333703, 0.3333333333333333703, 0.3333333333333333703, 0.3333333333333333703, 0.3333333333333333703, 0.3333333333333333703, 0.3333333333333333703),
 ( 1.000000000000000000, 1.000000000000000000, 1.000000000000000000, 1.000000000000000000, 1.000000000000000000, 1.000000000000000000, 1.000000000000000000, 1.000000000000000000) ) ) 
 REPRESENTATION_ITEM ( '' )  SURFACE ( )  );
#176376=CARTESIAN_POINT ( 'NONE',  ( -11.80235830595198010, 11.29999999999999893, -1.696088231482795416 ) ) ;
#176386=EDGE_CURVE ( 'NONE', #181928, #140668, #163891, .T. ) ;
#176395=CARTESIAN_POINT ( 'NONE',  ( 9.601931918643629160, 4.115787718308530962, -7.121346131705980298 ) ) ;
#176423=CARTESIAN_POINT ( 'NONE',  ( -11.81900460097218186, 11.25757134874137755, -1.592493057836596337 ) ) ;
#176430=CARTESIAN_POINT ( 'NONE',  ( 9.475938008234967569, 4.398642192756169855, 7.290290965542337354 ) ) ;
#176468=CIRCLE ( 'NONE', #138453, 12.00000000000000355 ) ;
#176473=ORIENTED_EDGE ( 'NONE', *, *, #130972, .F. ) ;
#176475=SURFACE_SIDE_STYLE ('',( #128866 ) ) ;
#176483=EDGE_CURVE ( 'NONE', #179460, #63230, #63217, .T. ) ;
#176490=ORIENTED_EDGE ( 'NONE', *, *, #97999, .F. ) ;
#176501=PRESENTATION_STYLE_ASSIGNMENT (( #78987 ) ) ;
#176506=DIRECTION ( 'NONE',  ( 0.000000000000000000, 0.000000000000000000, -1.000000000000000000 ) ) ;
#176512=CARTESIAN_POINT ( 'NONE',  ( -10.44369227015510404, 5.112964020592959180, 5.232143560358712087 ) ) ;
#176576=CIRCLE ( 'NONE', #138545, 0.08000000000000014044 ) ;
#176593=VECTOR ( 'NONE', #69038, 1000.000000000000000 ) ;
#176607=CARTESIAN_POINT ( 'NONE',  ( 11.86145016429273191, 19.00000000000000000, 1.179999999999997051 ) ) ;
#176609=DIRECTION ( 'NONE',  ( -0.000000000000000000, 1.000000000000000000, 0.000000000000000000 ) ) ;
#176633=EDGE_LOOP ( 'NONE', ( #41395, #81396, #43622, #203809 ) ) ;
#176649=CARTESIAN_POINT ( 'NONE',  ( -9.569358774130435563, 3.553060279300347180, -7.167287524826059020 ) ) ;
#176656=DIRECTION ( 'NONE',  ( 0.000000000000000000, 0.000000000000000000, -1.000000000000000000 ) ) ;
#176671=CARTESIAN_POINT ( 'NONE',  ( -11.41381675112453209, 13.40000000000000036, -3.704697986577182078 ) ) ;
#176713=CARTESIAN_POINT ( 'NONE',  ( -11.97929049433705373, 12.22000000000000064, 0.7046979865771783036 ) ) ;
#176725=FACE_OUTER_BOUND ( 'NONE', #194350, .T. ) ;
#176772=CARTESIAN_POINT ( 'NONE',  ( -8.752560982292409975, 14.99999996918461775, -9.356054898121708874 ) ) ;
#176825=B_SPLINE_CURVE_WITH_KNOTS ( 'NONE', 3,
 ( #35745, #53063, #36806, #167887, #19488, #151652 ),
 .UNSPECIFIED., .F., .F.,
 ( 4, 2, 4 ),
 ( 0.000000000000000000, 0.0003132070624402877746, 0.0006264141248805755492 ),
 .UNSPECIFIED. ) ;
#176826=CARTESIAN_POINT ( 'NONE',  ( 11.41381676900473430, 11.03041960022390988, -3.704697931490291918 ) ) ;
#176843=CARTESIAN_POINT ( 'NONE',  ( 10.50000000000000178, 13.40000000000000036, -3.600000000000002309 ) ) ;
#176856=ORIENTED_EDGE ( 'NONE', *, *, #206271, .F. ) ;
#176885=CARTESIAN_POINT ( 'NONE',  ( 11.94105721237523277, 10.07259609010266388, -1.187919463087249827 ) ) ;
#176897=STYLED_ITEM ( 'NONE', ( #112775 ), #165716 ) ;
#176913=CARTESIAN_POINT ( 'NONE',  ( 11.31666751210511102, 7.462798040830318946, -3.198044674750592620 ) ) ;
#176917=VERTEX_POINT ( 'NONE', #149762 ) ;
#176938=AXIS2_PLACEMENT_3D ( 'NONE', #128244, #11176, #144445 ) ;
#176939=CARTESIAN_POINT ( 'NONE',  ( -10.50060100873255031, 5.377693802073529206, 5.808388628131297970 ) ) ;
#176969=CARTESIAN_POINT ( 'NONE',  ( -11.43204722947019825, 9.944072459738260150, -3.649275849833183649 ) ) ;
#176972=CARTESIAN_POINT ( 'NONE',  ( 1.000000047849762153, 14.00000000000000533, 11.64874984998672325 ) ) ;
#176977=CARTESIAN_POINT ( 'NONE',  ( -1.416786528094066355, 7.999640415717691688, 11.00953083556809275 ) ) ;
#177012=CARTESIAN_POINT ( 'NONE',  ( -12.00071372354016752, 8.501427447926152681, -1.132741196307404330 ) ) ;
#177016=CARTESIAN_POINT ( 'NONE',  ( 6.743451144134843922, 15.00000000000000000, -9.536680065235831449 ) ) ;
#177019=CARTESIAN_POINT ( 'NONE',  ( 7.457859969268502809, 13.90606279126528300, 8.983713841573639058 ) ) ;
#177038=CARTESIAN_POINT ( 'NONE',  ( -10.49167095263961613, 5.343775707538777731, -5.730694126968513658 ) ) ;
#177042=CARTESIAN_POINT ( 'NONE',  ( -10.39320420135713263, 4.932286138528427344, 5.331284845095887626 ) ) ;
#177043=( NAMED_UNIT ( * ) SI_UNIT ( $, .STERADIAN. ) SOLID_ANGLE_UNIT ( ) );
#177053=CARTESIAN_POINT ( 'NONE',  ( -12.40359606095370992, 6.583381993447835256, -3.463844519762692364 ) ) ;
#177060=ADVANCED_FACE ( 'NONE', ( #2399 ), #111692, .T. ) ;
#177070=CARTESIAN_POINT ( 'NONE',  ( -9.508835372460842095, 14.89852095282139643, 7.212874380408685226 ) ) ;
#177077=CARTESIAN_POINT ( 'NONE',  ( 11.94521494846196319, 7.576335522585334381, -0.4351009623805371374 ) ) ;
#177088=VECTOR ( 'NONE', #4340, 1000.000000000000000 ) ;
#177122=CYLINDRICAL_SURFACE ( 'NONE', #212368, 0.3999999999999997446 ) ;
#177126=CARTESIAN_POINT ( 'NONE',  ( -11.33112879397343065, 6.585244639288670321, 3.816637121560833013 ) ) ;
#177130=CARTESIAN_POINT ( 'NONE',  ( -15.75000000000000000, 11.29999999999998117, 1.799999999999999600 ) ) ;
#177135=CARTESIAN_POINT ( 'NONE',  ( -11.71930699919508356, 8.545276028816752856, 2.376758398160924379 ) ) ;
#177137=( NAMED_UNIT ( * ) SI_UNIT ( $, .STERADIAN. ) SOLID_ANGLE_UNIT ( ) );
#177155=CARTESIAN_POINT ( 'NONE',  ( -11.94105721237523099, 12.69999999999999929, -1.187919463087249827 ) ) ;
#177166=CARTESIAN_POINT ( 'NONE',  ( -11.33520460194134394, 5.279085700950885141, -5.677819296561938955 ) ) ;
#177171=( NAMED_UNIT ( * ) PLANE_ANGLE_UNIT ( ) SI_UNIT ( $, .RADIAN. ) );
#177177=B_SPLINE_CURVE_WITH_KNOTS ( 'NONE', 3,
 ( #107739, #203004, #169459, #56781, #204057, #121863, #53578, #104475, #173763, #88217, #87143, #106651, #3725, #120792, #119712, #6932, #205138, #186769, #55710, #187834, #38396, #122948, #170522, #103399, #22104, #138044, #188906, #40547, #63184, #176939 ),
 .UNSPECIFIED., .F., .F.,
 ( 4, 2, 2, 2, 2, 2, 2, 2, 2, 2, 2, 2, 2, 2, 4 ),
 ( 0.000000000000000000, 0.001872196198237568955, 0.002808294297356353324, 0.003744392396475137910, 0.004680490495593922495, 0.005616588594712706647, 0.007488784792950275819, 0.008424882892069060839, 0.009360980991187844991, 0.01029707909030662914, 0.01123317718942541329, 0.01216927528854419745, 0.01310537338766298333, 0.01404147148678176749, 0.01497756958590055164 ),
 .UNSPECIFIED. ) ;
#177185=CIRCLE ( 'NONE', #166823, 0.08000000000000020983 ) ;
#177198=CARTESIAN_POINT ( 'NONE',  ( -4.373855720720293050, 15.44734568083558912, 11.13580561285369264 ) ) ;
#177210=CARTESIAN_POINT ( 'NONE',  ( 9.681420877353911436, 3.865149423709368648, 7.090140323037526393 ) ) ;
#177227=LINE ( 'NONE', #163115, #144088 ) ;
#177235=CARTESIAN_POINT ( 'NONE',  ( 1.734723475976807094E-15, 14.55305236562695193, 11.95586206896570580 ) ) ;
#177236=DIRECTION ( 'NONE',  ( -0.000000000000000000, 1.000000000000000000, 0.000000000000000000 ) ) ;
#177240=CARTESIAN_POINT ( 'NONE',  ( -9.645406396194509568, 4.042443384815813445, -6.587269312116742270 ) ) ;
#177250=FACE_OUTER_BOUND ( 'NONE', #88466, .T. ) ;
#177257=ORIENTED_EDGE ( 'NONE', *, *, #73951, .T. ) ;
#177308=CARTESIAN_POINT ( 'NONE',  ( 11.01135777277262306, 10.19999999999999929, -1.400000000000001910 ) ) ;
#177319=EDGE_CURVE ( 'NONE', #46947, #43590, #155074, .T. ) ;
#177320=VERTEX_POINT ( 'NONE', #104214 ) ;
#177338=CARTESIAN_POINT ( 'NONE',  ( -1.734723475976807094E-15, 3.553060279300227275, -11.95586206894163617 ) ) ;
#177339=CARTESIAN_POINT ( 'NONE',  ( 11.89197816957260301, 11.29999999999999893, 0.8055420615339542456 ) ) ;
#177340=CARTESIAN_POINT ( 'NONE',  ( 9.444970172009428566, 11.06549187246454125, 7.331777211066839328 ) ) ;
#177344=( LENGTH_UNIT ( ) NAMED_UNIT ( * ) SI_UNIT ( .MILLI., .METRE. ) );
#177348=CARTESIAN_POINT ( 'NONE',  ( -8.789227347474932728, 15.51892067737951741, 8.182113819008643318 ) ) ;
#177369=CARTESIAN_POINT ( 'NONE',  ( 11.33772463945043718, 10.19999999999997264, 3.600000000000075140 ) ) ;
#177380=CARTESIAN_POINT ( 'NONE',  ( 7.191817663470090771, 15.44694763254654113, -9.557497708673340142 ) ) ;
#177430=CARTESIAN_POINT ( 'NONE',  ( 10.91047834641517689, 10.31727674668477768, -5.055935782571435055 ) ) ;
#177437=CARTESIAN_POINT ( 'NONE',  ( -11.91292854676703605, 11.11481529673016233, -1.446370920797322990 ) ) ;
#177462=CARTESIAN_POINT ( 'NONE',  ( -9.587917471435847716, 4.026361754648488223, -6.670783315233271615 ) ) ;
#177465=CIRCLE ( 'NONE', #180863, 11.09999999999999964 ) ;
#177496=CARTESIAN_POINT ( 'NONE',  ( 9.423306279978271860, 13.09470160913627090, -7.356095995331378923 ) ) ;
#177501=( LENGTH_UNIT ( ) NAMED_UNIT ( * ) SI_UNIT ( .MILLI., .METRE. ) );
#177504=CARTESIAN_POINT ( 'NONE',  ( -10.77520153956138138, 4.485527145162882867, 5.284729349356103612 ) ) ;
#177537=CIRCLE ( 'NONE', #46138, 11.09999999999999964 ) ;
#177550=CARTESIAN_POINT ( 'NONE',  ( 11.01135777277262306, 10.90000000000000036, -1.400000000000001910 ) ) ;
#177572=CARTESIAN_POINT ( 'NONE',  ( -9.404204976007665806, 14.49017091736342167, 7.453969464079248652 ) ) ;
#177585=ORIENTED_EDGE ( 'NONE', *, *, #90081, .F. ) ;
#177591=B_SPLINE_CURVE_WITH_KNOTS ( 'NONE', 3,
 ( #32004, #147892, #213908, #197679, #194493, #111184 ),
 .UNSPECIFIED., .F., .F.,
 ( 4, 2, 4 ),
 ( 0.000000000000000000, 0.0003141553954499744596, 0.0006283107908999489193 ),
 .UNSPECIFIED. ) ;
#177601=CARTESIAN_POINT ( 'NONE',  ( -10.50000000000000000, 12.69999999999998153, 3.599999999999999201 ) ) ;
#177613=ORIENTED_EDGE ( 'NONE', *, *, #107860, .T. ) ;
#177665=ORIENTED_EDGE ( 'NONE', *, *, #156430, .F. ) ;
#177680=CARTESIAN_POINT ( 'NONE',  ( -11.48788097203293823, 11.33043054397690241, -3.469500700354831491 ) ) ;
#177686=CARTESIAN_POINT ( 'NONE',  ( -11.06298660227979802, 11.25680399625266936, -0.9087478855431304625 ) ) ;
#177699=SURFACE_STYLE_FILL_AREA ( #210168 ) ;
#177701=CARTESIAN_POINT ( 'NONE',  ( -9.361980464089073806, 14.57101365722899899, 7.422930886903910341 ) ) ;
#177705=TOROIDAL_SURFACE ( 'NONE', #205347, 11.92000000000000171, 0.08000000000000000167 ) ;
#177729=CARTESIAN_POINT ( 'NONE',  ( -11.94651559118242901, 9.948693441210181732, -1.135242698369575587 ) ) ;
#177767=CARTESIAN_POINT ( 'NONE',  ( 8.633889707083076459, 13.74036372393864447, 8.268811287266492727 ) ) ;
#177789=DIRECTION ( 'NONE',  ( 0.8003905289055504024, -4.396526966619893387E-05, 0.5994789398347104559 ) ) ;
#177796=CARTESIAN_POINT ( 'NONE',  ( 11.84104725192624130, 11.10983537451419778, -1.443823348526961814 ) ) ;
#177799=CARTESIAN_POINT ( 'NONE',  ( -11.45846087878745756, 12.50688399218583235, 3.566076377698269351 ) ) ;
#177822=VERTEX_POINT ( 'NONE', #145300 ) ;
#177832=UNCERTAINTY_MEASURE_WITH_UNIT (LENGTH_MEASURE( 1.000000000000000082E-05 ), #82587, 'distance_accuracy_value', 'NONE');
#177833=VERTEX_POINT ( 'NONE', #110692 ) ;
#177843=LINE ( 'NONE', #210314, #164169 ) ;
#177857=DIRECTION ( 'NONE',  ( 0.000000000000000000, 0.000000000000000000, -1.000000000000000000 ) ) ;
#177897=LINE ( 'NONE', #98777, #31680 ) ;
#177905=FACE_OUTER_BOUND ( 'NONE', #82270, .T. ) ;
#177912=CARTESIAN_POINT ( 'NONE',  ( -11.07790593930098311, 11.29999999999999893, 0.6999999999999992895 ) ) ;
#177964=COLOUR_RGB ( '', 0.40784314, 0.44705882, 0.49803922) ;
#177990=CARTESIAN_POINT ( 'NONE',  ( 12.64922964589999843, 7.339083607935379838, 3.660861416055261497 ) ) ;
#178042=CARTESIAN_POINT ( 'NONE',  ( -10.94892088761405802, 5.391493950907642940, -4.806431146316898051 ) ) ;
#178045=CARTESIAN_POINT ( 'NONE',  ( -3.796053574492273874, 15.00000000000182077, 12.24940615670316468 ) ) ;
#178059=ORIENTED_EDGE ( 'NONE', *, *, #195779, .T. ) ;
#178067=CIRCLE ( 'NONE', #63792, 11.05000000000000426 ) ;
#178072=FACE_OUTER_BOUND ( 'NONE', #18760, .T. ) ;
#178085=CARTESIAN_POINT ( 'NONE',  ( -10.62722285141355094, 4.751451743136023254, 5.577054254164887759 ) ) ;
#178089=CARTESIAN_POINT ( 'NONE',  ( 9.599742726594369557, 13.73983281947659840, -8.263962686181493211 ) ) ;
#178092=CARTESIAN_POINT ( 'NONE',  ( 6.939993127879787060, 13.99500908125960663, 9.397576848110693604 ) ) ;
#178102=CARTESIAN_POINT ( 'NONE',  ( -11.44791656467458552, 11.29999999999999716, -3.303228920649581291 ) ) ;
#178125=CARTESIAN_POINT ( 'NONE',  ( -10.45911050446410506, 5.175404930453152197, 5.201426885097844455 ) ) ;
#178131=STYLED_ITEM ( 'NONE', ( #108369 ), #86095 ) ;
#178151=CARTESIAN_POINT ( 'NONE',  ( 11.87811798030312005, 7.788899244876387407, 1.760824057802017784 ) ) ;
#178163=DIRECTION ( 'NONE',  ( -0.000000000000000000, -1.000000000000000000, -0.000000000000000000 ) ) ;
#178173=EDGE_CURVE ( 'NONE', #124966, #213513, #205458, .T. ) ;
#178201=CARTESIAN_POINT ( 'NONE',  ( -11.94105721237523099, 10.19999999999999929, -1.187919463087249827 ) ) ;
#178202=CARTESIAN_POINT ( 'NONE',  ( -11.56409840263781597, 7.060128173693748010, 3.212945948728421541 ) ) ;
#178211=CARTESIAN_POINT ( 'NONE',  ( -11.41530515461175455, 7.844461421556668590, -3.709416182095576442 ) ) ;
#178224=ORIENTED_EDGE ( 'NONE', *, *, #141380, .F. ) ;
#178231=CARTESIAN_POINT ( 'NONE',  ( -11.97929049433705373, 12.22000000000000064, -0.7046979865771834106 ) ) ;
#178235=CARTESIAN_POINT ( 'NONE',  ( 11.86145016429273191, 10.90000000000000036, 1.099999999999996758 ) ) ;
#178243=CARTESIAN_POINT ( 'NONE',  ( -11.76695491367977375, 4.673720869072629291, 4.995412848167406494 ) ) ;
#178251=ORIENTED_EDGE ( 'NONE', *, *, #110028, .F. ) ;
#178267=CARTESIAN_POINT ( 'NONE',  ( 11.45842088241064793, 13.59306470877039885, -3.566211699757709574 ) ) ;
#178280=STYLED_ITEM ( 'NONE', ( #68956 ), #87889 ) ;
#178286=CARTESIAN_POINT ( 'NONE',  ( 9.651614352920402595, 4.121347559867366783, 7.130841425383052545 ) ) ;
#178287=EDGE_CURVE ( 'NONE', #14390, #121817, #28747, .T. ) ;
#178318=CARTESIAN_POINT ( 'NONE',  ( -1.734723475976807094E-15, 4.000007913748543587, -12.17999999982603399 ) ) ;
#178338=FACE_BOUND ( 'NONE', #133939, .T. ) ;
#178392=VERTEX_POINT ( 'NONE', #140513 ) ;
#178404=CARTESIAN_POINT ( 'NONE',  ( -9.333041836230016486, 15.44694763438214125, 7.472413793098208856 ) ) ;
#178406=ORIENTED_EDGE ( 'NONE', *, *, #133034, .F. ) ;
#178415=CARTESIAN_POINT ( 'NONE',  ( 6.882015208740356549, 14.48154074412736847, -9.732639244658484401 ) ) ;
#178451=CARTESIAN_POINT ( 'NONE',  ( 0.008622031262369225790, 14.55347103577515000, 11.95585889282743253 ) ) ;
#178474=CARTESIAN_POINT ( 'NONE',  ( -9.587917471435847716, 4.026361754648488223, -6.670783315233271615 ) ) ;
#178498=CARTESIAN_POINT ( 'NONE',  ( 9.728550251279687089, 13.21449840343153426, 8.106492410889076794 ) ) ;
#178525=SURFACE_STYLE_FILL_AREA ( #49576 ) ;
#178550=CARTESIAN_POINT ( 'NONE',  ( 0.000000000000000000, 4.518467169708412001, 0.000000000000000000 ) ) ;
#178555=STYLED_ITEM ( 'NONE', ( #130086 ), #98770 ) ;
#178560=B_SPLINE_CURVE_WITH_KNOTS ( 'NONE', 3,
 ( #163917, #131453, #115215, #181205, #148721, #50151 ),
 .UNSPECIFIED., .F., .F.,
 ( 4, 2, 4 ),
 ( 0.000000000000000000, 0.0003239988925529259747, 0.0006479977851058519494 ),
 .UNSPECIFIED. ) ;
#178616=DIRECTION ( 'NONE',  ( 0.000000000000000000, 0.000000000000000000, 1.000000000000000000 ) ) ;
#178631=ORIENTED_EDGE ( 'NONE', *, *, #202497, .T. ) ;
#178650=CARTESIAN_POINT ( 'NONE',  ( 0.0001326617329764151682, 14.56986279537652784, 11.92506549394788173 ) ) ;
#178654=CARTESIAN_POINT ( 'NONE',  ( -10.43230948805442893, 5.066484524551064794, 5.254757398418679060 ) ) ;
#178655=ORIENTED_EDGE ( 'NONE', *, *, #11908, .F. ) ;
#178679=CARTESIAN_POINT ( 'NONE',  ( -11.88235317400313917, 11.25664239773029607, -0.9089793033029951452 ) ) ;
#178730=ORIENTED_EDGE ( 'NONE', *, *, #59542, .F. ) ;
#178736=CARTESIAN_POINT ( 'NONE',  ( 11.92050416151433012, 11.15205375279633238, 1.381922468431395767 ) ) ;
#178754=EDGE_CURVE ( 'NONE', #87946, #86738, #191096, .T. ) ;
#178768=ORIENTED_EDGE ( 'NONE', *, *, #211218, .F. ) ;
#178771=FACE_OUTER_BOUND ( 'NONE', #91856, .T. ) ;
#178781=ORIENTED_EDGE ( 'NONE', *, *, #130972, .T. ) ;
#178788=ORIENTED_EDGE ( 'NONE', *, *, #117333, .F. ) ;
#178799=CARTESIAN_POINT ( 'NONE',  ( -11.97929049433705551, 9.719999999999998863, -0.7046979865771821894 ) ) ;
#178808=ORIENTED_EDGE ( 'NONE', *, *, #210828, .T. ) ;
#178809=EDGE_LOOP ( 'NONE', ( #50042, #124417, #62603, #42090 ) ) ;
#178813=EDGE_LOOP ( 'NONE', ( #181798, #77273, #41572, #149797 ) ) ;
#178825=ORIENTED_EDGE ( 'NONE', *, *, #64968, .T. ) ;
#178851=CARTESIAN_POINT ( 'NONE',  ( -10.52211599421018740, 5.354012650763445791, -5.769493145238627108 ) ) ;
#178870=FACE_OUTER_BOUND ( 'NONE', #116913, .T. ) ;
#178891=B_SPLINE_CURVE_WITH_KNOTS ( 'NONE', 3,
 ( #207119, #72843, #204969, #175706, #122779, #93403 ),
 .UNSPECIFIED., .F., .F.,
 ( 4, 2, 4 ),
 ( 0.000000000000000000, 0.0003157158648874024685, 0.0006314317297748052622 ),
 .UNSPECIFIED. ) ;
#178895=ORIENTED_EDGE ( 'NONE', *, *, #154810, .F. ) ;
#178914=FACE_OUTER_BOUND ( 'NONE', #59404, .T. ) ;
#178949=DIRECTION ( 'NONE',  ( 0.000000000000000000, 0.000000000000000000, -1.000000000000000000 ) ) ;
#178966=EDGE_LOOP ( 'NONE', ( #89127, #82427, #8066, #120837 ) ) ;
#178974=CARTESIAN_POINT ( 'NONE',  ( 11.41126283316785361, 11.25874606908454645, -3.405403429622925415 ) ) ;
#179010=FACE_OUTER_BOUND ( 'NONE', #187361, .T. ) ;
#179012=CARTESIAN_POINT ( 'NONE',  ( 6.928203230275514990, 14.48195938056239385, 9.797958971132711525 ) ) ;
#179032=EDGE_LOOP ( 'NONE', ( #13985, #170472, #48255, #24643, #129004, #71075, #71526, #126366 ) ) ;
#179038=CARTESIAN_POINT ( 'NONE',  ( 9.605376611548043897, 12.69998406307712457, 7.195705270794549691 ) ) ;
#179046=FACE_OUTER_BOUND ( 'NONE', #124215, .T. ) ;
#179056=CARTESIAN_POINT ( 'NONE',  ( 12.21012343519211285, 8.048746090400854314, -4.966865933635960850 ) ) ;
#179058=ORIENTED_EDGE ( 'NONE', *, *, #213686, .T. ) ;
#179071=CARTESIAN_POINT ( 'NONE',  ( -11.84668730067608600, 10.89999999999998259, 1.399999999999998579 ) ) ;
#179073=CARTESIAN_POINT ( 'NONE',  ( 11.04536101718726293, 12.59418840193640854, -1.100000000000000311 ) ) ;
#179107=CARTESIAN_POINT ( 'NONE',  ( -11.68273847554845446, 7.482503557960598961, 2.547333347333169407 ) ) ;
#179110=CARTESIAN_POINT ( 'NONE',  ( 0.7124089920922128671, 16.00000000000000000, 12.66466791154580207 ) ) ;
#179121=VECTOR ( 'NONE', #174572, 1000.000000000000000 ) ;
#179139=SURFACE_STYLE_FILL_AREA ( #126194 ) ;
#179151=CARTESIAN_POINT ( 'NONE',  ( 1.469576158976824342E-15, 3.999999999999998224, -12.00000000000000355 ) ) ;
#179155=CARTESIAN_POINT ( 'NONE',  ( 7.618117652040820253, 15.99345985719275909, -10.13859572747731264 ) ) ;
#179158=CARTESIAN_POINT ( 'NONE',  ( 9.216031757539681735, 13.21158034223240918, 9.026211791306899102 ) ) ;
#179190=CARTESIAN_POINT ( 'NONE',  ( -11.37834099079384487, 6.126291437673294205, 3.408052918099385931 ) ) ;
#179202=EDGE_CURVE ( 'NONE', #117081, #11196, #122782, .T. ) ;
#179217=CARTESIAN_POINT ( 'NONE',  ( 11.92064487511310666, 7.617312143620704745, -0.8788818785119806298 ) ) ;
#179268=CARTESIAN_POINT ( 'NONE',  ( -11.84668730067608777, 13.50634727754793651, 1.399999999999998579 ) ) ;
#179269=CARTESIAN_POINT ( 'NONE',  ( -11.86644718583810132, 7.726483972532615319, -1.803327366047848157 ) ) ;
#179278=CARTESIAN_POINT ( 'NONE',  ( -11.52521982855896354, 8.148448055807163470, -3.186923921493055811 ) ) ;
#179294=B_SPLINE_CURVE_WITH_KNOTS ( 'NONE', 3,
 ( #212435, #98712, #14225, #96, #164771, #130220 ),
 .UNSPECIFIED., .F., .F.,
 ( 4, 2, 4 ),
 ( 0.000000000000000000, 0.0003157158648874033901, 0.0006314317297748067801 ),
 .UNSPECIFIED. ) ;
#179297=AXIS2_PLACEMENT_3D ( 'NONE', #106152, #200376, #37901 ) ;
#179298=VECTOR ( 'NONE', #122043, 1000.000000000000000 ) ;
#179310=CARTESIAN_POINT ( 'NONE',  ( -11.80098439192703097, 4.809115636342174760, 4.927210371565812430 ) ) ;
#179330=CARTESIAN_POINT ( 'NONE',  ( -11.84668730067608600, 12.69999999999998153, 1.399999999999998357 ) ) ;
#179339=PRESENTATION_STYLE_ASSIGNMENT (( #180389 ) ) ;
#179365=DIRECTION ( 'NONE',  ( 0.000000000000000000, -1.000000000000000000, 0.000000000000000000 ) ) ;
#179369=CARTESIAN_POINT ( 'NONE',  ( 0.000000000000000000, 12.22000000000000064, 0.000000000000000000 ) ) ;
#179380=CARTESIAN_POINT ( 'NONE',  ( -10.32224513571693869, 3.007486591634276341, -7.366906358548013678 ) ) ;
#179386=AXIS2_PLACEMENT_3D ( 'NONE', #183757, #49497, #16968 ) ;
#179418=SURFACE_SIDE_STYLE ('',( #163166 ) ) ;
#179436=COLOUR_RGB ( '', 0.31764706, 0.68627451, 0.89019608) ;
#179460=VERTEX_POINT ( 'NONE', #28378 ) ;
#179476=CARTESIAN_POINT ( 'NONE',  ( 10.88587197153689701, 8.292399138164135763, 4.942068264615757656 ) ) ;
#179517=CARTESIAN_POINT ( 'NONE',  ( 8.952720908857106252, 14.54244786625251962, -7.923410800768315276 ) ) ;
#179536=ORIENTED_EDGE ( 'NONE', *, *, #23138, .F. ) ;
#179541=CARTESIAN_POINT ( 'NONE',  ( -10.41986968326957808, 5.020773655391575829, -5.279272669861445166 ) ) ;
#179548=CARTESIAN_POINT ( 'NONE',  ( -11.33772463945037146, 12.69999999999998153, 3.599999999999999201 ) ) ;
#179560=EDGE_LOOP ( 'NONE', ( #182197, #192600, #195646, #198965 ) ) ;
#179563=CARTESIAN_POINT ( 'NONE',  ( 11.59565239942670800, 8.772708109194649495, 2.738260425586001912 ) ) ;
#179574=CARTESIAN_POINT ( 'NONE',  ( 8.140346590616603706, 14.24105188827307167, -8.817491472814088738 ) ) ;
#179578=CARTESIAN_POINT ( 'NONE',  ( -11.04984958223792368, 13.60917513768126597, 1.056557932048282078 ) ) ;
#179590=( NAMED_UNIT ( * ) SI_UNIT ( $, .STERADIAN. ) SOLID_ANGLE_UNIT ( ) );
#179593=CARTESIAN_POINT ( 'NONE',  ( 1.250000000000037526, 8.500000000000000000, 10.97907099895068583 ) ) ;
#179596=CARTESIAN_POINT ( 'NONE',  ( -9.508841981786570585, 14.91423885135806415, 7.212865296072065391 ) ) ;
#179605=( NAMED_UNIT ( * ) SI_UNIT ( $, .STERADIAN. ) SOLID_ANGLE_UNIT ( ) );
#179613=AXIS2_PLACEMENT_3D ( 'NONE', #22253, #186909, #204197 ) ;
#179649=DIRECTION ( 'NONE',  ( 0.000000000000000000, 0.000000000000000000, -1.000000000000000000 ) ) ;
#179681=AXIS2_PLACEMENT_3D ( 'NONE', #192742, #10794, #207933 ) ;
#179698=B_SPLINE_CURVE_WITH_KNOTS ( 'NONE', 3,
 ( #81107, #180738, #61662, #113683, #29163, #148257 ),
 .UNSPECIFIED., .F., .F.,
 ( 4, 2, 4 ),
 ( 0.000000000000000000, 0.0003168911866439334617, 0.0006337823732878669234 ),
 .UNSPECIFIED. ) ;
#179708=CARTESIAN_POINT ( 'NONE',  ( 11.84668730067608600, 19.00000000000000000, 1.319999999999998286 ) ) ;
#179732=EDGE_CURVE ( 'NONE', #18531, #37868, #136652, .T. ) ;
#179751=EDGE_CURVE ( 'NONE', #150697, #83956, #177843, .T. ) ;
#179790=ORIENTED_EDGE ( 'NONE', *, *, #164554, .T. ) ;
#179827=( LENGTH_UNIT ( ) NAMED_UNIT ( * ) SI_UNIT ( .MILLI., .METRE. ) );
#179847=CARTESIAN_POINT ( 'NONE',  ( -11.94655611907590220, 13.65200944546904083, 1.134828163062136852 ) ) ;
#179864=CARTESIAN_POINT ( 'NONE',  ( -15.75000000000000000, 10.19999999999998153, 1.399999999999998579 ) ) ;
#179897=DIRECTION ( 'NONE',  ( -0.000000000000000000, -1.000000000000000000, -0.000000000000000000 ) ) ;
#179905=DIRECTION ( 'NONE',  ( 1.000000000000000000, -0.000000000000000000, -0.000000000000000000 ) ) ;
#179909=EDGE_CURVE ( 'NONE', #36225, #76712, #46507, .T. ) ;
#179923=DIRECTION ( 'NONE',  ( 1.000000000000000000, 0.000000000000000000, 0.000000000000000000 ) ) ;
#179926=CARTESIAN_POINT ( 'NONE',  ( -11.55950211276791428, 12.21999999999998288, 3.221476510067112109 ) ) ;
#179937=DIRECTION ( 'NONE',  ( 0.000000000000000000, 0.000000000000000000, -1.000000000000000000 ) ) ;
#179943=CIRCLE ( 'NONE', #20809, 11.92000000000000171 ) ;
#179971=( LENGTH_UNIT ( ) NAMED_UNIT ( * ) SI_UNIT ( .MILLI., .METRE. ) );
#179973=ORIENTED_EDGE ( 'NONE', *, *, #87967, .F. ) ;
#180002=STYLED_ITEM ( 'NONE', ( #139110 ), #162075 ) ;
#180011=ADVANCED_FACE ( 'NONE', ( #211291 ), #62916, .T. ) ;
#180029=DIRECTION ( 'NONE',  ( 0.000000000000000000, 1.000000000000000000, 0.000000000000000000 ) ) ;
#180046=FACE_OUTER_BOUND ( 'NONE', #47351, .T. ) ;
#180070=CARTESIAN_POINT ( 'NONE',  ( 0.03257979115088038835, 14.52968454062227188, 11.98509113246684699 ) ) ;
#180078=CARTESIAN_POINT ( 'NONE',  ( -11.78331023100045627, 9.799999999999998934, -1.800000000000001155 ) ) ;
#180089=ORIENTED_EDGE ( 'NONE', *, *, #201840, .T. ) ;
#180094=DIRECTION ( 'NONE',  ( -0.000000000000000000, -1.000000000000000000, -0.000000000000000000 ) ) ;
#180097=CARTESIAN_POINT ( 'NONE',  ( -11.84668729035104384, 10.09481419982587802, -1.400000000000001688 ) ) ;
#180105=CIRCLE ( 'NONE', #197401, 12.00000000000000178 ) ;
#180116=CARTESIAN_POINT ( 'NONE',  ( 9.259438961641526689, 13.05523824266862398, 8.991576184352215506 ) ) ;
#180125=CARTESIAN_POINT ( 'NONE',  ( 11.00592740523952173, 9.989797575316798017, 1.444008943503716225 ) ) ;
#180132=CARTESIAN_POINT ( 'NONE',  ( -11.88168329227127096, 11.37999999999998302, 1.685799833707126050 ) ) ;
#180141=STYLED_ITEM ( 'NONE', ( #6723 ), #163490 ) ;
#180168=CARTESIAN_POINT ( 'NONE',  ( -11.91807834161487634, 8.018667342336753379, 1.063137970766440121 ) ) ;
#180172=CARTESIAN_POINT ( 'NONE',  ( -11.95753012856830644, 7.932397174992964928, -1.041636101723666163 ) ) ;
#180185=AXIS2_PLACEMENT_3D ( 'NONE', #193826, #162420, #212198 ) ;
#180190=VERTEX_POINT ( 'NONE', #17 ) ;
#180192=STYLED_ITEM ( 'NONE', ( #182945 ), #57047 ) ;
#180218=CARTESIAN_POINT ( 'NONE',  ( 8.771385051288104862, 13.55262984818672045, -7.723180138624951674 ) ) ;
#180227=ORIENTED_EDGE ( 'NONE', *, *, #117565, .T. ) ;
#180250=CARTESIAN_POINT ( 'NONE',  ( -11.01567899581106325, 5.044704703271206903, 4.264317011375222677 ) ) ;
#180265=DIRECTION ( 'NONE',  ( 0.000000000000000000, 1.000000000000000000, 0.000000000000000000 ) ) ;
#180270=CARTESIAN_POINT ( 'NONE',  ( -9.472628840146047224, 14.62787916692008849, 7.367007921869499931 ) ) ;
#180278=CARTESIAN_POINT ( 'NONE',  ( 10.86983561997773684, 9.640297115645962478, 5.096404461738570646 ) ) ;
#180325=CARTESIAN_POINT ( 'NONE',  ( -11.99120512803725447, 8.059048065725468390, -0.5291463972175238784 ) ) ;
#180333=CARTESIAN_POINT ( 'NONE',  ( -11.95117894359873212, 8.932389826126765797, -1.235014725827771720 ) ) ;
#180337=PRESENTATION_STYLE_ASSIGNMENT (( #63387 ) ) ;
#180341=ORIENTED_EDGE ( 'NONE', *, *, #209339, .F. ) ;
#180352=DIRECTION ( 'NONE',  ( 0.000000000000000000, 1.000000000000000000, 0.000000000000000000 ) ) ;
#180389=SURFACE_STYLE_USAGE ( .BOTH. , #97035 ) ;
#180390=CARTESIAN_POINT ( 'NONE',  ( -6.732740262479597781, 15.44786667752632248, 9.889642727345355766 ) ) ;
#180403=CARTESIAN_POINT ( 'NONE',  ( 9.601861708076793178, 3.883749503203103526, 7.121442012218603956 ) ) ;
#180491=B_SPLINE_CURVE_WITH_KNOTS ( 'NONE', 3,
 ( #70864, #69311, #4304, #200385, #34698, #184144, #136492, #135422, #35767, #68248, #198256, #118159 ),
 .UNSPECIFIED., .F., .F.,
 ( 4, 2, 2, 2, 2, 4 ),
 ( 0.000000000000000000, 0.0007653844701297385540, 0.001530768940259477108, 0.001913461175324346819, 0.002296153410389216963, 0.003061537880518958119 ),
 .UNSPECIFIED. ) ;
#180509=DIRECTION ( 'NONE',  ( 0.000000000000000000, 1.000000000000000000, 0.000000000000000000 ) ) ;
#180544=ADVANCED_FACE ( 'NONE', ( #188384 ), #122427, .F. ) ;
#180561=CARTESIAN_POINT ( 'NONE',  ( 11.86145016429273191, 10.19999999999999929, -1.100000000000000533 ) ) ;
#180562=CARTESIAN_POINT ( 'NONE',  ( -15.75000000000000000, 12.69999999999999929, -1.800000000000001155 ) ) ;
#180564=CARTESIAN_POINT ( 'NONE',  ( -11.78331023100045627, 11.37999999999998302, 1.799999999999999600 ) ) ;
#180590=CARTESIAN_POINT ( 'NONE',  ( -9.968662085647130411, 5.546348307810219147, -6.001034872913991514 ) ) ;
#180598=CARTESIAN_POINT ( 'NONE',  ( -11.33772463945037323, 12.59097530385348307, 3.599999999999999201 ) ) ;
#180604=CARTESIAN_POINT ( 'NONE',  ( -15.75000000000000000, 10.19999999999999929, -1.100000000000000311 ) ) ;
#180610=ORIENTED_EDGE ( 'NONE', *, *, #510, .F. ) ;
#180613=CARTESIAN_POINT ( 'NONE',  ( 8.857939311156123097, 13.09004391473939677, -7.626805567664353802 ) ) ;
#180648=CARTESIAN_POINT ( 'NONE',  ( -10.19200560444942560, 4.477620260464512114, -5.707107691925500603 ) ) ;
#180659=SURFACE_SIDE_STYLE ('',( #14934 ) ) ;
#180672=SURFACE_STYLE_FILL_AREA ( #162305 ) ;
#180717=COLOUR_RGB ( '', 0.66274510, 0.83137255, 0.94901961) ;
#180722=CARTESIAN_POINT ( 'NONE',  ( -11.94980361058168938, 10.19999999999999929, 1.099999999999996980 ) ) ;
#180729=ORIENTED_EDGE ( 'NONE', *, *, #151802, .T. ) ;
#180731=CARTESIAN_POINT ( 'NONE',  ( 1.469576158976824144E-15, 3.481540744127368026, 12.00000000000000178 ) ) ;
#180738=CARTESIAN_POINT ( 'NONE',  ( 11.80247861663003484, 12.29999999999998295, 1.695431928471866190 ) ) ;
#180747=VERTEX_POINT ( 'NONE', #152696 ) ;
#180758=CYLINDRICAL_SURFACE ( 'NONE', #43914, 0.07999999999999998779 ) ;
#180786=VECTOR ( 'NONE', #81739, 1000.000000000000000 ) ;
#180793=CARTESIAN_POINT ( 'NONE',  ( -11.89197415570408900, 11.29999999999999893, -0.8055989572471861093 ) ) ;
#180820=CARTESIAN_POINT ( 'NONE',  ( 8.564503538342812305, 13.79480036990495861, 8.405811576776271110 ) ) ;
#180841=EDGE_CURVE ( 'NONE', #37868, #208182, #1620, .T. ) ;
#180863=AXIS2_PLACEMENT_3D ( 'NONE', #34275, #84096, #1752 ) ;
#180880=DIRECTION ( 'NONE',  ( -1.000000000000000000, 0.000000000000000000, 1.224646799147353207E-16 ) ) ;
#180891=CARTESIAN_POINT ( 'NONE',  ( -11.41126283316785361, 11.25874606908456776, 3.405403429622881006 ) ) ;
#180906=CARTESIAN_POINT ( 'NONE',  ( -11.71938954792528698, 8.545439090133012172, 2.376335979313274560 ) ) ;
#180956=CARTESIAN_POINT ( 'NONE',  ( -10.42538027328838801, 5.087954508094563622, -5.944375093558058154 ) ) ;
#180960=EDGE_CURVE ( 'NONE', #79990, #80159, #167557, .T. ) ;
#180965=CARTESIAN_POINT ( 'NONE',  ( 11.41381675112453387, 12.69999999999998153, 3.704697986577180746 ) ) ;
#180977=CARTESIAN_POINT ( 'NONE',  ( -11.44779963594988814, 12.69999999999998153, 3.600000000000001421 ) ) ;
#180989=SURFACE_SIDE_STYLE ('',( #146394 ) ) ;
#180996=COLOUR_RGB ( '', 0.09019608, 0.27058824, 0.51372549) ;
#181022=SURFACE_SIDE_STYLE ('',( #17430 ) ) ;
#181025=CARTESIAN_POINT ( 'NONE',  ( -10.59782195348455680, 9.799999999999997158, -3.302675849420335652 ) ) ;
#181028=UNCERTAINTY_MEASURE_WITH_UNIT (LENGTH_MEASURE( 1.000000000000000082E-05 ), #179827, 'distance_accuracy_value', 'NONE');
#181087=EDGE_CURVE ( 'NONE', #47238, #149901, #61590, .T. ) ;
#181100=ADVANCED_FACE ( 'NONE', ( #45359 ), #60416, .F. ) ;
#181113=EDGE_LOOP ( 'NONE', ( #55487, #109377, #189840, #57892 ) ) ;
#181120=VERTEX_POINT ( 'NONE', #109353 ) ;
#181143=ORIENTED_EDGE ( 'NONE', *, *, #105829, .F. ) ;
#181149=CARTESIAN_POINT ( 'NONE',  ( 0.000000000000000000, 4.000007913748540922, 0.000000000000000000 ) ) ;
#181152=CARTESIAN_POINT ( 'NONE',  ( -11.88172094500852971, 9.720000056015496881, -1.685553348215898861 ) ) ;
#181158=( NAMED_UNIT ( * ) PLANE_ANGLE_UNIT ( ) SI_UNIT ( $, .RADIAN. ) );
#181171=CARTESIAN_POINT ( 'NONE',  ( 9.299556801071242162, 12.92894989638156922, -8.960987479870890837 ) ) ;
#181172=ORIENTED_EDGE ( 'NONE', *, *, #129757, .F. ) ;
#181174=VERTEX_POINT ( 'NONE', #57331 ) ;
#181205=CARTESIAN_POINT ( 'NONE',  ( 11.35610322553117157, 9.985783710708249217, -3.553412924323506861 ) ) ;
#181222=DIRECTION ( 'NONE',  ( 0.000000000000000000, 0.000000000000000000, 1.000000000000000000 ) ) ;
#181252=( NAMED_UNIT ( * ) SI_UNIT ( $, .STERADIAN. ) SOLID_ANGLE_UNIT ( ) );
#181266=CARTESIAN_POINT ( 'NONE',  ( 6.978933388731730858, 14.99484663357710801, -9.366624288252014097 ) ) ;
#181286=CARTESIAN_POINT ( 'NONE',  ( 11.78331023100045627, 13.79999999999999893, -1.800000000000001155 ) ) ;
#181298=CARTESIAN_POINT ( 'NONE',  ( -11.37872555039425748, 6.127336012342636806, -3.407788289652350588 ) ) ;
#181302=CARTESIAN_POINT ( 'NONE',  ( 9.168541482314250146, 14.15586233142781758, -7.671659664418466917 ) ) ;
#181320=CARTESIAN_POINT ( 'NONE',  ( -9.490193176586279478, 14.79883486810179427, 7.238303200480997290 ) ) ;
#181341=CARTESIAN_POINT ( 'NONE',  ( 11.84103413958613160, 12.48995521526856578, -1.443924719788771682 ) ) ;
#181367=AXIS2_PLACEMENT_3D ( 'NONE', #209629, #145767, #130614 ) ;
#181381=CARTESIAN_POINT ( 'NONE',  ( -11.95500993068053930, 8.101295389535254188, -0.2609214463033582843 ) ) ;
#181389=CARTESIAN_POINT ( 'NONE',  ( -11.98824733424307709, 9.000663626117129112, 0.6135287215046117959 ) ) ;
#181405=CYLINDRICAL_SURFACE ( 'NONE', #208092, 0.3999999999999997446 ) ;
#181435=DIRECTION ( 'NONE',  ( 0.000000000000000000, 1.000000000000000000, 0.000000000000000000 ) ) ;
#181442=( LENGTH_UNIT ( ) NAMED_UNIT ( * ) SI_UNIT ( .MILLI., .METRE. ) );
#181453=CARTESIAN_POINT ( 'NONE',  ( 9.622977958535759768, 4.242291508015313184, 7.169920593678671850 ) ) ;
#181488=PLANE ( 'NONE',  #26217 ) ;
#181507=COLOUR_RGB ( '', 0.31764706, 0.68627451, 0.89019608) ;
#181522=UNCERTAINTY_MEASURE_WITH_UNIT (LENGTH_MEASURE( 1.000000000000000082E-05 ), #154558, 'distance_accuracy_value', 'NONE');
#181580=CARTESIAN_POINT ( 'NONE',  ( -15.75000000000000000, 10.90000000000000036, -3.200000000000001510 ) ) ;
#181593=FACE_OUTER_BOUND ( 'NONE', #182516, .T. ) ;
#181635=VERTEX_POINT ( 'NONE', #213736 ) ;
#181642=CARTESIAN_POINT ( 'NONE',  ( -9.645406396194509568, 4.042443384815813445, -6.587269312116742270 ) ) ;
#181658=CARTESIAN_POINT ( 'NONE',  ( 9.285642839235046964, 11.47635228829340370, -7.530412293235562160 ) ) ;
#181667=CARTESIAN_POINT ( 'NONE',  ( 9.263131865311954982, 13.58559029627111592, -6.818719126704674949 ) ) ;
#181679=ORIENTED_EDGE ( 'NONE', *, *, #92241, .F. ) ;
#181691=SURFACE_SIDE_STYLE ('',( #194757 ) ) ;
#181700=ORIENTED_EDGE ( 'NONE', *, *, #135941, .F. ) ;
#181716=CARTESIAN_POINT ( 'NONE',  ( -11.86145016429273191, 13.40000000000000036, 1.099999999999996758 ) ) ;
#181742=VERTEX_POINT ( 'NONE', #55539 ) ;
#181749=SURFACE_STYLE_FILL_AREA ( #198008 ) ;
#181798=ORIENTED_EDGE ( 'NONE', *, *, #175858, .T. ) ;
#181856=EDGE_CURVE ( 'NONE', #167726, #123196, #98160, .T. ) ;
#181871=CARTESIAN_POINT ( 'NONE',  ( 7.323366971182228902, 14.46633393321924999, 9.509224143632334147 ) ) ;
#181891=AXIS2_PLACEMENT_3D ( 'NONE', #42793, #23285, #92612 ) ;
#181928=VERTEX_POINT ( 'NONE', #183400 ) ;
#181930=CARTESIAN_POINT ( 'NONE',  ( 8.396038884180011763, 15.16511954447424593, 8.575115785561168380 ) ) ;
#181932=CARTESIAN_POINT ( 'NONE',  ( -10.30047605039691128, 4.688744718740807116, 5.507884344589919934 ) ) ;
#181934=CARTESIAN_POINT ( 'NONE',  ( -11.89942855770814134, 11.37999999999999901, 0.6999999999999992895 ) ) ;
#181953=CARTESIAN_POINT ( 'NONE',  ( -11.41381675112460670, 11.03016735491473810, 3.704697986577268232 ) ) ;
#181970=ORIENTED_EDGE ( 'NONE', *, *, #70055, .T. ) ;
#182001=ORIENTED_EDGE ( 'NONE', *, *, #48333, .T. ) ;
#182014=CARTESIAN_POINT ( 'NONE',  ( -11.48784849554596121, 12.26950472818065663, -3.469614872287748231 ) ) ;
#182023=DIRECTION ( 'NONE',  ( -0.000000000000000000, -1.000000000000000000, -0.000000000000000000 ) ) ;
#182025=FACE_OUTER_BOUND ( 'NONE', #34178, .T. ) ;
#182038=CARTESIAN_POINT ( 'NONE',  ( -11.84668730067608600, 19.00000000000000000, -1.320000000000001616 ) ) ;
#182044=CARTESIAN_POINT ( 'NONE',  ( 0.000000000000000000, 0.08000000000000020983, 0.000000000000000000 ) ) ;
#182046=AXIS2_PLACEMENT_3D ( 'NONE', #46606, #212266, #44478 ) ;
#182072=CARTESIAN_POINT ( 'NONE',  ( -10.33392256004288079, 4.765625372279607141, 5.445010993851796322 ) ) ;
#182080=ORIENTED_EDGE ( 'NONE', *, *, #114896, .T. ) ;
#182085=EDGE_LOOP ( 'NONE', ( #160384, #122646, #119546, #210443 ) ) ;
#182128=CARTESIAN_POINT ( 'NONE',  ( -10.16842870470028437, 3.679487716134552944, -6.373158935749277276 ) ) ;
#182137=DIRECTION ( 'NONE',  ( -0.000000000000000000, -1.000000000000000000, -0.000000000000000000 ) ) ;
#182148=DIRECTION ( 'NONE',  ( -1.000000000000000000, 0.000000000000000000, 0.000000000000000000 ) ) ;
#182170=EDGE_CURVE ( 'NONE', #26907, #138623, #167720, .T. ) ;
#182180=B_SPLINE_CURVE_WITH_KNOTS ( 'NONE', 3,
 ( #177235, #194535, #45122, #47255, #13647, #162058, #193478 ),
 .UNSPECIFIED., .F., .F.,
 ( 4, 3, 4 ),
 ( -5.999999999944987321E-08, 0.000000000000000000, 8.562056648505256864E-06 ),
 .UNSPECIFIED. ) ;
#182191=CARTESIAN_POINT ( 'NONE',  ( -11.35605497252127094, 12.48581854048354423, -3.553547709190210124 ) ) ;
#182197=ORIENTED_EDGE ( 'NONE', *, *, #2823, .T. ) ;
#182206=CARTESIAN_POINT ( 'NONE',  ( -11.78331023100045627, 9.799999999999998934, -1.800000000000001155 ) ) ;
#182215=( LENGTH_UNIT ( ) NAMED_UNIT ( * ) SI_UNIT ( .MILLI., .METRE. ) );
#182216=CARTESIAN_POINT ( 'NONE',  ( 11.33772463945037323, 13.50902469614648815, 3.599999999999999201 ) ) ;
#182226=CARTESIAN_POINT ( 'NONE',  ( 13.13649811952651270, 6.591446614545316329, 1.105413235251222925 ) ) ;
#182260=CARTESIAN_POINT ( 'NONE',  ( 11.55950211276791251, 12.22000000000000064, -3.221476510067114329 ) ) ;
#182270=AXIS2_PLACEMENT_3D ( 'NONE', #185750, #37383, #150087 ) ;
#182275=CARTESIAN_POINT ( 'NONE',  ( -11.78331023100045627, 13.79999999999998295, 1.799999999999999600 ) ) ;
#182280=DIRECTION ( 'NONE',  ( -0.000000000000000000, -1.000000000000000000, -0.000000000000000000 ) ) ;
#182283=ADVANCED_FACE ( 'NONE', ( #57680 ), #139241, .T. ) ;
#182301=DIRECTION ( 'NONE',  ( -0.000000000000000000, -1.000000000000000000, -0.000000000000000000 ) ) ;
#182304=CARTESIAN_POINT ( 'NONE',  ( -15.75000000000000000, 13.79999999999999893, -1.800000000000001155 ) ) ;
#182323=CARTESIAN_POINT ( 'NONE',  ( 9.148157776457804147, 13.34235666145839616, -9.071852530902138056 ) ) ;
#182341=CARTESIAN_POINT ( 'NONE',  ( 11.81911962874442068, 13.75710573484113475, -1.591749704452471326 ) ) ;
#182344=B_SPLINE_CURVE_WITH_KNOTS ( 'NONE', 3,
 ( #155571, #68942, #2872, #7154, #86291, #185903 ),
 .UNSPECIFIED., .F., .F.,
 ( 4, 2, 4 ),
 ( 0.000000000000000000, 0.0003767011250903910184, 0.0007534022501807818200 ),
 .UNSPECIFIED. ) ;
#182367=VERTEX_POINT ( 'NONE', #123837 ) ;
#182383=CARTESIAN_POINT ( 'NONE',  ( 11.88237951145550220, 11.25680652621284494, -0.9087114598430711121 ) ) ;
#182388=CARTESIAN_POINT ( 'NONE',  ( 7.006712406718516029, 14.55305236961725690, -9.688386885671178561 ) ) ;
#182395=( GEOMETRIC_REPRESENTATION_CONTEXT ( 3 ) GLOBAL_UNCERTAINTY_ASSIGNED_CONTEXT ( ( #61955 ) ) GLOBAL_UNIT_ASSIGNED_CONTEXT ( ( #41497, #205018, #169339 ) ) REPRESENTATION_CONTEXT ( 'NONE', 'WORKASPACE' ) );
#182412=CARTESIAN_POINT ( 'NONE',  ( -15.75000000000000000, 10.19999999999999929, -1.400000000000001910 ) ) ;
#182442=CARTESIAN_POINT ( 'NONE',  ( -11.63070519946230874, 8.357210500689234323, 2.967829092913087941 ) ) ;
#182445=CARTESIAN_POINT ( 'NONE',  ( -15.75000000000000000, 13.79999999999999893, 0.6999999999999992895 ) ) ;
#182455=VERTEX_POINT ( 'NONE', #92 ) ;
#182459=CARTESIAN_POINT ( 'NONE',  ( -11.96217875511318063, 9.771456334210229855, -0.9561995067075080845 ) ) ;
#182472=VERTEX_POINT ( 'NONE', #28370 ) ;
#182473=DIRECTION ( 'NONE',  ( 0.000000000000000000, -1.000000000000000000, 0.000000000000000000 ) ) ;
#182489=CARTESIAN_POINT ( 'NONE',  ( -10.51568781791557328, 12.48743269796084299, 3.554797817682051164 ) ) ;
#182490=FACE_OUTER_BOUND ( 'NONE', #176633, .T. ) ;
#182493=AXIS2_PLACEMENT_3D ( 'NONE', #168435, #54682, #52551 ) ;
#182516=EDGE_LOOP ( 'NONE', ( #114127, #94729, #169692, #43455 ) ) ;
#182525=B_SPLINE_CURVE_WITH_KNOTS ( 'NONE', 3,
 ( #47147, #28742, #45012, #113263, #179268, #43941 ),
 .UNSPECIFIED., .F., .F.,
 ( 4, 2, 4 ),
 ( 0.000000000000000000, 0.0003168911866439334617, 0.0006337823732878669234 ),
 .UNSPECIFIED. ) ;
#182550=DIRECTION ( 'NONE',  ( -1.000000000000000000, 0.000000000000000000, 0.000000000000000000 ) ) ;
#182558=CARTESIAN_POINT ( 'NONE',  ( -11.86239285000045740, 13.87999999999998302, 1.812080536912751283 ) ) ;
#182579=CARTESIAN_POINT ( 'NONE',  ( 11.89942855770814312, 11.29999999999999893, 0.6999999999999992895 ) ) ;
#182580=SHAPE_DEFINITION_REPRESENTATION ( #194171, #135824 ) ;
#182609=CARTESIAN_POINT ( 'NONE',  ( 1.000000047849771923, 15.00000000000000888, -11.64874984998672502 ) ) ;
#182612=CARTESIAN_POINT ( 'NONE',  ( -10.91449010664383223, 5.922815305582411760, 6.336942051301835299 ) ) ;
#182641=UNCERTAINTY_MEASURE_WITH_UNIT (LENGTH_MEASURE( 1.000000000000000082E-05 ), #164668, 'distance_accuracy_value', 'NONE');
#182648=CARTESIAN_POINT ( 'NONE',  ( 10.56513397747884397, 12.34099903485656213, 3.405015282931167508 ) ) ;
#182685=CARTESIAN_POINT ( 'NONE',  ( 11.86686399458719521, 9.990712702246625554, -1.056461745586973588 ) ) ;
#182687=EDGE_CURVE ( 'NONE', #199511, #133821, #53756, .T. ) ;
#182699=( BOUNDED_SURFACE ( )  B_SPLINE_SURFACE ( 3, 2, ( 
 ( #101941, #149628, #135521 ),
 ( #197301, #18543, #133412 ),
 ( #48941, #199419, #32674 ),
 ( #201542, #98753, #117185 ),
 ( #183186, #19613, #34791 ),
 ( #164810, #151773, #3345 ),
 ( #16402, #82480, #69414 ),
 ( #150709, #100866, #166952 ),
 ( #153898, #5467, #27888 ),
 ( #137657, #110277, #87828 ),
 ( #158962, #76631, #71549 ),
 ( #127620, #209818, #203677 ),
 ( #190372, #26814, #152825 ),
 ( #142746, #58258, #176286 ),
 ( #124414, #38011, #170132 ),
 ( #160027, #191437, #141686 ),
 ( #70473, #10557, #193584 ),
 ( #175229, #192505, #93985 ) ),
 .UNSPECIFIED., .F., .F., .F. ) 
 B_SPLINE_SURFACE_WITH_KNOTS ( ( 4, 2, 2, 2, 2, 2, 2, 2, 4 ),
 ( 3, 3 ),
 ( 2.412349833780247366E-18, 8.835779862913541985E-05, 0.0001767155972582684273, 0.0003534311945165344152, 0.0007068623890330664452, 0.001060293583549598529, 0.001237009180807864626, 0.001325366979436997565, 0.001413724778066130505 ),
 ( 0.000000000000000000, 1.000000000000000000 ),
 .UNSPECIFIED. ) 
 GEOMETRIC_REPRESENTATION_ITEM ( )  RATIONAL_B_SPLINE_SURFACE ( (
 ( 1.000000000000000000, 0.8509629433930240294, 1.000000000000000000),
 ( 1.000000000000000000, 0.8498006689708330619, 1.000000000000000000),
 ( 1.000000000000000000, 0.8320552336068607335, 1.000000000000000000),
 ( 1.000000000000000000, 0.8099185496895315861, 1.000000000000000000),
 ( 1.000000000000000000, 0.8026556248574672203, 1.000000000000000000),
 ( 1.000000000000000000, 0.7864057361600924612, 1.000000000000000000),
 ( 1.000000000000000000, 0.7820376697136646182, 1.000000000000000000),
 ( 1.000000000000000000, 0.7712304172528938739, 1.000000000000000000),
 ( 1.000000000000000000, 0.7693781127658743113, 1.000000000000000000),
 ( 1.000000000000000000, 0.7693828318226363372, 1.000000000000000000),
 ( 1.000000000000000000, 0.7713025106372017881, 1.000000000000000000),
 ( 1.000000000000000000, 0.7820120508712598006, 1.000000000000000000),
 ( 1.000000000000000000, 0.7865355378789550267, 1.000000000000000000),
 ( 1.000000000000000000, 0.8025478247494930439, 1.000000000000000000),
 ( 1.000000000000000000, 0.8098425554835826379, 1.000000000000000000),
 ( 1.000000000000000000, 0.8320142507518490937, 1.000000000000000000),
 ( 1.000000000000000000, 0.8496692035686509437, 1.000000000000000000),
 ( 1.000000000000000000, 0.8509629433917188512, 1.000000000000000000) ) ) 
 REPRESENTATION_ITEM ( '' )  SURFACE ( )  );
#182713=CARTESIAN_POINT ( 'NONE',  ( -9.857748099689047194, 5.276144085703439401, -6.217795349555793827 ) ) ;
#182723=CARTESIAN_POINT ( 'NONE',  ( -11.69243366784185945, 8.407932920124673970, 1.097391832464843286 ) ) ;
#182729=CARTESIAN_POINT ( 'NONE',  ( 11.87808349579980671, 6.802413298898714267, -1.723793258986091370 ) ) ;
#182740=COLOUR_RGB ( '', 0.31764706, 0.68627451, 0.89019608) ;
#182742=CARTESIAN_POINT ( 'NONE',  ( 9.309616742661452449, 13.13421366227010445, -6.702222026789643294 ) ) ;
#182794=DIRECTION ( 'NONE',  ( 0.9885327375000381167, 0.000000000000000000, 0.1510067114093955609 ) ) ;
#182807=EDGE_LOOP ( 'NONE', ( #204450, #45557, #144084, #4637 ) ) ;
#182851=CARTESIAN_POINT ( 'NONE',  ( -11.94105722165067363, 10.07417237917041497, 1.187919369849792295 ) ) ;
#182852=TOROIDAL_SURFACE ( 'NONE', #89503, 12.17999951260719804, 0.5000000000000008882 ) ;
#182863=UNCERTAINTY_MEASURE_WITH_UNIT (LENGTH_MEASURE( 1.000000000000000082E-05 ), #183635, 'distance_accuracy_value', 'NONE');
#182870=CARTESIAN_POINT ( 'NONE',  ( 8.776573235218638303, 13.27486625357122385, -8.183627694784497919 ) ) ;
#182886=DIRECTION ( 'NONE',  ( -0.000000000000000000, -1.000000000000000000, -0.000000000000000000 ) ) ;
#182896=CARTESIAN_POINT ( 'NONE',  ( -11.84668730067608244, 12.59363775091779125, 1.399999999999998357 ) ) ;
#182909=CARTESIAN_POINT ( 'NONE',  ( -9.445420027513423022, 15.31879668566292985, -7.300025634049747580 ) ) ;
#182918=AXIS2_PLACEMENT_3D ( 'NONE', #90093, #106379, #123739 ) ;
#182945=PRESENTATION_STYLE_ASSIGNMENT (( #119084 ) ) ;
#182951=CARTESIAN_POINT ( 'NONE',  ( 8.766148990750032510, 13.42095518280116906, 8.127564194100379780 ) ) ;
#182990=CARTESIAN_POINT ( 'NONE',  ( 11.91292854676703961, 9.985184703269753825, -1.446370920797349635 ) ) ;
#183005=CARTESIAN_POINT ( 'NONE',  ( 8.030844283385320637, 15.33938070391476671, 8.918166425210744208 ) ) ;
#183008=CARTESIAN_POINT ( 'NONE',  ( -9.949568243101348131, 5.483630524090502334, 6.039417671888569039 ) ) ;
#183019=CARTESIAN_POINT ( 'NONE',  ( -11.44779964734699540, 10.99810470129610529, 3.599999963171390593 ) ) ;
#183034=CARTESIAN_POINT ( 'NONE',  ( -11.90624282132911382, 8.910973456084862576, -1.225840489975523306 ) ) ;
#183053=PRESENTATION_STYLE_ASSIGNMENT (( #35732 ) ) ;
#183064=DIRECTION ( 'NONE',  ( 3.491481338843133355E-15, 0.000000000000000000, 1.000000000000000000 ) ) ;
#183072=EDGE_CURVE ( 'NONE', #133821, #62106, #175514, .T. ) ;
#183080=ORIENTED_EDGE ( 'NONE', *, *, #73755, .F. ) ;
#183085=B_SPLINE_CURVE_WITH_KNOTS ( 'NONE', 3,
 ( #57324, #10684, #41094, #75704, #126669, #124546 ),
 .UNSPECIFIED., .F., .F.,
 ( 4, 2, 4 ),
 ( 0.000000000000000000, 0.0003767643964918269734, 0.0007535287929836536214 ),
 .UNSPECIFIED. ) ;
#183086=CARTESIAN_POINT ( 'NONE',  ( 0.000000000000000000, 13.79999999999998295, 0.000000000000000000 ) ) ;
#183094=CARTESIAN_POINT ( 'NONE',  ( -11.52901446936791352, 12.30574472532448205, -3.330874149801263062 ) ) ;
#183116=PRESENTATION_STYLE_ASSIGNMENT (( #144544 ) ) ;
#183122=FILL_AREA_STYLE ('',( #70407 ) ) ;
#183127=SURFACE_STYLE_FILL_AREA ( #84560 ) ;
#183135=EDGE_CURVE ( 'NONE', #182367, #84148, #74483, .T. ) ;
#183155=CYLINDRICAL_SURFACE ( 'NONE', #136735, 0.3999999999999997446 ) ;
#183186=CARTESIAN_POINT ( 'NONE',  ( -9.383668910029371091, 15.40608514343435509, -7.388226147498031082 ) ) ;
#183206=CARTESIAN_POINT ( 'NONE',  ( 11.84100621633422179, 12.48958425776664072, -1.444132586618106728 ) ) ;
#183211=EDGE_CURVE ( 'NONE', #161745, #166496, #28181, .T. ) ;
#183239=CARTESIAN_POINT ( 'NONE',  ( 11.94980361490495291, 11.00332124735860617, -1.099999952232860512 ) ) ;
#183269=DIRECTION ( 'NONE',  ( 0.000000000000000000, 1.000000000000000000, 0.000000000000000000 ) ) ;
#183276=VERTEX_POINT ( 'NONE', #46581 ) ;
#183288=CARTESIAN_POINT ( 'NONE',  ( -12.46228870304231329, 8.331136472732479703, -2.451782011337487965 ) ) ;
#183290=FACE_OUTER_BOUND ( 'NONE', #120256, .T. ) ;
#183316=DIRECTION ( 'NONE',  ( 0.000000000000000000, 1.804652791718263484E-16, -1.000000000000000000 ) ) ;
#183326=EDGE_CURVE ( 'NONE', #175615, #139393, #212695, .T. ) ;
#183342=CARTESIAN_POINT ( 'NONE',  ( 11.92619526913699879, 10.89999999999998259, 1.328859060402684644 ) ) ;
#183358=CARTESIAN_POINT ( 'NONE',  ( -10.91033920341459051, 4.885615726745599297, 4.996448585388897357 ) ) ;
#183379=( GEOMETRIC_REPRESENTATION_CONTEXT ( 3 ) GLOBAL_UNCERTAINTY_ASSIGNED_CONTEXT ( ( #68058 ) ) GLOBAL_UNIT_ASSIGNED_CONTEXT ( ( #89298, #5862, #41624 ) ) REPRESENTATION_CONTEXT ( 'NONE', 'WORKASPACE' ) );
#183400=CARTESIAN_POINT ( 'NONE',  ( -11.48243876534946040, 13.79999999999999893, -3.200000000000001510 ) ) ;
#183403=CARTESIAN_POINT ( 'NONE',  ( 7.836497216431498103, 13.95913530938479497, -9.964358386139231527 ) ) ;
#183409=ORIENTED_EDGE ( 'NONE', *, *, #182170, .T. ) ;
#183455=DIRECTION ( 'NONE',  ( 1.000000000000000000, -0.000000000000000000, -0.000000000000000000 ) ) ;
#183465=CARTESIAN_POINT ( 'NONE',  ( 11.84668730067608600, 13.40000000000000036, -1.400000000000001910 ) ) ;
#183468=CARTESIAN_POINT ( 'NONE',  ( 10.50000000000000178, 10.89999999999998259, 3.599999999999999201 ) ) ;
#183469=ORIENTED_EDGE ( 'NONE', *, *, #106403, .F. ) ;
#183471=CARTESIAN_POINT ( 'NONE',  ( -11.91826848330638455, 11.00729645956977798, 1.400000080589927753 ) ) ;
#183494=LINE ( 'NONE', #146773, #180786 ) ;
#183504=( LENGTH_UNIT ( ) NAMED_UNIT ( * ) SI_UNIT ( .MILLI., .METRE. ) );
#183506=CARTESIAN_POINT ( 'NONE',  ( -11.86687215968023601, 12.49057787694210653, -1.056395335932043045 ) ) ;
#183507=CARTESIAN_POINT ( 'NONE',  ( -11.12459591588106811, 5.815451121142331203, -4.514238076378977560 ) ) ;
#183515=STYLED_ITEM ( 'NONE', ( #165200 ), #169296 ) ;
#183516=CARTESIAN_POINT ( 'NONE',  ( -11.32461466721508181, 7.705894113993029038, 3.976347498773577183 ) ) ;
#183528=COLOUR_RGB ( '', 0.40784314, 0.44705882, 0.49803922) ;
#183529=ADVANCED_FACE ( 'NONE', ( #127917 ), #21524, .T. ) ;
#183534=( NAMED_UNIT ( * ) SI_UNIT ( $, .STERADIAN. ) SOLID_ANGLE_UNIT ( ) );
#183543=CARTESIAN_POINT ( 'NONE',  ( 6.743450862738472829, 15.00041888085534758, 9.536679667281278583 ) ) ;
#183558=EDGE_LOOP ( 'NONE', ( #65198, #208909, #157106, #208635 ) ) ;
#183564=CARTESIAN_POINT ( 'NONE',  ( -10.56514123924917392, 13.75891954478806234, -3.404988257269842222 ) ) ;
#183574=CARTESIAN_POINT ( 'NONE',  ( -11.84668730067608600, 12.69999999999998153, 1.399999999999998579 ) ) ;
#183600=DIRECTION ( 'NONE',  ( -0.000000000000000000, 1.000000000000000000, 0.000000000000000000 ) ) ;
#183608=EDGE_CURVE ( 'NONE', #101488, #142386, #65969, .T. ) ;
#183627=CIRCLE ( 'NONE', #41888, 12.00000000000000178 ) ;
#183635=( LENGTH_UNIT ( ) NAMED_UNIT ( * ) SI_UNIT ( .MILLI., .METRE. ) );
#183658=UNCERTAINTY_MEASURE_WITH_UNIT (LENGTH_MEASURE( 1.000000000000000082E-05 ), #205447, 'distance_accuracy_value', 'NONE');
#183685=CARTESIAN_POINT ( 'NONE',  ( -8.065673753977488758, 14.99999996918362832, -8.613976771944329869 ) ) ;
#183687=CARTESIAN_POINT ( 'NONE',  ( -9.986127180934126102, 5.615481227002261377, 5.966285604742011195 ) ) ;
#183731=AXIS2_PLACEMENT_3D ( 'NONE', #185064, #33501, #199173 ) ;
#183757=CARTESIAN_POINT ( 'NONE',  ( -15.75000000000000000, 10.90000000000000036, -0.7000000000000009548 ) ) ;
#183770=EDGE_CURVE ( 'NONE', #203495, #116100, #119089, .T. ) ;
#183783=CIRCLE ( 'NONE', #173473, 0.5000000000000008882 ) ;
#183787=CARTESIAN_POINT ( 'NONE',  ( -10.47097306639366820, 4.046871294038967726, -7.151610515452683003 ) ) ;
#183800=ORIENTED_EDGE ( 'NONE', *, *, #143084, .F. ) ;
#183803=CARTESIAN_POINT ( 'NONE',  ( 11.70317096822030400, 7.060310916292978689, -2.662588479640240813 ) ) ;
#183815=CARTESIAN_POINT ( 'NONE',  ( 9.285099613924293394, 13.38408970557267175, 6.770650828121584475 ) ) ;
#183818=ORIENTED_EDGE ( 'NONE', *, *, #156042, .T. ) ;
#183825=CARTESIAN_POINT ( 'NONE',  ( 6.902720183911292828, 14.55305236562704074, -9.761920501353824164 ) ) ;
#183826=CARTESIAN_POINT ( 'NONE',  ( 5.133413704082500385E-17, 15.44694763437295748, -11.95586206896552106 ) ) ;
#183827=VERTEX_POINT ( 'NONE', #57232 ) ;
#183845=EDGE_CURVE ( 'NONE', #129573, #175025, #19373, .T. ) ;
#183848=ORIENTED_EDGE ( 'NONE', *, *, #134782, .T. ) ;
#183877=( GEOMETRIC_REPRESENTATION_CONTEXT ( 3 ) GLOBAL_UNCERTAINTY_ASSIGNED_CONTEXT ( ( #103484 ) ) GLOBAL_UNIT_ASSIGNED_CONTEXT ( ( #172642, #108764, #192056 ) ) REPRESENTATION_CONTEXT ( 'NONE', 'WORKASPACE' ) );
#183878=ORIENTED_EDGE ( 'NONE', *, *, #96921, .T. ) ;
#183922=CARTESIAN_POINT ( 'NONE',  ( -11.97297122925985136, 9.801250793269115746, 0.8121202983519364427 ) ) ;
#183936=CARTESIAN_POINT ( 'NONE',  ( 11.48784849554594345, 12.26950472818075077, 3.469614872287801521 ) ) ;
#183962=CARTESIAN_POINT ( 'NONE',  ( -11.84100621633422179, 12.48958425776662118, 1.444132586618105174 ) ) ;
#183987=( NAMED_UNIT ( * ) PLANE_ANGLE_UNIT ( ) SI_UNIT ( $, .RADIAN. ) );
#184060=DIRECTION ( 'NONE',  ( 1.000000000000000000, -0.000000000000000000, -0.000000000000000000 ) ) ;
#184069=CARTESIAN_POINT ( 'NONE',  ( -9.915825940873133959, 4.173851563286998356, 6.175246223022227809 ) ) ;
#184079=CARTESIAN_POINT ( 'NONE',  ( 0.000000000000000000, 11.37999999999999901, 0.000000000000000000 ) ) ;
#184093=CARTESIAN_POINT ( 'NONE',  ( -11.29577547002741866, 7.647201583078615528, -3.921964478061291004 ) ) ;
#184144=CARTESIAN_POINT ( 'NONE',  ( -10.47222688565958926, 3.889612458557746510, 5.860485223248574016 ) ) ;
#184145=LINE ( 'NONE', #67180, #115148 ) ;
#184147=CARTESIAN_POINT ( 'NONE',  ( -11.84100621633422179, 13.61041574223336248, -1.444132586618106728 ) ) ;
#184150=( BOUNDED_SURFACE ( )  B_SPLINE_SURFACE ( 3, 2, ( 
 ( #128071, #180977, #111794 ),
 ( #96568, #13142, #98674 ),
 ( #145337, #177799, #28337 ),
 ( #29416, #211338, #147431 ),
 ( #64039, #94434, #130184 ),
 ( #196177, #47819, #179926 ) ),
 .UNSPECIFIED., .F., .F., .F. ) 
 B_SPLINE_SURFACE_WITH_KNOTS ( ( 4, 2, 4 ),
 ( 3, 3 ),
 ( 0.000000000000000000, 0.0003831327362561326704, 0.0007662654725122653408 ),
 ( 0.000000000000000000, 1.000000000000000000 ),
 .UNSPECIFIED. ) 
 GEOMETRIC_REPRESENTATION_ITEM ( )  RATIONAL_B_SPLINE_SURFACE ( (
 ( 1.000000000000000000, 0.5879095031487664436, 1.000000000000000000),
 ( 1.000000000000000000, 0.5873691247578739505, 1.000000000000000000),
 ( 1.000000000000000000, 0.6054349545497327290, 1.000000000000000000),
 ( 1.000000000000000000, 0.6533334602766750487, 1.000000000000000000),
 ( 1.000000000000000000, 0.6828746263150841100, 1.000000000000000000),
 ( 1.000000000000000000, 0.7071067811865475727, 1.000000000000000000) ) ) 
 REPRESENTATION_ITEM ( '' )  SURFACE ( )  );
#184152=CARTESIAN_POINT ( 'NONE',  ( -11.52483635780544624, 12.22000008642464941, -3.345866325258089358 ) ) ;
#184176=COLOUR_RGB ( '', 0.72549020, 0.75294118, 0.79215686) ;
#184179=( LENGTH_UNIT ( ) NAMED_UNIT ( * ) SI_UNIT ( .MILLI., .METRE. ) );
#184187=EDGE_CURVE ( 'NONE', #80885, #209385, #164324, .T. ) ;
#184210=CARTESIAN_POINT ( 'NONE',  ( -15.75000000000000000, 12.69999999999999929, -1.100000000000000311 ) ) ;
#184224=CARTESIAN_POINT ( 'NONE',  ( 10.59754597632703899, 11.29999999999999893, -3.303592501912006263 ) ) ;
#184239=CARTESIAN_POINT ( 'NONE',  ( 11.88237951145550220, 9.843193473787149372, 0.9087114598430685586 ) ) ;
#184247=CARTESIAN_POINT ( 'NONE',  ( -11.97181073603049661, 9.719999999999998863, 0.8318477717169566743 ) ) ;
#184261=CARTESIAN_POINT ( 'NONE',  ( 10.95308175811721085, 9.799999999999982947, 1.799999999999999600 ) ) ;
#184267=CARTESIAN_POINT ( 'NONE',  ( -11.81911962874442068, 12.34289426515883648, -1.591749704452499303 ) ) ;
#184282=CYLINDRICAL_SURFACE ( 'NONE', #34157, 0.08000000000000020983 ) ;
#184326=CARTESIAN_POINT ( 'NONE',  ( 11.33772467203874612, 10.09267152018149361, -3.600000000000000977 ) ) ;
#184331=COLOUR_RGB ( '', 0.09019608, 0.27058824, 0.51372549) ;
#184347=CARTESIAN_POINT ( 'NONE',  ( -11.91006458477769314, 5.204012295529565790, -4.700227299318338936 ) ) ;
#184349=DIRECTION ( 'NONE',  ( 0.9632918427306595976, 0.000000000000000000, 0.2684563758389253985 ) ) ;
#184350=( NAMED_UNIT ( * ) SI_UNIT ( $, .STERADIAN. ) SOLID_ANGLE_UNIT ( ) );
#184359=CARTESIAN_POINT ( 'NONE',  ( 12.12244102266335233, 8.055895858565015999, 3.199560920820632148 ) ) ;
#184373=CARTESIAN_POINT ( 'NONE',  ( 11.89197816957260478, 12.30000000000000071, -0.8055420615339534685 ) ) ;
#184399=SURFACE_STYLE_USAGE ( .BOTH. , #119480 ) ;
#184406=VECTOR ( 'NONE', #75762, 1000.000000000000000 ) ;
#184410=SURFACE_STYLE_FILL_AREA ( #89080 ) ;
#184411=CARTESIAN_POINT ( 'NONE',  ( 0.000000000000000000, 9.719999999999998863, 0.000000000000000000 ) ) ;
#184414=DIRECTION ( 'NONE',  ( 0.000000000000000000, 0.000000000000000000, -1.000000000000000000 ) ) ;
#184459=CARTESIAN_POINT ( 'NONE',  ( 7.449797558097145611, 15.00000000000000000, -10.26196259744787653 ) ) ;
#184478=MECHANICAL_DESIGN_GEOMETRIC_PRESENTATION_REPRESENTATION('',(#156843),#60024);
#184516=CARTESIAN_POINT ( 'NONE',  ( 11.89204169242350950, 13.79999999999999893, -0.8046421800350563869 ) ) ;
#184520=CARTESIAN_POINT ( 'NONE',  ( 6.902720183911290164, 14.55305236562705318, -9.761920501353818835 ) ) ;
#184523=CARTESIAN_POINT ( 'NONE',  ( 10.62873463776380056, 11.29999999999998117, 3.199999999999997957 ) ) ;
#184541=AXIS2_PLACEMENT_3D ( 'NONE', #112028, #29648, #147665 ) ;
#184563=B_SPLINE_CURVE_WITH_KNOTS ( 'NONE', 3,
 ( #70824, #116467, #182459, #168360, #86040, #66554 ),
 .UNSPECIFIED., .F., .F.,
 ( 4, 2, 4 ),
 ( 0.000000000000000000, 0.0003767643964918268649, 0.0007535287929836534046 ),
 .UNSPECIFIED. ) ;
#184564=CARTESIAN_POINT ( 'NONE',  ( -11.96535697748089078, 12.34737332935553944, -0.9148528286454110647 ) ) ;
#184577=FILL_AREA_STYLE ('',( #135855 ) ) ;
#184582=EDGE_CURVE ( 'NONE', #49028, #49203, #72129, .T. ) ;
#184604=ORIENTED_EDGE ( 'NONE', *, *, #175858, .F. ) ;
#184616=B_SPLINE_CURVE_WITH_KNOTS ( 'NONE', 3,
 ( #23618, #124429, #109231, #106004, #126556, #173104 ),
 .UNSPECIFIED., .F., .F.,
 ( 4, 2, 4 ),
 ( 0.000000000000000000, 0.0003239988925529259205, 0.0006479977851058518409 ),
 .UNSPECIFIED. ) ;
#184620=CARTESIAN_POINT ( 'NONE',  ( -10.50060100873255031, 5.377693802073529206, 5.808388628131297970 ) ) ;
#184630=PLANE ( 'NONE',  #97124 ) ;
#184660=PRESENTATION_STYLE_ASSIGNMENT (( #118676 ) ) ;
#184667=CARTESIAN_POINT ( 'NONE',  ( 0.000000000000000000, 11.29999999999999893, 0.000000000000000000 ) ) ;
#184671=EDGE_LOOP ( 'NONE', ( #203510, #50922, #142165, #81268 ) ) ;
#184689=DIRECTION ( 'NONE',  ( 0.000000000000000000, 0.000000000000000000, -1.000000000000000000 ) ) ;
#184731=CARTESIAN_POINT ( 'NONE',  ( 1.000000047849771034, 16.00000000000000711, -11.64874984998672680 ) ) ;
#184733=CARTESIAN_POINT ( 'NONE',  ( -11.52570357830391323, 8.091488070261075194, -2.173620758456770830 ) ) ;
#184741=CARTESIAN_POINT ( 'NONE',  ( -1.249999999999964695, 8.500000000000000000, -11.02939254900287303 ) ) ;
#184777=( NAMED_UNIT ( * ) SI_UNIT ( $, .STERADIAN. ) SOLID_ANGLE_UNIT ( ) );
#184778=DIRECTION ( 'NONE',  ( 0.000000000000000000, 1.000000000000000000, 0.000000000000000000 ) ) ;
#184809=CARTESIAN_POINT ( 'NONE',  ( 11.96217875511317885, 9.771456334210231631, 0.9561995067075056420 ) ) ;
#184810=CARTESIAN_POINT ( 'NONE',  ( 11.88235317400313917, 9.843357602269703577, -0.9089793033029952563 ) ) ;
#184836=DIRECTION ( 'NONE',  ( -0.000000000000000000, -1.000000000000000000, -0.000000000000000000 ) ) ;
#184837=CARTESIAN_POINT ( 'NONE',  ( -10.57449672806501262, 3.061848070889987561, -7.008429158759065913 ) ) ;
#184839=COLOUR_RGB ( '', 0.72549020, 0.75294118, 0.79215686) ;
#184851=DIRECTION ( 'NONE',  ( -8.881784197001252323E-15, 0.000000000000000000, 1.000000000000000000 ) ) ;
#184857=CARTESIAN_POINT ( 'NONE',  ( 11.75718816816947587, 6.923265086052656336, 2.447717586180979676 ) ) ;
#184861=ORIENTED_EDGE ( 'NONE', *, *, #80428, .F. ) ;
#184869=CARTESIAN_POINT ( 'NONE',  ( 8.815910235490386881, 13.32329502132428267, -7.673832123164161523 ) ) ;
#184877=TOROIDAL_SURFACE ( 'NONE', #25793, 11.18000000000000149, 0.08000000000000000167 ) ;
#184882=CARTESIAN_POINT ( 'NONE',  ( -4.795850263662800650, 15.51848109256882147, -11.00904932270169212 ) ) ;
#184886=MECHANICAL_DESIGN_GEOMETRIC_PRESENTATION_REPRESENTATION('',(#178131),#81168);
#184910=SURFACE_STYLE_FILL_AREA ( #120003 ) ;
#184922=CARTESIAN_POINT ( 'NONE',  ( 11.86145016429273191, 13.40000000000000036, -1.100000000000002087 ) ) ;
#184939=CARTESIAN_POINT ( 'NONE',  ( -15.75000000000000000, 10.89999999999998259, 3.599999999999999201 ) ) ;
#184968=EDGE_CURVE ( 'NONE', #97098, #207604, #97501, .T. ) ;
#185014=AXIS2_PLACEMENT_3D ( 'NONE', #207113, #107557, #124891 ) ;
#185024=UNCERTAINTY_MEASURE_WITH_UNIT (LENGTH_MEASURE( 1.000000000000000082E-05 ), #81896, 'distance_accuracy_value', 'NONE');
#185034=CIRCLE ( 'NONE', #119415, 0.08000000000000020983 ) ;
#185046=FACE_OUTER_BOUND ( 'NONE', #155631, .T. ) ;
#185052=DIRECTION ( 'NONE',  ( 0.000000000000000000, 0.000000000000000000, -1.000000000000000000 ) ) ;
#185064=CARTESIAN_POINT ( 'NONE',  ( -9.748756651352278979, 4.000007913748506283, -7.301653494139321410 ) ) ;
#185104=EDGE_CURVE ( 'NONE', #22427, #129544, #77562, .T. ) ;
#185122=VERTEX_POINT ( 'NONE', #175007 ) ;
#185126=CARTESIAN_POINT ( 'NONE',  ( -9.470186914265017464, 4.005096909781187264, 6.837150237413082365 ) ) ;
#185145=CIRCLE ( 'NONE', #39993, 11.09999999999999964 ) ;
#185170=DIRECTION ( 'NONE',  ( -0.000000000000000000, 0.000000000000000000, -1.000000000000000000 ) ) ;
#185176=CARTESIAN_POINT ( 'NONE',  ( -15.75000000000000000, 13.39999999999998259, 3.599999999999999201 ) ) ;
#185197=ORIENTED_EDGE ( 'NONE', *, *, #175333, .F. ) ;
#185202=SURFACE_STYLE_USAGE ( .BOTH. , #132248 ) ;
#185203=VERTEX_POINT ( 'NONE', #8209 ) ;
#185241=ADVANCED_FACE ( 'NONE', ( #45009 ), #177122, .F. ) ;
#185244=SURFACE_SIDE_STYLE ('',( #183127 ) ) ;
#185275=CARTESIAN_POINT ( 'NONE',  ( -10.28135750008142324, 4.005690466847553033, 7.422021812076344816 ) ) ;
#185278=UNCERTAINTY_MEASURE_WITH_UNIT (LENGTH_MEASURE( 1.000000000000000082E-05 ), #107039, 'distance_accuracy_value', 'NONE');
#185288=ORIENTED_EDGE ( 'NONE', *, *, #16807, .T. ) ;
#185292=ORIENTED_EDGE ( 'NONE', *, *, #60516, .F. ) ;
#185314=ORIENTED_EDGE ( 'NONE', *, *, #7913, .F. ) ;
#185327=ORIENTED_EDGE ( 'NONE', *, *, #110606, .T. ) ;
#185330=CARTESIAN_POINT ( 'NONE',  ( -10.79402553208788795, 4.457662888968881632, -5.246225075943923066 ) ) ;
#185336=CARTESIAN_POINT ( 'NONE',  ( -11.84668730067608422, 12.69999999999999929, -1.400000000000001688 ) ) ;
#185337=CARTESIAN_POINT ( 'NONE',  ( -11.89829993707161471, 9.770807717488722233, 1.561606677374347552 ) ) ;
#185344=AXIS2_PLACEMENT_3D ( 'NONE', #58411, #26957, #92001 ) ;
#185354=ORIENTED_EDGE ( 'NONE', *, *, #175553, .T. ) ;
#185361=CARTESIAN_POINT ( 'NONE',  ( -8.596519480563392435, 15.44749384048859930, -8.311898804283693210 ) ) ;
#185391=EDGE_LOOP ( 'NONE', ( #214031, #119106, #157883, #79013 ) ) ;
#185397=SPHERICAL_SURFACE ( 'NONE', #126386, 0.5000000000000001110 ) ;
#185414=CARTESIAN_POINT ( 'NONE',  ( -10.44369633504468631, 5.112959841837462882, -5.232137017608344820 ) ) ;
#185420=CARTESIAN_POINT ( 'NONE',  ( 11.88235317400313917, 12.34335760226970358, -0.9089793033029952563 ) ) ;
#185431=CIRCLE ( 'NONE', #213085, 0.07999999999999977962 ) ;
#185441=DIRECTION ( 'NONE',  ( 1.000000000000000000, -0.000000000000000000, -0.000000000000000000 ) ) ;
#185477=CARTESIAN_POINT ( 'NONE',  ( -1.499999999999960476, 7.000000000000000000, 10.99818166789401985 ) ) ;
#185496=ORIENTED_EDGE ( 'NONE', *, *, #79256, .T. ) ;
#185497=CARTESIAN_POINT ( 'NONE',  ( -15.75000000000000000, 12.29999999999998295, 3.199999999999997957 ) ) ;
#185503=COLOUR_RGB ( '', 0.40784314, 0.44705882, 0.49803922) ;
#185521=AXIS2_PLACEMENT_3D ( 'NONE', #136455, #74638, #56258 ) ;
#185525=CARTESIAN_POINT ( 'NONE',  ( 9.673880494682652653, 13.47554395514287684, -8.174421919205036247 ) ) ;
#185533=CARTESIAN_POINT ( 'NONE',  ( 1.734723475976807094E-15, 15.00041888085534758, 12.17999951260719982 ) ) ;
#185555=CARTESIAN_POINT ( 'NONE',  ( -10.47476534206535170, 5.237283261923990629, -5.169982392003922733 ) ) ;
#185559=CARTESIAN_POINT ( 'NONE',  ( 8.338567886252109318, 15.10332194136754680, -8.569227703174822963 ) ) ;
#185577=ORIENTED_EDGE ( 'NONE', *, *, #193910, .T. ) ;
#185580=CARTESIAN_POINT ( 'NONE',  ( 10.50000000000000178, 13.39999999999998259, 3.599999999999999201 ) ) ;
#185583=DIRECTION ( 'NONE',  ( -0.000000000000000000, 1.000000000000000000, -0.000000000000000000 ) ) ;
#185597=CARTESIAN_POINT ( 'NONE',  ( 11.89317557362582711, 12.33724156162407937, -1.599935658896034729 ) ) ;
#185610=AXIS2_PLACEMENT_3D ( 'NONE', #190579, #157048, #105102 ) ;
#185631=CARTESIAN_POINT ( 'NONE',  ( -11.01445754936173849, 5.351296611813540771, -4.769094010048264387 ) ) ;
#185641=CARTESIAN_POINT ( 'NONE',  ( -10.81128737566128528, 6.428770538698215020, 5.224633893128990181 ) ) ;
#185659=EDGE_CURVE ( 'NONE', #9995, #128985, #11179, .T. ) ;
#185662=ORIENTED_EDGE ( 'NONE', *, *, #120407, .F. ) ;
#185664=( GEOMETRIC_REPRESENTATION_CONTEXT ( 3 ) GLOBAL_UNCERTAINTY_ASSIGNED_CONTEXT ( ( #159191 ) ) GLOBAL_UNIT_ASSIGNED_CONTEXT ( ( #22164, #88279, #187893 ) ) REPRESENTATION_CONTEXT ( 'NONE', 'WORKASPACE' ) );
#185673=CARTESIAN_POINT ( 'NONE',  ( 0.000000000000000000, 14.48154074412737202, 0.000000000000000000 ) ) ;
#185720=FACE_OUTER_BOUND ( 'NONE', #28798, .T. ) ;
#185750=CARTESIAN_POINT ( 'NONE',  ( -15.75000000000000000, 13.79999999999999893, 0.6999999999999992895 ) ) ;
#185779=CARTESIAN_POINT ( 'NONE',  ( -15.75000000000000000, 10.90000000000000036, -1.400000000000001910 ) ) ;
#185803=CARTESIAN_POINT ( 'NONE',  ( -10.28823555840286552, 6.680969737303435352, 5.325637450257892702 ) ) ;
#185814=ORIENTED_EDGE ( 'NONE', *, *, #103222, .T. ) ;
#185816=ADVANCED_FACE ( 'NONE', ( #28516 ), #160650, .F. ) ;
#185822=CARTESIAN_POINT ( 'NONE',  ( -9.771731810572180876, 4.446950909175569677, 6.897090129977483386 ) ) ;
#185832=ORIENTED_EDGE ( 'NONE', *, *, #56390, .T. ) ;
#185834=SURFACE_STYLE_USAGE ( .BOTH. , #119856 ) ;
#185859=CARTESIAN_POINT ( 'NONE',  ( 6.902720183911293717, 15.44694763437295570, -9.761920501353824164 ) ) ;
#185894=ORIENTED_EDGE ( 'NONE', *, *, #72042, .F. ) ;
#185903=CARTESIAN_POINT ( 'NONE',  ( -11.97929049433705373, 11.37999999999999901, -0.7046979865771834106 ) ) ;
#185907=CARTESIAN_POINT ( 'NONE',  ( -10.40894566972866286, 4.029202461753065734, -7.241727701387177696 ) ) ;
#185923=CARTESIAN_POINT ( 'NONE',  ( 11.69944783379995812, 7.009427230352428317, -2.678979863565422725 ) ) ;
#185935=CARTESIAN_POINT ( 'NONE',  ( 10.75721414819643584, 8.375941707272300363, -4.789107451334092325 ) ) ;
#185942=CIRCLE ( 'NONE', #165236, 11.09999999999999964 ) ;
#185946=CARTESIAN_POINT ( 'NONE',  ( -9.340724465469280702, 15.44694763438213947, 7.462818192253868332 ) ) ;
#185949=CARTESIAN_POINT ( 'NONE',  ( -3.101822900477640754, 15.47022932557438324, -11.60075578494621595 ) ) ;
#185957=CARTESIAN_POINT ( 'NONE',  ( 10.59765138761703085, 9.799999999999982947, 3.303242380465396533 ) ) ;
#185991=DIRECTION ( 'NONE',  ( 0.000000000000000000, 0.000000000000000000, -1.000000000000000000 ) ) ;
#185995=CARTESIAN_POINT ( 'NONE',  ( -10.44369633504468631, 5.112959841837462882, -5.232137017608346596 ) ) ;
#185998=CARTESIAN_POINT ( 'NONE',  ( -15.75000000000000000, 10.89999999999998259, 1.399999999999998579 ) ) ;
#186020=SURFACE_SIDE_STYLE ('',( #157826 ) ) ;
#186060=DIRECTION ( 'NONE',  ( 0.000000000000000000, 0.000000000000000000, 1.000000000000000000 ) ) ;
#186063=CARTESIAN_POINT ( 'NONE',  ( 11.35569630219391968, 12.48731560708632138, 3.554478010595061743 ) ) ;
#186065=CARTESIAN_POINT ( 'NONE',  ( 9.452230854652610148, 11.00900109668812377, -7.398976902094164032 ) ) ;
#186069=CIRCLE ( 'NONE', #172338, 0.07999999999999946043 ) ;
#186074=ADVANCED_FACE ( 'NONE', ( #128246 ), #64223, .F. ) ;
#186082=ADVANCED_FACE ( 'NONE', ( #179046 ), #47996, .F. ) ;
#186112=CIRCLE ( 'NONE', #23449, 12.00000000000000178 ) ;
#186115=DIRECTION ( 'NONE',  ( 0.000000000000000000, 0.000000000000000000, 1.000000000000000000 ) ) ;
#186116=FILL_AREA_STYLE_COLOUR ( '', #30112 ) ;
#186120=DIRECTION ( 'NONE',  ( 1.000000000000000000, -0.000000000000000000, -0.000000000000000000 ) ) ;
#186145=CARTESIAN_POINT ( 'NONE',  ( -11.84100621633422179, 9.989584257766621178, 1.444132586618105174 ) ) ;
#186158=( GEOMETRIC_REPRESENTATION_CONTEXT ( 3 ) GLOBAL_UNCERTAINTY_ASSIGNED_CONTEXT ( ( #110212 ) ) GLOBAL_UNIT_ASSIGNED_CONTEXT ( ( #176099, #46106, #112224 ) ) REPRESENTATION_CONTEXT ( 'NONE', 'WORKASPACE' ) );
#186159=DIRECTION ( 'NONE',  ( 0.000000000000000000, 0.000000000000000000, -1.000000000000000000 ) ) ;
#186198=CARTESIAN_POINT ( 'NONE',  ( -9.645001968711920171, 4.042125922905831281, 6.587946042608958663 ) ) ;
#186204=AXIS2_PLACEMENT_3D ( 'NONE', #83158, #168688, #182794 ) ;
#186209=ORIENTED_EDGE ( 'NONE', *, *, #195119, .T. ) ;
#186294=CARTESIAN_POINT ( 'NONE',  ( 0.000000000000000000, 4.000000000000002665, 0.000000000000000000 ) ) ;
#186310=CARTESIAN_POINT ( 'NONE',  ( 6.882015208740342338, 14.48195938056239385, 9.732639244658489730 ) ) ;
#186335=EDGE_CURVE ( 'NONE', #135649, #55386, #126197, .T. ) ;
#186336=DIRECTION ( 'NONE',  ( 1.000000000000000000, 0.000000000000000000, -0.000000000000000000 ) ) ;
#186345=CARTESIAN_POINT ( 'NONE',  ( -10.21581353488473987, 4.000000000000001776, 7.512123095767014647 ) ) ;
#186367=CARTESIAN_POINT ( 'NONE',  ( -0.006200074199070590604, 15.44435154591194070, 11.95073779513205992 ) ) ;
#186374=CARTESIAN_POINT ( 'NONE',  ( -3.165656458280237118, 15.51990984979156352, 11.58349828325590991 ) ) ;
#186396=CARTESIAN_POINT ( 'NONE',  ( -10.84194285507322952, 4.687756354094246625, -5.144713108483911057 ) ) ;
#186408=AXIS2_PLACEMENT_3D ( 'NONE', #74465, #171967, #73378 ) ;
#186420=ORIENTED_EDGE ( 'NONE', *, *, #57578, .F. ) ;
#186422=CARTESIAN_POINT ( 'NONE',  ( 1.499999999999961364, 7.000000000000000000, -10.64483442802188939 ) ) ;
#186426=AXIS2_PLACEMENT_3D ( 'NONE', #88388, #104645, #122038 ) ;
#186444=FILL_AREA_STYLE_COLOUR ( '', #162317 ) ;
#186477=CARTESIAN_POINT ( 'NONE',  ( 10.98535488200954902, 13.75822556747230330, -1.593017372382192098 ) ) ;
#186486=CARTESIAN_POINT ( 'NONE',  ( -10.47476534206535170, 5.237283261923990629, -5.169982392003922733 ) ) ;
#186488=CARTESIAN_POINT ( 'NONE',  ( 11.41157692552970637, 13.75910337086997792, 3.404533818002357215 ) ) ;
#186513=LINE ( 'NONE', #86891, #13045 ) ;
#186597=DIRECTION ( 'NONE',  ( -0.000000000000000000, -1.000000000000000000, -0.000000000000000000 ) ) ;
#186600=CARTESIAN_POINT ( 'NONE',  ( 8.063487870853403905, 13.54606852283923857, -8.646108417490655285 ) ) ;
#186645=VERTEX_POINT ( 'NONE', #174543 ) ;
#186694=DIRECTION ( 'NONE',  ( 0.000000000000000000, -1.000000000000000000, 0.000000000000000000 ) ) ;
#186720=EDGE_LOOP ( 'NONE', ( #107717, #106341, #165427, #60477, #122689, #176237 ) ) ;
#186734=CARTESIAN_POINT ( 'NONE',  ( -11.48243876534946040, 13.88000000000000078, -3.200000000000001510 ) ) ;
#186769=CARTESIAN_POINT ( 'NONE',  ( -11.81451294207098179, 8.720850203416988577, 2.122579420461416344 ) ) ;
#186806=AXIS2_PLACEMENT_3D ( 'NONE', #172751, #90434, #206292 ) ;
#186813=ORIENTED_EDGE ( 'NONE', *, *, #48845, .F. ) ;
#186838=CARTESIAN_POINT ( 'NONE',  ( 0.000000000000000000, 15.00000000000000000, -12.00000000000000178 ) ) ;
#186845=CARTESIAN_POINT ( 'NONE',  ( 11.78331023100045627, 9.719999999999982876, 1.799999999999999600 ) ) ;
#186878=CARTESIAN_POINT ( 'NONE',  ( -10.05278092738192619, 5.876216011288541985, -5.831672646394378212 ) ) ;
#186883=EDGE_CURVE ( 'NONE', #115502, #16328, #132941, .T. ) ;
#186887=CARTESIAN_POINT ( 'NONE',  ( -11.04536101718726293, 10.19999999999999929, 1.099999999999996758 ) ) ;
#186909=DIRECTION ( 'NONE',  ( 1.000000000000000000, -0.000000000000000000, -0.000000000000000000 ) ) ;
#186920=FILL_AREA_STYLE_COLOUR ( '', #84143 ) ;
#186921=DIRECTION ( 'NONE',  ( 1.000000000000000000, -0.000000000000000000, -0.000000000000000000 ) ) ;
#186985=CARTESIAN_POINT ( 'NONE',  ( -10.41986968326957808, 5.020773655391575829, -5.279272669861445166 ) ) ;
#186997=SURFACE_SIDE_STYLE ('',( #134025 ) ) ;
#187003=CARTESIAN_POINT ( 'NONE',  ( 11.52860214534722694, 7.264370032338475447, 3.363647956867556132 ) ) ;
#187021=ADVANCED_FACE ( 'NONE', ( #99389 ), #200327, .T. ) ;
#187025=VERTEX_POINT ( 'NONE', #196876 ) ;
#187071=CARTESIAN_POINT ( 'NONE',  ( -10.47097306639366820, 4.046871294038967726, -7.151610515452683003 ) ) ;
#187173=FACE_OUTER_BOUND ( 'NONE', #38234, .T. ) ;
#187238=EDGE_CURVE ( 'NONE', #203495, #181928, #167545, .T. ) ;
#187257=CARTESIAN_POINT ( 'NONE',  ( -11.86145016429273014, 19.00000000000000000, -1.180000000000002158 ) ) ;
#187273=CARTESIAN_POINT ( 'NONE',  ( -9.420034542028389524, 2.999999999999999556, 6.906487091023606695 ) ) ;
#187287=DIRECTION ( 'NONE',  ( 0.7806247497458018714, 0.000000000000000000, -0.6250000000674432732 ) ) ;
#187304=LINE ( 'NONE', #84751, #191438 ) ;
#187315=DIRECTION ( 'NONE',  ( 0.000000000000000000, 1.000000000000000000, 0.000000000000000000 ) ) ;
#187323=CARTESIAN_POINT ( 'NONE',  ( -11.04536101718726293, 12.59542727035991661, 1.099999999999998757 ) ) ;
#187340=CIRCLE ( 'NONE', #166634, 0.07999999999999998779 ) ;
#187350=DIRECTION ( 'NONE',  ( 0.000000000000000000, 1.000000000000000000, 0.000000000000000000 ) ) ;
#187361=EDGE_LOOP ( 'NONE', ( #143180, #151118, #87411, #24872 ) ) ;
#187370=CARTESIAN_POINT ( 'NONE',  ( -3.058251533181919335, 15.44822376919687024, 11.56640689338974148 ) ) ;
#187380=CARTESIAN_POINT ( 'NONE',  ( 1.423205080756922314, 7.980384757729337863, 10.65537363484301459 ) ) ;
#187383=CARTESIAN_POINT ( 'NONE',  ( 11.82917762496792946, 7.768082351849152190, 1.754661222088528483 ) ) ;
#187404=EDGE_CURVE ( 'NONE', #182455, #13289, #15397, .T. ) ;
#187405=PRESENTATION_STYLE_ASSIGNMENT (( #138684 ) ) ;
#187416=CARTESIAN_POINT ( 'NONE',  ( -10.78913822082115281, 5.463154562124156399, 6.589184675844935057 ) ) ;
#187420=UNCERTAINTY_MEASURE_WITH_UNIT (LENGTH_MEASURE( 1.000000000000000082E-05 ), #37613, 'distance_accuracy_value', 'NONE');
#187432=DIRECTION ( 'NONE',  ( 0.000000000000000000, 0.000000000000000000, -1.000000000000000000 ) ) ;
#187434=( GEOMETRIC_REPRESENTATION_CONTEXT ( 3 ) GLOBAL_UNCERTAINTY_ASSIGNED_CONTEXT ( ( #140288 ) ) GLOBAL_UNIT_ASSIGNED_CONTEXT ( ( #112870, #213467, #192969 ) ) REPRESENTATION_CONTEXT ( 'NONE', 'WORKASPACE' ) );
#187449=DIRECTION ( 'NONE',  ( -0.000000000000000000, 1.000000000000000000, 0.000000000000000000 ) ) ;
#187460=CARTESIAN_POINT ( 'NONE',  ( 11.95359438122010864, 13.60421899708691562, 1.059536798430457338 ) ) ;
#187469=CARTESIAN_POINT ( 'NONE',  ( -9.906966810501817378, 3.509494795930026001, -6.775981647894812276 ) ) ;
#187493=ORIENTED_EDGE ( 'NONE', *, *, #153604, .F. ) ;
#187512=EDGE_CURVE ( 'NONE', #31691, #182472, #98443, .T. ) ;
#187532=FACE_OUTER_BOUND ( 'NONE', #102536, .T. ) ;
#187546=CARTESIAN_POINT ( 'NONE',  ( 11.01135777277262306, 13.40000000000000036, -1.400000000000001910 ) ) ;
#187552=CARTESIAN_POINT ( 'NONE',  ( -10.50660484223216606, 5.359830900411396648, 5.105327592218940502 ) ) ;
#187565=CARTESIAN_POINT ( 'NONE',  ( 11.15656239214823664, 9.703780284206802165, -5.826040129427457970 ) ) ;
#187568=ORIENTED_EDGE ( 'NONE', *, *, #79933, .F. ) ;
#187579=CARTESIAN_POINT ( 'NONE',  ( 11.94980361058169116, 12.70000000000000107, -1.099999999999998535 ) ) ;
#187609=ORIENTED_EDGE ( 'NONE', *, *, #208563, .T. ) ;
#187611=VERTEX_POINT ( 'NONE', #186422 ) ;
#187669=EDGE_LOOP ( 'NONE', ( #199404, #840, #102211, #174708 ) ) ;
#187681=CARTESIAN_POINT ( 'NONE',  ( 1.673491136019439323E-15, 15.00041888085534758, 11.67999951260719982 ) ) ;
#187682=ORIENTED_EDGE ( 'NONE', *, *, #56195, .T. ) ;
#187714=CARTESIAN_POINT ( 'NONE',  ( 7.854620613934385709, 15.31793777779468968, 9.015191429226655728 ) ) ;
#187716=VERTEX_POINT ( 'NONE', #37569 ) ;
#187725=CARTESIAN_POINT ( 'NONE',  ( -0.8988756482332411757, 14.48154074969179739, -11.99999999996309974 ) ) ;
#187732=EDGE_LOOP ( 'NONE', ( #110849, #78244, #65371, #188686 ) ) ;
#187735=B_SPLINE_CURVE_WITH_KNOTS ( 'NONE', 3,
 ( #184620, #84999, #168389, #70854, #19985, #136968 ),
 .UNSPECIFIED., .F., .F.,
 ( 4, 2, 4 ),
 ( 1.226634733346699349E-18, 0.0009740587311750446408, 0.001948117462350088197 ),
 .UNSPECIFIED. ) ;
#187779=CARTESIAN_POINT ( 'NONE',  ( -11.48243876534946040, 11.29999999999999893, -3.200000000000001510 ) ) ;
#187812=CARTESIAN_POINT ( 'NONE',  ( -11.55950211276791073, 9.799999999999998934, -3.221476510067115662 ) ) ;
#187824=CARTESIAN_POINT ( 'NONE',  ( 9.333041836227131682, 4.446947634373626279, -7.472413793103381607 ) ) ;
#187827=CARTESIAN_POINT ( 'NONE',  ( 11.04536101718726293, 12.69999999999999929, 1.099999999999996758 ) ) ;
#187834=CARTESIAN_POINT ( 'NONE',  ( -11.63182876714490632, 8.359486921846603025, 2.963400241755523634 ) ) ;
#187841=EDGE_CURVE ( 'NONE', #181174, #116397, #195387, .T. ) ;
#187893=( NAMED_UNIT ( * ) SI_UNIT ( $, .STERADIAN. ) SOLID_ANGLE_UNIT ( ) );
#187909=CARTESIAN_POINT ( 'NONE',  ( 7.825489347732291989, 14.97139610117899444, 9.977962224420885207 ) ) ;
#187929=CARTESIAN_POINT ( 'NONE',  ( 11.96212011828584387, 9.771875549500522951, 0.9569185076417748848 ) ) ;
#187942=CARTESIAN_POINT ( 'NONE',  ( -11.78039045457385292, 4.728130269440308453, 4.968650233931813709 ) ) ;
#187947=CARTESIAN_POINT ( 'NONE',  ( -10.97010717055062656, 12.30000000000000249, -1.696399592028410952 ) ) ;
#187949=AXIS2_PLACEMENT_3D ( 'NONE', #193733, #81058, #197992 ) ;
#187962=CARTESIAN_POINT ( 'NONE',  ( -10.49167311136684511, 5.343773310534622567, 5.730690286876297002 ) ) ;
#187975=CARTESIAN_POINT ( 'NONE',  ( 9.348381460497192208, 13.52536904890506264, 7.450314784081288444 ) ) ;
#187986=DIRECTION ( 'NONE',  ( 0.000000000000000000, 0.000000000000000000, 1.000000000000000000 ) ) ;
#188013=EDGE_LOOP ( 'NONE', ( #37278, #93181, #122539, #186420 ) ) ;
#188035=COLOUR_RGB ( '', 0.66274510, 0.83137255, 0.94901961) ;
#188037=ORIENTED_EDGE ( 'NONE', *, *, #200653, .T. ) ;
#188054=ORIENTED_EDGE ( 'NONE', *, *, #140722, .F. ) ;
#188061=CARTESIAN_POINT ( 'NONE',  ( -10.16814981310353616, 6.288261174334121684, -5.589887627215723853 ) ) ;
#188067=CARTESIAN_POINT ( 'NONE',  ( 8.809690371089201832, 13.28836970969089393, 8.148114100277203065 ) ) ;
#188090=FACE_OUTER_BOUND ( 'NONE', #175653, .T. ) ;
#188106=SURFACE_SIDE_STYLE ('',( #150296 ) ) ;
#188135=CARTESIAN_POINT ( 'NONE',  ( 1.333449616921239089, 8.249651149236392200, 11.01993490927446828 ) ) ;
#188140=CARTESIAN_POINT ( 'NONE',  ( -10.48363756508902611, 5.078564944783316548, -7.119907325005036647 ) ) ;
#188144=EDGE_CURVE ( 'NONE', #116165, #94694, #79034, .T. ) ;
#188217=CARTESIAN_POINT ( 'NONE',  ( -11.86145016429273014, 13.40000000000000036, -1.100000000000002087 ) ) ;
#188258=CARTESIAN_POINT ( 'NONE',  ( 11.48243876534946217, 13.79999999999998295, 3.199999999999997957 ) ) ;
#188265=SURFACE_STYLE_USAGE ( .BOTH. , #122307 ) ;
#188299=ORIENTED_EDGE ( 'NONE', *, *, #52780, .F. ) ;
#188310=CARTESIAN_POINT ( 'NONE',  ( 9.452953479610789245, 4.518459255872631530, 7.393264888175490768 ) ) ;
#188318=LINE ( 'NONE', #154772, #121119 ) ;
#188338=CARTESIAN_POINT ( 'NONE',  ( -10.39851513827935747, 3.504673854002353206, 5.419231829292963099 ) ) ;
#188340=DIRECTION ( 'NONE',  ( 1.000000000000000000, -0.000000000000000000, -0.000000000000000000 ) ) ;
#188347=ORIENTED_EDGE ( 'NONE', *, *, #66268, .F. ) ;
#188369=VERTEX_POINT ( 'NONE', #99407 ) ;
#188377=CARTESIAN_POINT ( 'NONE',  ( 0.000000000000000000, 4.446947634372835800, 0.000000000000000000 ) ) ;
#188378=( NAMED_UNIT ( * ) PLANE_ANGLE_UNIT ( ) SI_UNIT ( $, .RADIAN. ) );
#188384=FACE_OUTER_BOUND ( 'NONE', #141246, .T. ) ;
#188390=CARTESIAN_POINT ( 'NONE',  ( -3.098866152801546647, 14.55178984617735694, 11.55550500168035555 ) ) ;
#188409=VERTEX_POINT ( 'NONE', #149214 ) ;
#188437=CARTESIAN_POINT ( 'NONE',  ( -4.337327078093950128, 15.44737643973769359, 11.15018912635215464 ) ) ;
#188443=CIRCLE ( 'NONE', #95096, 11.09999999999999964 ) ;
#188451=CARTESIAN_POINT ( 'NONE',  ( 0.000000000000000000, 12.30000000000000071, 0.000000000000000000 ) ) ;
#188453=CARTESIAN_POINT ( 'NONE',  ( 10.19631792989279084, 10.81030520795681582, -6.241902085265002675 ) ) ;
#188457=EDGE_CURVE ( 'NONE', #150697, #66179, #166534, .T. ) ;
#188477=CARTESIAN_POINT ( 'NONE',  ( -15.75000000000000000, 13.40000000000000036, -1.400000000000001910 ) ) ;
#188487=CARTESIAN_POINT ( 'NONE',  ( -10.47051000334347570, 4.046481986658133856, 7.152373939818348347 ) ) ;
#188537=CARTESIAN_POINT ( 'NONE',  ( -11.06299035296667732, 12.34316295623905191, -0.9087041361035911313 ) ) ;
#188548=DIRECTION ( 'NONE',  ( 0.000000000000000000, -7.254698431504949604E-17, 1.000000000000000000 ) ) ;
#188573=ORIENTED_EDGE ( 'NONE', *, *, #22230, .F. ) ;
#188610=CIRCLE ( 'NONE', #26103, 0.07999999999999998779 ) ;
#188611=EDGE_LOOP ( 'NONE', ( #183878, #73253, #115117, #57518 ) ) ;
#188623=CARTESIAN_POINT ( 'NONE',  ( -10.60630588279735242, 5.715763139788331948, 4.896273837757428637 ) ) ;
#188626=CARTESIAN_POINT ( 'NONE',  ( -11.49966000274969602, 9.857671544352443860, 3.429881629453267244 ) ) ;
#188628=DIRECTION ( 'NONE',  ( -0.7806247334443685570, 0.000000000000000000, -0.6250000204279265725 ) ) ;
#188631=AXIS2_PLACEMENT_3D ( 'NONE', #179369, #97066, #163119 ) ;
#188653=DIRECTION ( 'NONE',  ( -1.124869321039521280E-29, -7.437565543542506798E-15, 1.000000000000000000 ) ) ;
#188686=ORIENTED_EDGE ( 'NONE', *, *, #33483, .F. ) ;
#188691=FILL_AREA_STYLE_COLOUR ( '', #126348 ) ;
#188696=DIRECTION ( 'NONE',  ( 0.000000000000000000, 0.000000000000000000, -1.000000000000000000 ) ) ;
#188744=EDGE_LOOP ( 'NONE', ( #29273, #106868, #161072, #9046 ) ) ;
#188773=AXIS2_PLACEMENT_3D ( 'NONE', #3953, #71093, #184851 ) ;
#188780=CARTESIAN_POINT ( 'NONE',  ( -10.72645012907092443, 4.497370833040986504, 5.281782792447082819 ) ) ;
#188789=SURFACE_STYLE_USAGE ( .BOTH. , #141528 ) ;
#188796=( LENGTH_UNIT ( ) NAMED_UNIT ( * ) SI_UNIT ( .MILLI., .METRE. ) );
#188802=CARTESIAN_POINT ( 'NONE',  ( -8.135612300829253130, 14.55183989155882784, -8.805242580674113029 ) ) ;
#188838=DIRECTION ( 'NONE',  ( -0.1652856342098213693, 0.9636458296411444246, -0.2099223050061321261 ) ) ;
#188872=CARTESIAN_POINT ( 'NONE',  ( 1.500000000000037748, 8.500000000000000000, 10.64483442802188051 ) ) ;
#188884=CARTESIAN_POINT ( 'NONE',  ( -11.44779963594995387, 10.19999999999999041, -3.600000000000078693 ) ) ;
#188887=EDGE_LOOP ( 'NONE', ( #19480, #11957, #91578, #178655 ) ) ;
#188893=ORIENTED_EDGE ( 'NONE', *, *, #195389, .F. ) ;
#188898=CARTESIAN_POINT ( 'NONE',  ( -0.01716059204523777415, 15.45541796569955650, 11.96980914358345061 ) ) ;
#188901=STYLED_ITEM ( 'NONE', ( #200306 ), #99019 ) ;
#188905=B_SPLINE_CURVE_WITH_KNOTS ( 'NONE', 3,
 ( #23247, #40608, #155407, #158619, #140260, #123014 ),
 .UNSPECIFIED., .F., .F.,
 ( 4, 2, 4 ),
 ( 0.000000000000000000, 0.0003258677429877275783, 0.0006517354859754551566 ),
 .UNSPECIFIED. ) ;
#188906=CARTESIAN_POINT ( 'NONE',  ( -10.81324141427316299, 6.418649203030321715, 5.206428076515513759 ) ) ;
#188910=STYLED_ITEM ( 'NONE', ( #56046 ), #146365 ) ;
#188966=DIRECTION ( 'NONE',  ( 0.000000000000000000, 1.000000000000000000, 0.000000000000000000 ) ) ;
#188977=CARTESIAN_POINT ( 'NONE',  ( 11.47453837139429211, 7.808021129890302170, -3.623698920762073783 ) ) ;
#188982=DIRECTION ( 'NONE',  ( 1.000000000000000000, -0.000000000000000000, -0.000000000000000000 ) ) ;
#188984=CARTESIAN_POINT ( 'NONE',  ( 7.576886519560940947, 14.99604748842864410, 10.16829559912798686 ) ) ;
#189006=ADVANCED_FACE ( 'NONE', ( #46669 ), #13067, .F. ) ;
#189007=CARTESIAN_POINT ( 'NONE',  ( 11.94105721839851952, 10.07301656658867195, 1.187919402540718927 ) ) ;
#189021=CARTESIAN_POINT ( 'NONE',  ( -11.76695491367977375, 4.673720869072629291, 4.995412848167406494 ) ) ;
#189030=PLANE ( 'NONE',  #160288 ) ;
#189039=ADVANCED_FACE ( 'NONE', ( #2123 ), #153745, .F. ) ;
#189125=ORIENTED_EDGE ( 'NONE', *, *, #67738, .F. ) ;
#189141=CARTESIAN_POINT ( 'NONE',  ( -11.15867860892636365, 6.757705308438493041, -5.812542620506402358 ) ) ;
#189146=TOROIDAL_SURFACE ( 'NONE', #88822, 11.92000000000000171, 0.08000000000000000167 ) ;
#189168=ORIENTED_EDGE ( 'NONE', *, *, #181087, .F. ) ;
#189173=CIRCLE ( 'NONE', #40461, 0.07999999999999940492 ) ;
#189210=CYLINDRICAL_SURFACE ( 'NONE', #148346, 0.3999999999999997446 ) ;
#189215=CARTESIAN_POINT ( 'NONE',  ( -9.399770542442999144, 4.999985930147239799, -6.933469103752857521 ) ) ;
#189269=EDGE_LOOP ( 'NONE', ( #29439, #106425, #37049, #45521 ) ) ;
#189279=CARTESIAN_POINT ( 'NONE',  ( 11.96786122759180770, 6.617496858734535969, 1.004052467025347006 ) ) ;
#189293=CARTESIAN_POINT ( 'NONE',  ( -11.86686399458719343, 13.60928729775336699, -1.056461745586973811 ) ) ;
#189299=EDGE_LOOP ( 'NONE', ( #132398, #30184, #61990, #70024 ) ) ;
#189306=AXIS2_PLACEMENT_3D ( 'NONE', #200946, #203085, #167421 ) ;
#189314=CARTESIAN_POINT ( 'NONE',  ( 11.86685672517501899, 11.10918917859810584, 1.056525322636017172 ) ) ;
#189330=DIRECTION ( 'NONE',  ( 1.000000000000000000, 0.000000000000000000, -0.000000000000000000 ) ) ;
#189333=MECHANICAL_DESIGN_GEOMETRIC_PRESENTATION_REPRESENTATION('',(#89015),#85428);
#189349=SURFACE_STYLE_FILL_AREA ( #57224 ) ;
#189375=MECHANICAL_DESIGN_GEOMETRIC_PRESENTATION_REPRESENTATION('',(#144441),#47625);
#189393=FACE_OUTER_BOUND ( 'NONE', #145234, .T. ) ;
#189409=CARTESIAN_POINT ( 'NONE',  ( -11.94651559118242368, 13.65130655878970956, 1.135242698369626435 ) ) ;
#189410=CARTESIAN_POINT ( 'NONE',  ( -11.23957921816311512, 4.929848952671569862, 5.866464787178605533 ) ) ;
#189421=EDGE_CURVE ( 'NONE', #108640, #115330, #42144, .T. ) ;
#189422=PRODUCT_DEFINITION ( 'UNKNOWN', '', #90350, #82879 ) ;
#189425=DIRECTION ( 'NONE',  ( 1.000000000000000000, -0.000000000000000000, -0.000000000000000000 ) ) ;
#189445=EDGE_LOOP ( 'NONE', ( #199474, #23842, #168102, #156413 ) ) ;
#189453=PRESENTATION_STYLE_ASSIGNMENT (( #58391 ) ) ;
#189490=CARTESIAN_POINT ( 'NONE',  ( -11.07790593930098311, 11.29999999999999893, 0.6999999999999992895 ) ) ;
#189506=CYLINDRICAL_SURFACE ( 'NONE', #87634, 0.07999999999999998779 ) ;
#189520=CARTESIAN_POINT ( 'NONE',  ( 10.65587894154546511, 9.861925906080523774, -5.419733535610468778 ) ) ;
#189551=CARTESIAN_POINT ( 'NONE',  ( -0.03257979115088098510, 15.47115322108842328, 11.98509113246685409 ) ) ;
#189552=CARTESIAN_POINT ( 'NONE',  ( -10.14895191633106819, 5.000000000000002665, 7.601392964450658596 ) ) ;
#189562=AXIS2_PLACEMENT_3D ( 'NONE', #74665, #208902, #155921 ) ;
#189603=CARTESIAN_POINT ( 'NONE',  ( -9.569358774130440892, 3.553060279300377822, -7.167287524826073231 ) ) ;
#189608=CARTESIAN_POINT ( 'NONE',  ( -11.86239285000045740, 11.29999999999998295, 1.812080536912751061 ) ) ;
#189614=CARTESIAN_POINT ( 'NONE',  ( 11.41381675112460847, 11.03016735491475941, -3.704697986577268232 ) ) ;
#189619=CIRCLE ( 'NONE', #148193, 12.00000000000000178 ) ;
#189667=CARTESIAN_POINT ( 'NONE',  ( 11.41381678389391574, 10.07120581758926647, -3.704697885617874942 ) ) ;
#189686=SURFACE_SIDE_STYLE ('',( #155067 ) ) ;
#189687=CARTESIAN_POINT ( 'NONE',  ( -10.48267169704037727, 5.268073273308885973, 5.153989745587932880 ) ) ;
#189689=CARTESIAN_POINT ( 'NONE',  ( -11.41381678389398502, 10.07120581758917233, 3.704697885617667996 ) ) ;
#189713=CARTESIAN_POINT ( 'NONE',  ( -10.95308175811721085, 9.799999999999998934, -1.800000000000001155 ) ) ;
#189716=CARTESIAN_POINT ( 'NONE',  ( -15.75000000000000000, 13.40000000000000036, -1.100000000000002087 ) ) ;
#189775=CARTESIAN_POINT ( 'NONE',  ( -1.499999999999960476, 7.000000000000000000, -10.99818166789402163 ) ) ;
#189784=CIRCLE ( 'NONE', #20312, 0.07999999999999971023 ) ;
#189798=CARTESIAN_POINT ( 'NONE',  ( 7.988145303641245754, 15.26989286654994693, 8.896987721899689561 ) ) ;
#189810=UNCERTAINTY_MEASURE_WITH_UNIT (LENGTH_MEASURE( 1.000000000000000082E-05 ), #31192, 'distance_accuracy_value', 'NONE');
#189834=EDGE_CURVE ( 'NONE', #180747, #21587, #185145, .T. ) ;
#189840=ORIENTED_EDGE ( 'NONE', *, *, #26426, .T. ) ;
#189860=CARTESIAN_POINT ( 'NONE',  ( 11.84668730067608600, 13.39999999999998259, 1.399999999999998579 ) ) ;
#189888=EDGE_CURVE ( 'NONE', #181635, #109578, #32215, .T. ) ;
#189913=CARTESIAN_POINT ( 'NONE',  ( -11.86685672517501899, 12.49081082140188670, 1.056525322636010289 ) ) ;
#189922=FACE_OUTER_BOUND ( 'NONE', #157743, .T. ) ;
#189927=ORIENTED_EDGE ( 'NONE', *, *, #121060, .T. ) ;
#189949=CARTESIAN_POINT ( 'NONE',  ( 10.90597896324554306, 8.126158609150163414, 4.424724984770519676 ) ) ;
#189952=CARTESIAN_POINT ( 'NONE',  ( -11.44779964734733113, 10.10189529870398850, -3.599999963171534478 ) ) ;
#189965=CARTESIAN_POINT ( 'NONE',  ( 9.405838923370980709, 3.553052382341641113, -7.381490207074687504 ) ) ;
#190027=CYLINDRICAL_SURFACE ( 'NONE', #39168, 0.3999999999999997446 ) ;
#190045=CARTESIAN_POINT ( 'NONE',  ( 6.928203230275525648, 15.00000000000000000, -9.797958971132702644 ) ) ;
#190050=CARTESIAN_POINT ( 'NONE',  ( 8.964365016547233722, 14.59103508737832300, -8.971863053630826812 ) ) ;
#190052=CARTESIAN_POINT ( 'NONE',  ( 10.07786606378326688, 13.99524484309983130, 7.406424912067739896 ) ) ;
#190085=CARTESIAN_POINT ( 'NONE',  ( -12.45759369916135029, 8.320971494343229580, 2.471636155840711169 ) ) ;
#190104=ORIENTED_EDGE ( 'NONE', *, *, #154690, .T. ) ;
#190197=CARTESIAN_POINT ( 'NONE',  ( -11.15881748666195072, 6.758040191959135079, 5.811769976250384495 ) ) ;
#190215=CARTESIAN_POINT ( 'NONE',  ( -11.01135777277262129, 10.19999999999998153, 1.399999999999998579 ) ) ;
#190216=ADVANCED_FACE ( 'NONE', ( #79939 ), #28000, .F. ) ;
#190264=SURFACE_SIDE_STYLE ('',( #141576 ) ) ;
#190270=CARTESIAN_POINT ( 'NONE',  ( -10.14895191580505163, 4.000029896383376027, -7.601392964056682189 ) ) ;
#190318=DIRECTION ( 'NONE',  ( 0.000000000000000000, 0.2129637811552522741, -0.9770600943217657708 ) ) ;
#190345=EDGE_LOOP ( 'NONE', ( #77548, #75065, #204600, #200600 ) ) ;
#190360=ORIENTED_EDGE ( 'NONE', *, *, #133034, .T. ) ;
#190369=CARTESIAN_POINT ( 'NONE',  ( -10.62729803237054149, 4.099240035649311942, -5.576248508406539628 ) ) ;
#190372=CARTESIAN_POINT ( 'NONE',  ( -9.417400627377789490, 14.63813357754229294, -7.338645108920092142 ) ) ;
#190387=PRESENTATION_STYLE_ASSIGNMENT (( #57205 ) ) ;
#190420=B_SPLINE_CURVE_WITH_KNOTS ( 'NONE', 3,
 ( #25097, #9918, #59739, #111761, #191856, #95477, #75992, #208110, #128040, #211308, #177767, #161525, #125897, #10972 ),
 .UNSPECIFIED., .F., .F.,
 ( 4, 2, 2, 2, 2, 2, 4 ),
 ( -5.999999999644659878E-08, 0.0007540416219186539450, 0.001508143243837304498, 0.001885194054796629666, 0.002262244865755954834, 0.002639295676715280002, 0.003016346487674605170 ),
 .UNSPECIFIED. ) ;
#190426=CARTESIAN_POINT ( 'NONE',  ( -9.569358774130488854, 4.446955548196734220, -7.167287524826102540 ) ) ;
#190444=EDGE_CURVE ( 'NONE', #16927, #181635, #1769, .T. ) ;
#190463=CARTESIAN_POINT ( 'NONE',  ( -9.978677811866239367, 3.146997876264563843, 6.103086072356673775 ) ) ;
#190472=STYLED_ITEM ( 'NONE', ( #65612 ), #163756 ) ;
#190536=ORIENTED_EDGE ( 'NONE', *, *, #38452, .F. ) ;
#190542=CARTESIAN_POINT ( 'NONE',  ( 1.477171894776290046E-15, 15.32408086029860428, 11.75104470124082034 ) ) ;
#190561=CARTESIAN_POINT ( 'NONE',  ( -7.079625160978284093, 15.44809611314506803, 9.644241769956890309 ) ) ;
#190572=DIRECTION ( 'NONE',  ( -0.000000000000000000, -1.000000000000000000, -0.000000000000000000 ) ) ;
#190579=CARTESIAN_POINT ( 'NONE',  ( 0.000000000000000000, 9.799999999999998934, 0.000000000000000000 ) ) ;
#190607=EDGE_LOOP ( 'NONE', ( #52353, #169085, #201454, #213549 ) ) ;
#190621=SURFACE_SIDE_STYLE ('',( #174417 ) ) ;
#190658=CARTESIAN_POINT ( 'NONE',  ( -11.33772463945036968, 10.09088423488573838, -3.600000000000000977 ) ) ;
#190669=CARTESIAN_POINT ( 'NONE',  ( 11.86686399458719521, 13.60928729775337054, 1.056461745586970258 ) ) ;
#190694=EDGE_LOOP ( 'NONE', ( #176856, #4997, #26895, #121484 ) ) ;
#190702=CARTESIAN_POINT ( 'NONE',  ( -11.55950211276791428, 11.37999999999999901, -3.221476510067114329 ) ) ;
#190724=CARTESIAN_POINT ( 'NONE',  ( -11.84668730067608600, 10.19999999999999929, -1.400000000000001910 ) ) ;
#190727=CARTESIAN_POINT ( 'NONE',  ( -11.92619526913699879, 13.40000000000000036, -1.328859060402686199 ) ) ;
#190751=CARTESIAN_POINT ( 'NONE',  ( -11.94980361490462428, 10.09667875264143255, -1.099999952232860290 ) ) ;
#190767=CARTESIAN_POINT ( 'NONE',  ( -11.49966000274973155, 13.74232845564745276, -3.429881629453017222 ) ) ;
#190768=ADVANCED_FACE ( 'NONE', ( #87984 ), #67621, .T. ) ;
#190794=ORIENTED_EDGE ( 'NONE', *, *, #85069, .F. ) ;
#190855=CARTESIAN_POINT ( 'NONE',  ( 9.255591775348552375, 14.20198051862420385, 7.641521890740467171 ) ) ;
#190863=DIRECTION ( 'NONE',  ( -0.000000000000000000, 1.000000000000000000, -0.000000000000000000 ) ) ;
#190871=CARTESIAN_POINT ( 'NONE',  ( 11.89835103415199313, 9.771069141675322811, 1.561208891256346876 ) ) ;
#190876=ORIENTED_EDGE ( 'NONE', *, *, #208132, .T. ) ;
#190894=MECHANICAL_DESIGN_GEOMETRIC_PRESENTATION_REPRESENTATION('',(#73224),#42186);
#190916=CARTESIAN_POINT ( 'NONE',  ( -10.45911201557330195, 5.175391108250987138, -5.201428006079835242 ) ) ;
#190924=AXIS2_PLACEMENT_3D ( 'NONE', #34569, #148341, #149396 ) ;
#190985=ORIENTED_EDGE ( 'NONE', *, *, #110539, .F. ) ;
#190990=CARTESIAN_POINT ( 'NONE',  ( -11.55950211276791251, 13.87999999999998302, 3.221476510067112109 ) ) ;
#191001=CARTESIAN_POINT ( 'NONE',  ( 8.353377556026719830, 13.12787966248234994, -8.539254890958119404 ) ) ;
#191009=VERTEX_POINT ( 'NONE', #106422 ) ;
#191013=CARTESIAN_POINT ( 'NONE',  ( -11.92619526913699879, 10.19999999999998153, 1.328859060402684644 ) ) ;
#191018=MECHANICAL_DESIGN_GEOMETRIC_PRESENTATION_REPRESENTATION('',(#94122),#114879);
#191021=LINE ( 'NONE', #207282, #117335 ) ;
#191040=STYLED_ITEM ( 'NONE', ( #9048 ), #133060 ) ;
#191061=CARTESIAN_POINT ( 'NONE',  ( -6.671583288098617892, 15.00000000000324718, 9.747470831330359076 ) ) ;
#191082=FILL_AREA_STYLE ('',( #208400 ) ) ;
#191096=B_SPLINE_CURVE_WITH_KNOTS ( 'NONE', 3,
 ( #42740, #108845, #144526, #77341, #193225, #209451 ),
 .UNSPECIFIED., .F., .F.,
 ( 4, 2, 4 ),
 ( 0.001877801214402442754, 0.002190719108449961511, 0.002503637002497480051 ),
 .UNSPECIFIED. ) ;
#191101=CARTESIAN_POINT ( 'NONE',  ( 12.00094528747601430, 6.998582067892187730, -0.9367503912666700350 ) ) ;
#191108=CARTESIAN_POINT ( 'NONE',  ( 9.165183341830644537, 14.44137815449902895, 8.758053443030863860 ) ) ;
#191109=( BOUNDED_CURVE ( )  B_SPLINE_CURVE ( 3, ( #77020, #44555, #74907, #57591 ),
 .UNSPECIFIED., .F., .T. ) 
 B_SPLINE_CURVE_WITH_KNOTS ( ( 4, 4 ),
 ( 4.576839133004758864, 4.599536981099443977 ),
 .UNSPECIFIED. ) 
 CURVE ( )  GEOMETRIC_REPRESENTATION_ITEM ( )  RATIONAL_B_SPLINE_CURVE ( ( 1.000000000000000000, 0.9999570677684579412, 0.9999570677684579412, 1.000000000000000000 ) ) 
 REPRESENTATION_ITEM ( '' )  );
#191127=CARTESIAN_POINT ( 'NONE',  ( 11.94105721237523277, 10.19999999999999929, 1.187919463087245386 ) ) ;
#191132=PRESENTATION_STYLE_ASSIGNMENT (( #193283 ) ) ;
#191142=CARTESIAN_POINT ( 'NONE',  ( -10.93377262805118555, 5.994763374826558966, -6.297255446303106297 ) ) ;
#191156=CARTESIAN_POINT ( 'NONE',  ( -15.75000000000000000, 13.79999999999999893, 0.6999999999999992895 ) ) ;
#191168=CARTESIAN_POINT ( 'NONE',  ( 9.397486876216097684, 13.53113053364065443, 7.462549781540802840 ) ) ;
#191194=TOROIDAL_SURFACE ( 'NONE', #66553, 11.92000000000000171, 0.08000000000000000167 ) ;
#191199=EDGE_CURVE ( 'NONE', #73222, #83914, #57907, .T. ) ;
#191224=AXIS2_PLACEMENT_3D ( 'NONE', #78348, #113064, #112001 ) ;
#191247=SURFACE_STYLE_FILL_AREA ( #125287 ) ;
#191255=CARTESIAN_POINT ( 'NONE',  ( -10.87640920097716091, 5.776148811624420176, 6.414305308649663750 ) ) ;
#191260=CARTESIAN_POINT ( 'NONE',  ( 9.020730412796739373, 12.35293633087048271, 7.916875519941681816 ) ) ;
#191328=CARTESIAN_POINT ( 'NONE',  ( -9.505468521307150809, 5.017170101577987928, -6.783879874543660371 ) ) ;
#191345=AXIS2_PLACEMENT_3D ( 'NONE', #120034, #2979, #88544 ) ;
#191386=ORIENTED_EDGE ( 'NONE', *, *, #147671, .T. ) ;
#191397=CARTESIAN_POINT ( 'NONE',  ( -15.75000000000000000, 13.79999999999999893, -3.200000000000001510 ) ) ;
#191411=CARTESIAN_POINT ( 'NONE',  ( 11.81911962874431055, 9.842894265158827594, 1.591749704452489533 ) ) ;
#191429=CARTESIAN_POINT ( 'NONE',  ( 11.89942855770813956, 11.29999999999999893, 0.6999999999999992895 ) ) ;
#191430=CARTESIAN_POINT ( 'NONE',  ( 11.80029657321907877, 6.865618457657816975, 1.950723814763024810 ) ) ;
#191437=CARTESIAN_POINT ( 'NONE',  ( -9.393996030428326094, 14.54120606779820513, -7.466831080202041449 ) ) ;
#191438=VECTOR ( 'NONE', #122407, 1000.000000000000000 ) ;
#191448=CARTESIAN_POINT ( 'NONE',  ( -10.95308175811721085, 9.799999999999982947, 1.799999999999999600 ) ) ;
#191471=CARTESIAN_POINT ( 'NONE',  ( 8.627580382214878441, 15.01093739429174079, -8.342115253638150207 ) ) ;
#191495=AXIS2_PLACEMENT_3D ( 'NONE', #40174, #73730, #24970 ) ;
#191508=CARTESIAN_POINT ( 'NONE',  ( 11.94105721237523277, 10.90000000000000036, 1.187919463087248273 ) ) ;
#191521=VERTEX_POINT ( 'NONE', #158863 ) ;
#191524=CARTESIAN_POINT ( 'NONE',  ( 10.18750394041541441, 13.31248422858857694, -7.180467324466926371 ) ) ;
#191525=CARTESIAN_POINT ( 'NONE',  ( -10.87092197480563271, 4.494752981060541330, 4.557748927716649412 ) ) ;
#191527=( BOUNDED_SURFACE ( )  B_SPLINE_SURFACE ( 3, 2, ( 
 ( #2292, #1233, #149652 ),
 ( #116139, #186396, #68369 ),
 ( #152849, #200505, #185330 ),
 ( #168029, #151792, #20687 ),
 ( #104103, #135541, #86778 ),
 ( #53212, #119343, #103033 ),
 ( #70494, #21739, #87848 ),
 ( #158, #182128, #99834 ),
 ( #7637, #203699, #191722 ),
 ( #156048, #71570, #187469 ),
 ( #157125, #55345, #27096 ),
 ( #189603, #121497, #39099 ) ),
 .UNSPECIFIED., .F., .F., .T. ) 
 B_SPLINE_SURFACE_WITH_KNOTS ( ( 4, 2, 2, 2, 2, 4 ),
 ( 3, 3 ),
 ( -1.951563910473907981E-18, 0.0007589766761258975305, 0.001517953352251797013, 0.001897441690314746916, 0.002276930028377696820, 0.003035906704503596194 ),
 ( 0.000000000000000000, 1.000000000000000000 ),
 .UNSPECIFIED. ) 
 GEOMETRIC_REPRESENTATION_ITEM ( )  RATIONAL_B_SPLINE_SURFACE ( (
 ( 1.000000000000000000, 0.8462407054814394813, 1.000000000000000000),
 ( 1.000000000000000000, 0.8467927744362970799, 1.000000000000000000),
 ( 1.000000000000000000, 0.8474042438982406500, 1.000000000000000000),
 ( 1.000000000000000000, 0.8486200509115283674, 1.000000000000000000),
 ( 1.000000000000000000, 0.8492421577839870395, 1.000000000000000000),
 ( 1.000000000000000000, 0.8499339144819614278, 1.000000000000000000),
 ( 1.000000000000000000, 0.8500877183792072689, 1.000000000000000000),
 ( 1.000000000000000000, 0.8503387282033902927, 1.000000000000000000),
 ( 1.000000000000000000, 0.8504341930334453625, 1.000000000000000000),
 ( 1.000000000000000000, 0.8507248712736660279, 1.000000000000000000),
 ( 1.000000000000000000, 0.8508901730824002252, 1.000000000000000000),
 ( 1.000000000000000000, 0.8509629433086481898, 1.000000000000000000) ) ) 
 REPRESENTATION_ITEM ( '' )  SURFACE ( )  );
#191554=CARTESIAN_POINT ( 'NONE',  ( -3.101842500994827390, 15.51993578035120791, -11.60075130251052755 ) ) ;
#191559=ORIENTED_EDGE ( 'NONE', *, *, #202741, .F. ) ;
#191566=DIRECTION ( 'NONE',  ( 1.000000000000000000, -0.000000000000000000, -0.000000000000000000 ) ) ;
#191572=EDGE_CURVE ( 'NONE', #59479, #209385, #163821, .T. ) ;
#191574=CARTESIAN_POINT ( 'NONE',  ( -11.06305611892948448, 12.34238460445608609, 0.9079708613958296093 ) ) ;
#191578=CARTESIAN_POINT ( 'NONE',  ( -11.84100621633422179, 11.11041574223335893, -1.444132586618106728 ) ) ;
#191579=CARTESIAN_POINT ( 'NONE',  ( 0.000000000000000000, 0.08000000000000020983, 11.18000000000000149 ) ) ;
#191585=SURFACE_STYLE_USAGE ( .BOTH. , #9646 ) ;
#191594=CARTESIAN_POINT ( 'NONE',  ( -9.907867159398911383, 3.530917919964545071, 6.788957344969876573 ) ) ;
#191605=( NAMED_UNIT ( * ) PLANE_ANGLE_UNIT ( ) SI_UNIT ( $, .RADIAN. ) );
#191649=AXIS2_PLACEMENT_3D ( 'NONE', #206409, #123146, #58033 ) ;
#191659=SURFACE_SIDE_STYLE ('',( #211111 ) ) ;
#191663=DIRECTION ( 'NONE',  ( 0.000000000000000000, 0.000000000000000000, 1.000000000000000000 ) ) ;
#191664=CARTESIAN_POINT ( 'NONE',  ( 1.734723475976807094E-15, 14.57308041853048231, 11.91973154060107376 ) ) ;
#191678=ORIENTED_EDGE ( 'NONE', *, *, #31143, .F. ) ;
#191689=ORIENTED_EDGE ( 'NONE', *, *, #168266, .F. ) ;
#191699=DIRECTION ( 'NONE',  ( -1.000000000000000000, -0.000000000000000000, 0.000000000000000000 ) ) ;
#191708=DIRECTION ( 'NONE',  ( 0.000000000000000000, -1.000000000000000000, 0.000000000000000000 ) ) ;
#191711=DIRECTION ( 'NONE',  ( 0.9632918427306580433, 0.000000000000000000, -0.2684563758389303945 ) ) ;
#191722=CARTESIAN_POINT ( 'NONE',  ( -10.11125148033187315, 3.596105362421267326, -6.463595993774343462 ) ) ;
#191765=B_SPLINE_CURVE_WITH_KNOTS ( 'NONE', 3,
 ( #29658, #178042, #61080, #14439, #159651, #131464, #197465, #163929, #31794, #94674, #145578, #46985, #196417, #65315, #49109, #95744, #180168, #143439, #79462, #179107, #27506, #161795, #28586, #93606, #213693, #13386, #48061, #112041 ),
 .UNSPECIFIED., .F., .F.,
 ( 4, 2, 2, 2, 2, 2, 2, 2, 2, 2, 2, 2, 2, 4 ),
 ( -5.999999999696835784E-08, 0.001605602215309425698, 0.002408433322964136092, 0.003211264430618846703, 0.004014095538273557313, 0.004816926645928267491, 0.005619757753582977668, 0.006422588861237687845, 0.008028251076547109066, 0.008831082184201819243, 0.009633913291856527686, 0.01043674439951123786, 0.01123957550716594804, 0.01284523772247536492 ),
 .UNSPECIFIED. ) ;
#191775=DIRECTION ( 'NONE',  ( 1.000000000000000000, -0.000000000000000000, -0.000000000000000000 ) ) ;
#191789=CARTESIAN_POINT ( 'NONE',  ( 10.62873463776380056, 13.79999999999999893, -3.200000000000001510 ) ) ;
#191804=CARTESIAN_POINT ( 'NONE',  ( -11.94105721237523454, 13.52740784401789220, 1.187919463087248273 ) ) ;
#191807=CARTESIAN_POINT ( 'NONE',  ( 9.680359324772703999, 13.43752487939449836, 8.167046318416048223 ) ) ;
#191814=DIRECTION ( 'NONE',  ( 0.1510067114093955887, -0.000000000000000000, 0.9885327375000383388 ) ) ;
#191821=EDGE_CURVE ( 'NONE', #15788, #177320, #74478, .T. ) ;
#191822=CARTESIAN_POINT ( 'NONE',  ( 11.96535697748089078, 12.34737332935543286, 0.9148528286453676550 ) ) ;
#191832=DIRECTION ( 'NONE',  ( 0.000000000000000000, -1.000000000000000000, -1.804652791718263484E-16 ) ) ;
#191839=CARTESIAN_POINT ( 'NONE',  ( 1.466069532605751007E-15, 14.48154074412737558, 12.00000000000000178 ) ) ;
#191856=CARTESIAN_POINT ( 'NONE',  ( 7.872797348053842015, 14.38630072364382784, 9.000752197161077106 ) ) ;
#191869=ADVANCED_FACE ( 'NONE', ( #177250 ), #181488, .F. ) ;
#191895=( NAMED_UNIT ( * ) PLANE_ANGLE_UNIT ( ) SI_UNIT ( $, .RADIAN. ) );
#191917=EDGE_CURVE ( 'NONE', #147946, #93554, #62889, .T. ) ;
#191927=UNCERTAINTY_MEASURE_WITH_UNIT (LENGTH_MEASURE( 1.000000000000000082E-05 ), #38477, 'distance_accuracy_value', 'NONE');
#191955=( GEOMETRIC_REPRESENTATION_CONTEXT ( 3 ) GLOBAL_UNCERTAINTY_ASSIGNED_CONTEXT ( ( #182641 ) ) GLOBAL_UNIT_ASSIGNED_CONTEXT ( ( #164668, #45606, #82336 ) ) REPRESENTATION_CONTEXT ( 'NONE', 'WORKASPACE' ) );
#191982=CARTESIAN_POINT ( 'NONE',  ( -11.86687934130374167, 9.990480503834417547, -1.056332641424308827 ) ) ;
#191994=DIRECTION ( 'NONE',  ( 0.000000000000000000, 1.000000000000000000, 0.000000000000000000 ) ) ;
#192009=EDGE_CURVE ( 'NONE', #124966, #8666, #60194, .T. ) ;
#192010=STYLED_ITEM ( 'NONE', ( #18857 ), #86694 ) ;
#192020=( GEOMETRIC_REPRESENTATION_CONTEXT ( 3 ) GLOBAL_UNCERTAINTY_ASSIGNED_CONTEXT ( ( #72597 ) ) GLOBAL_UNIT_ASSIGNED_CONTEXT ( ( #129868, #161223, #179605 ) ) REPRESENTATION_CONTEXT ( 'NONE', 'WORKASPACE' ) );
#192042=CARTESIAN_POINT ( 'NONE',  ( 11.84668730067608600, 10.90000000000000036, -1.400000000000001910 ) ) ;
#192056=( NAMED_UNIT ( * ) SI_UNIT ( $, .STERADIAN. ) SOLID_ANGLE_UNIT ( ) );
#192067=CARTESIAN_POINT ( 'NONE',  ( 8.916730223294068836, 12.80236288771289743, -7.560066957809561394 ) ) ;
#192075=ORIENTED_EDGE ( 'NONE', *, *, #168226, .F. ) ;
#192124=TRIMMED_CURVE ( 'NONE', #45076, ( PARAMETER_VALUE ( 3.141592653589793116 ), #94716 ), ( PARAMETER_VALUE ( 4.069539037113614199 ), #192169 ), .T., .PARAMETER. ) ;
#192129=CARTESIAN_POINT ( 'NONE',  ( -7.247736482492920018, 16.00000000000182254, 10.57961706324668150 ) ) ;
#192157=( NAMED_UNIT ( * ) PLANE_ANGLE_UNIT ( ) SI_UNIT ( $, .RADIAN. ) );
#192169=CARTESIAN_POINT ( 'NONE',  ( -9.604686356149278126, 3.999999999999997335, -7.193747284969076894 ) ) ;
#192176=CARTESIAN_POINT ( 'NONE',  ( 10.13617411650463396, 13.69189752474446742, 7.314094131634138130 ) ) ;
#192199=FILL_AREA_STYLE ('',( #109977 ) ) ;
#192209=CARTESIAN_POINT ( 'NONE',  ( -11.47199464713663453, 5.776720398841780124, 5.393175811422019628 ) ) ;
#192221=CYLINDRICAL_SURFACE ( 'NONE', #128820, 0.3999999999999997446 ) ;
#192233=CARTESIAN_POINT ( 'NONE',  ( 11.07015750233977691, 9.209416967217014971, 4.635152785948085885 ) ) ;
#192243=CARTESIAN_POINT ( 'NONE',  ( 0.000000000000000000, 0.000000000000000000, 0.000000000000000000 ) ) ;
#192278=( NAMED_UNIT ( * ) SI_UNIT ( $, .STERADIAN. ) SOLID_ANGLE_UNIT ( ) );
#192282=CARTESIAN_POINT ( 'NONE',  ( -11.26709733201210284, 6.404816583109345096, 4.000485531852068455 ) ) ;
#192322=CARTESIAN_POINT ( 'NONE',  ( -11.21412923722849619, 8.995494058042485364, 2.499828665724475485 ) ) ;
#192327=FILL_AREA_STYLE ('',( #140441 ) ) ;
#192342=CARTESIAN_POINT ( 'NONE',  ( -1.249999999999964695, 8.500000000000000000, 12.00100000000000122 ) ) ;
#192350=DIRECTION ( 'NONE',  ( 0.9632918427306580433, 0.000000000000000000, 0.2684563758389303945 ) ) ;
#192397=CARTESIAN_POINT ( 'NONE',  ( -9.409940793360268785, 3.999985931113709814, -6.919963696468023784 ) ) ;
#192419=EDGE_CURVE ( 'NONE', #7565, #123335, #195696, .T. ) ;
#192463=CARTESIAN_POINT ( 'NONE',  ( 0.02684197942426417779, 14.48154074394417812, 12.00000000000000178 ) ) ;
#192479=CARTESIAN_POINT ( 'NONE',  ( 11.91826849282518275, 10.19999999999998153, 1.399999999999998579 ) ) ;
#192505=CARTESIAN_POINT ( 'NONE',  ( -9.367496997601861608, 14.53091781611221833, -7.499999999994731326 ) ) ;
#192515=CARTESIAN_POINT ( 'NONE',  ( 8.731294531955244409, 14.92342541429118263, -8.233198443303315628 ) ) ;
#192525=CARTESIAN_POINT ( 'NONE',  ( 11.52483635780546045, 9.720000086424631647, 3.345866325258041840 ) ) ;
#192536=CARTESIAN_POINT ( 'NONE',  ( 8.674533818622323977, 14.86056906971758096, -8.228093639940686543 ) ) ;
#192583=CARTESIAN_POINT ( 'NONE',  ( 11.92619526913700057, 13.39999999999998259, 1.328859060402682868 ) ) ;
#192588=CARTESIAN_POINT ( 'NONE',  ( 9.809883170912574002, 12.88719579058855125, -8.001885615786651584 ) ) ;
#192592=AXIS2_PLACEMENT_3D ( 'NONE', #40798, #20235, #22361 ) ;
#192597=FILL_AREA_STYLE ('',( #161188 ) ) ;
#192600=ORIENTED_EDGE ( 'NONE', *, *, #47209, .F. ) ;
#192614=AXIS2_PLACEMENT_3D ( 'NONE', #77358, #112071, #70403 ) ;
#192622=CARTESIAN_POINT ( 'NONE',  ( -9.917242840447775265, 4.174869238508773783, -6.172972641688763140 ) ) ;
#192647=( LENGTH_UNIT ( ) NAMED_UNIT ( * ) SI_UNIT ( .MILLI., .METRE. ) );
#192652=CARTESIAN_POINT ( 'NONE',  ( 9.333041836227053523, 4.446947634372834912, 7.472413793103392265 ) ) ;
#192699=PLANE ( 'NONE',  #132935 ) ;
#192715=B_SPLINE_CURVE_WITH_KNOTS ( 'NONE', 3,
 ( #81922, #144846, #164248, #44116, #214020, #79789 ),
 .UNSPECIFIED., .F., .F.,
 ( 4, 2, 4 ),
 ( 0.000000000000000000, 0.0003844267940947831432, 0.0007688535881895662864 ),
 .UNSPECIFIED. ) ;
#192724=DIRECTION ( 'NONE',  ( 1.000000000000000000, -0.000000000000000000, -0.000000000000000000 ) ) ;
#192737=EDGE_LOOP ( 'NONE', ( #25288, #70552, #35851, #25038, #63163, #109084, #212701, #91975 ) ) ;
#192742=CARTESIAN_POINT ( 'NONE',  ( 0.000000000000000000, 13.88000000000000078, 0.000000000000000000 ) ) ;
#192762=COLOUR_RGB ( '', 0.08235294, 0.09019608, 0.10196078) ;
#192819=ADVANCED_FACE ( 'NONE', ( #193799 ), #40385, .T. ) ;
#192852=DIRECTION ( 'NONE',  ( -0.000000000000000000, 1.000000000000000000, -0.000000000000000000 ) ) ;
#192877=CARTESIAN_POINT ( 'NONE',  ( -11.35573736746270335, 9.987295855867214911, 3.554362808847973731 ) ) ;
#192892=ORIENTED_EDGE ( 'NONE', *, *, #189888, .F. ) ;
#192926=ORIENTED_EDGE ( 'NONE', *, *, #206146, .F. ) ;
#192943=CARTESIAN_POINT ( 'NONE',  ( -1.734723475976807094E-15, 3.481548657788671619, -12.00000000000000178 ) ) ;
#192969=( NAMED_UNIT ( * ) SI_UNIT ( $, .STERADIAN. ) SOLID_ANGLE_UNIT ( ) );
#193005=CARTESIAN_POINT ( 'NONE',  ( 11.92046840572485777, 9.947478752057280715, 1.382231356234940867 ) ) ;
#193006=ORIENTED_EDGE ( 'NONE', *, *, #9864, .F. ) ;
#193017=VECTOR ( 'NONE', #71678, 1000.000000000000000 ) ;
#193020=ORIENTED_EDGE ( 'NONE', *, *, #90081, .T. ) ;
#193034=AXIS2_PLACEMENT_3D ( 'NONE', #183086, #100767, #166849 ) ;
#193047=CARTESIAN_POINT ( 'NONE',  ( 11.55950211276791251, 11.29999999999998295, 3.221476510067111665 ) ) ;
#193059=CARTESIAN_POINT ( 'NONE',  ( 11.41381675112459959, 10.90000000000001101, -3.704697986577260682 ) ) ;
#193060=CARTESIAN_POINT ( 'NONE',  ( -9.604686356149278126, 4.518467169708413778, -7.193747284969076006 ) ) ;
#193073=DIRECTION ( 'NONE',  ( 0.000000000000000000, -1.000000000000000000, 0.000000000000000000 ) ) ;
#193079=EDGE_CURVE ( 'NONE', #158402, #102449, #11080, .T. ) ;
#193080=CARTESIAN_POINT ( 'NONE',  ( -15.75000000000000000, 13.39999999999998259, 1.399999999999998579 ) ) ;
#193087=EDGE_CURVE ( 'NONE', #80159, #195702, #123881, .T. ) ;
#193089=SURFACE_SIDE_STYLE ('',( #81484 ) ) ;
#193107=B_SPLINE_CURVE_WITH_KNOTS ( 'NONE', 3,
 ( #184922, #88527, #102632, #120015, #52804, #203300 ),
 .UNSPECIFIED., .F., .F.,
 ( 4, 2, 4 ),
 ( 0.000000000000000000, 0.0003157158648874031190, 0.0006314317297748062380 ),
 .UNSPECIFIED. ) ;
#193117=COLOUR_RGB ( '', 0.40784314, 0.44705882, 0.49803922) ;
#193134=CARTESIAN_POINT ( 'NONE',  ( 11.88048553210577296, 7.839794170119552597, 1.743655026309894218 ) ) ;
#193153=CARTESIAN_POINT ( 'NONE',  ( 12.19510520210794979, 6.199134917050342253, -2.169279492894659711 ) ) ;
#193213=CARTESIAN_POINT ( 'NONE',  ( 0.3554123170483391991, 14.00000000000058265, 12.67999999502907649 ) ) ;
#193219=CARTESIAN_POINT ( 'NONE',  ( -1.333449616921166703, 8.249651149236390424, 11.01993490927447539 ) ) ;
#193225=CARTESIAN_POINT ( 'NONE',  ( 11.04536101718726293, 10.09418840193640499, -1.100000000000000311 ) ) ;
#193242=( LENGTH_UNIT ( ) NAMED_UNIT ( * ) SI_UNIT ( .MILLI., .METRE. ) );
#193256=LINE ( 'NONE', #208422, #162633 ) ;
#193259=CARTESIAN_POINT ( 'NONE',  ( 7.922173639401519196, 13.65794249303706920, 8.699232811755850392 ) ) ;
#193282=CARTESIAN_POINT ( 'NONE',  ( -9.541824394042135893, 5.027248526908232762, 6.730710380108894775 ) ) ;
#193283=SURFACE_STYLE_USAGE ( .BOTH. , #108906 ) ;
#193294=CARTESIAN_POINT ( 'NONE',  ( -11.69380381030441107, 8.410673437356566140, -1.083569014401829955 ) ) ;
#193305=DIRECTION ( 'NONE',  ( 1.000000000000000000, -0.000000000000000000, -0.000000000000000000 ) ) ;
#193310=CARTESIAN_POINT ( 'NONE',  ( -9.586287156527431463, 14.76664842859987914, 7.218579095329854312 ) ) ;
#193317=CARTESIAN_POINT ( 'NONE',  ( 11.87989628165243161, 7.840779707844498958, 1.747908902009029708 ) ) ;
#193355=EDGE_CURVE ( 'NONE', #46648, #122534, #101638, .T. ) ;
#193368=CARTESIAN_POINT ( 'NONE',  ( -11.32640490158465774, 6.353037010736665380, 3.968039318877488952 ) ) ;
#193376=AXIS2_PLACEMENT_3D ( 'NONE', #202295, #120085, #186060 ) ;
#193377=CARTESIAN_POINT ( 'NONE',  ( -11.77314774087514238, 8.651273335165431178, 2.095004279193475760 ) ) ;
#193391=VERTEX_POINT ( 'NONE', #68354 ) ;
#193409=CARTESIAN_POINT ( 'NONE',  ( -11.87988507903381219, 5.100570458969788668, 4.764376171217361566 ) ) ;
#193418=EDGE_LOOP ( 'NONE', ( #37912, #499, #75816, #4909 ) ) ;
#193425=VERTEX_POINT ( 'NONE', #53198 ) ;
#193430=FACE_OUTER_BOUND ( 'NONE', #172272, .T. ) ;
#193462=VERTEX_POINT ( 'NONE', #152835 ) ;
#193468=DIRECTION ( 'NONE',  ( -0.9885327375000381167, 0.000000000000000000, -0.1510067114093955609 ) ) ;
#193478=CARTESIAN_POINT ( 'NONE',  ( 0.008622056077349157799, 14.55305231409391808, 11.95585894185517084 ) ) ;
#193483=DIRECTION ( 'NONE',  ( 1.224646797963766027E-16, -4.396526966619892032E-05, 0.9999999990335275424 ) ) ;
#193484=( BOUNDED_SURFACE ( )  B_SPLINE_SURFACE ( 3, 2, ( 
 ( #163302, #164364, #82032 ),
 ( #63663, #214126, #197910 ),
 ( #49538, #144952, #115664 ),
 ( #181658, #33284, #165421 ),
 ( #195799, #193655, #14883 ),
 ( #46360, #17017, #62585 ),
 ( #111417, #210958, #128747 ),
 ( #129817, #169690, #116729 ),
 ( #68963, #1828, #151323 ),
 ( #19161, #150260, #53818 ),
 ( #52737, #152380, #749 ),
 ( #3959, #183803, #185923 ),
 ( #87384, #119948, #70027 ),
 ( #136142, #67887, #37558 ),
 ( #137217, #182729, #100421 ),
 ( #85235, #201096, #167561 ),
 ( #103638, #202160, #21278 ),
 ( #135083, #54882, #5025 ),
 ( #153452, #166492, #168621 ),
 ( #118871, #88461, #121036 ),
 ( #50604, #102561, #184857 ),
 ( #71099, #51691, #187003 ),
 ( #203238, #84171, #38634 ),
 ( #104711, #36484, #170760 ),
 ( #22349, #117813, #2891 ),
 ( #66815, #132958, #86309 ),
 ( #198961, #134032, #101491 ),
 ( #35413, #34348, #18083 ),
 ( #200039, #20223, #75403 ),
 ( #89536, #191260, #55950 ),
 ( #122103, #39697, #139350 ),
 ( #23425, #188067, #205380 ) ),
 .UNSPECIFIED., .F., .F., .F. ) 
 B_SPLINE_SURFACE_WITH_KNOTS ( ( 4, 2, 2, 2, 2, 2, 2, 2, 2, 2, 2, 2, 2, 2, 2, 4 ),
 ( 3, 3 ),
 ( 0.000000000000000000, 0.001493720594899021785, 0.002987441189798043569, 0.005974882379596087138, 0.007468602974495109140, 0.008962323569394130274, 0.009709183866843641708, 0.01045604416429315314, 0.01194976475919217428, 0.01344348535409119541, 0.01493720594899021828, 0.01643092654388923768, 0.01792464713878826055, 0.02091208832858630629, 0.02240580892348532915, 0.02389952951838434855 ),
 ( 0.000000000000000000, 1.000000000000000000 ),
 .UNSPECIFIED. ) 
 GEOMETRIC_REPRESENTATION_ITEM ( )  RATIONAL_B_SPLINE_SURFACE ( (
 ( 1.000000000000000000, 0.8434733505592640901, 1.000000000000000000),
 ( 1.000000000000000000, 0.8431702246155254876, 1.000000000000000000),
 ( 1.000000000000000000, 0.8426367324223418276, 1.000000000000000000),
 ( 1.000000000000000000, 0.8408650922403015926, 1.000000000000000000),
 ( 1.000000000000000000, 0.8396428711856337435, 1.000000000000000000),
 ( 1.000000000000000000, 0.8353280728740983818, 1.000000000000000000),
 ( 1.000000000000000000, 0.8320647679512711559, 1.000000000000000000),
 ( 1.000000000000000000, 0.8235806410807833267, 1.000000000000000000),
 ( 1.000000000000000000, 0.8255774334008273430, 1.000000000000000000),
 ( 1.000000000000000000, 0.8281857448045425452, 1.000000000000000000),
 ( 1.000000000000000000, 0.8295473863155264915, 1.000000000000000000),
 ( 1.000000000000000000, 0.8309453578789692818, 1.000000000000000000),
 ( 1.000000000000000000, 0.8312210268024100568, 1.000000000000000000),
 ( 1.000000000000000000, 0.8317131830652759739, 1.000000000000000000),
 ( 1.000000000000000000, 0.8319338935246425315, 1.000000000000000000),
 ( 1.000000000000000000, 0.8326804068065388753, 1.000000000000000000),
 ( 1.000000000000000000, 0.8334031718083524387, 1.000000000000000000),
 ( 1.000000000000000000, 0.8334179402980076423, 1.000000000000000000),
 ( 1.000000000000000000, 0.8328045324390893622, 1.000000000000000000),
 ( 1.000000000000000000, 0.8317996902536097803, 1.000000000000000000),
 ( 1.000000000000000000, 0.8314091991306797880, 1.000000000000000000),
 ( 1.000000000000000000, 0.8295445083194166180, 1.000000000000000000),
 ( 1.000000000000000000, 0.8285669895138008112, 1.000000000000000000),
 ( 1.000000000000000000, 0.8259632866995387790, 1.000000000000000000),
 ( 1.000000000000000000, 0.8235472590115482383, 1.000000000000000000),
 ( 1.000000000000000000, 0.8321649622163090898, 1.000000000000000000),
 ( 1.000000000000000000, 0.8357012932624516832, 1.000000000000000000),
 ( 1.000000000000000000, 0.8399852490580022035, 1.000000000000000000),
 ( 1.000000000000000000, 0.8411359117240285732, 1.000000000000000000),
 ( 1.000000000000000000, 0.8427639893650330505, 1.000000000000000000),
 ( 1.000000000000000000, 0.8432301679486819967, 1.000000000000000000),
 ( 1.000000000000000000, 0.8435419936913640671, 1.000000000000000000) ) ) 
 REPRESENTATION_ITEM ( '' )  SURFACE ( )  );
#193499=EDGE_CURVE ( 'NONE', #25291, #94694, #20674, .T. ) ;
#193556=PRESENTATION_STYLE_ASSIGNMENT (( #161064 ) ) ;
#193561=CARTESIAN_POINT ( 'NONE',  ( 11.92619526913699701, 10.19999999999998153, 1.328859060402682868 ) ) ;
#193578=CARTESIAN_POINT ( 'NONE',  ( 11.95123034216491398, 6.644963984119064193, -0.4921840132778478871 ) ) ;
#193584=CARTESIAN_POINT ( 'NONE',  ( -9.386399777248481513, 14.48154088884566804, -7.476390435783241806 ) ) ;
#193605=CARTESIAN_POINT ( 'NONE',  ( 11.44800751629993130, 9.799999999999982947, 3.302956944461088451 ) ) ;
#193616=CARTESIAN_POINT ( 'NONE',  ( 9.428250952287722697, 13.54490846161957762, -7.423481931054033645 ) ) ;
#193655=CARTESIAN_POINT ( 'NONE',  ( 9.476699878348894046, 11.04296043381019743, -7.367623491263915803 ) ) ;
#193659=CARTESIAN_POINT ( 'NONE',  ( 11.92050416151433012, 13.65205375279633238, 1.381922468431395767 ) ) ;
#193664=CARTESIAN_POINT ( 'NONE',  ( 10.40290000253160940, 12.22595686778796065, -6.657689775135003707 ) ) ;
#193677=CIRCLE ( 'NONE', #31068, 11.09999999999999964 ) ;
#193707=CARTESIAN_POINT ( 'NONE',  ( -9.608183788959879124, 14.88164563814821939, -7.189075342400532698 ) ) ;
#193716=CARTESIAN_POINT ( 'NONE',  ( -15.75000000000000000, 13.40000000000000036, 1.099999999999996758 ) ) ;
#193721=DIRECTION ( 'NONE',  ( -0.000000000000000000, 0.000000000000000000, -1.000000000000000000 ) ) ;
#193728=CARTESIAN_POINT ( 'NONE',  ( 9.601861702642535690, 3.883749503993501051, 7.121442011178659826 ) ) ;
#193733=CARTESIAN_POINT ( 'NONE',  ( -15.75000000000000000, 11.29999999999999893, 0.6999999999999992895 ) ) ;
#193736=CARTESIAN_POINT ( 'NONE',  ( -9.569358774149645086, 3.553052365627043852, 7.167287524840456392 ) ) ;
#193761=B_SPLINE_CURVE_WITH_KNOTS ( 'NONE', 3,
 ( #84908, #201831, #3626, #67561, #135807, #133704 ),
 .UNSPECIFIED., .F., .F.,
 ( 4, 2, 4 ),
 ( 0.000000000000000000, 0.0003168911866439334617, 0.0006337823732878669234 ),
 .UNSPECIFIED. ) ;
#193766=CARTESIAN_POINT ( 'NONE',  ( 11.89942855770814312, 13.88000000000000078, 0.6999999999999992895 ) ) ;
#193776=FILL_AREA_STYLE ('',( #97373 ) ) ;
#193778=PLANE ( 'NONE',  #49322 ) ;
#193779=DIRECTION ( 'NONE',  ( -8.881784197001252323E-15, 0.000000000000000000, 1.000000000000000000 ) ) ;
#193799=FACE_OUTER_BOUND ( 'NONE', #12139, .T. ) ;
#193826=CARTESIAN_POINT ( 'NONE',  ( 0.000000000000000000, 11.29999999999999893, 0.000000000000000000 ) ) ;
#193870=CARTESIAN_POINT ( 'NONE',  ( -11.92619526913700057, 19.00000000000000000, 1.328859060402684644 ) ) ;
#193872=ORIENTED_EDGE ( 'NONE', *, *, #187404, .F. ) ;
#193898=DIRECTION ( 'NONE',  ( 0.000000000000000000, 1.000000000000000000, 0.000000000000000000 ) ) ;
#193907=EDGE_CURVE ( 'NONE', #30509, #121309, #58529, .T. ) ;
#193910=EDGE_CURVE ( 'NONE', #90767, #171829, #6555, .T. ) ;
#193929=DIRECTION ( 'NONE',  ( -0.000000000000000000, -1.000000000000000000, -0.000000000000000000 ) ) ;
#193931=DIRECTION ( 'NONE',  ( -0.7806247497998005658, 0.000000000000000000, -0.6249999999999988898 ) ) ;
#193934=DIRECTION ( 'NONE',  ( 0.000000000000000000, 0.000000000000000000, 1.000000000000000000 ) ) ;
#193980=LINE ( 'NONE', #213413, #13207 ) ;
#194024=CARTESIAN_POINT ( 'NONE',  ( 11.91826849282518275, 10.89999999999999858, -1.400000000000001465 ) ) ;
#194027=CARTESIAN_POINT ( 'NONE',  ( -11.95359438122011042, 13.60421899708702753, -1.059536798430454008 ) ) ;
#194044=EDGE_CURVE ( 'NONE', #127188, #62746, #23878, .T. ) ;
#194061=DIRECTION ( 'NONE',  ( -0.000000000000000000, -1.000000000000000000, -0.000000000000000000 ) ) ;
#194085=ORIENTED_EDGE ( 'NONE', *, *, #94666, .F. ) ;
#194120=CARTESIAN_POINT ( 'NONE',  ( 11.52469724861194678, 11.37999993351184891, 3.346365485506860526 ) ) ;
#194135=CARTESIAN_POINT ( 'NONE',  ( -11.44791656467458552, 13.79999999999999716, -3.303228920649581291 ) ) ;
#194143=CARTESIAN_POINT ( 'NONE',  ( 1.499999999999959588, 7.000000000000000000, -10.89724735885168805 ) ) ;
#194148=( LENGTH_UNIT ( ) NAMED_UNIT ( * ) SI_UNIT ( .MILLI., .METRE. ) );
#194163=EDGE_LOOP ( 'NONE', ( #13115, #97540, #165897, #168093 ) ) ;
#194171=PRODUCT_DEFINITION_SHAPE ( 'NONE', 'NONE',  #189422 ) ;
#194185=B_SPLINE_CURVE_WITH_KNOTS ( 'NONE', 3,
 ( #199236, #201366, #150532, #99633, #117006, #35686, #183005, #151595, #181930, #67096, #18366, #118080, #33561, #133232, #84443, #36749 ),
 .UNSPECIFIED., .F., .F.,
 ( 4, 2, 2, 2, 2, 2, 2, 4 ),
 ( 0.000000000000000000, 0.0005357556996629550235, 0.001071511399325910047, 0.001607267098988864962, 0.002143022798651820094, 0.003214534197977728189, 0.003750289897640680069, 0.004286045597303632382 ),
 .UNSPECIFIED. ) ;
#194194=CARTESIAN_POINT ( 'NONE',  ( -11.48788097203293823, 12.26956945602307947, 3.469500700354829714 ) ) ;
#194204=( GEOMETRIC_REPRESENTATION_CONTEXT ( 3 ) GLOBAL_UNCERTAINTY_ASSIGNED_CONTEXT ( ( #202332 ) ) GLOBAL_UNIT_ASSIGNED_CONTEXT ( ( #130101, #197137, #50896 ) ) REPRESENTATION_CONTEXT ( 'NONE', 'WORKASPACE' ) );
#194210=SURFACE_STYLE_USAGE ( .BOTH. , #165980 ) ;
#194221=CARTESIAN_POINT ( 'NONE',  ( 9.372627106707136946, 12.67835162939719318, 8.896217961834167909 ) ) ;
#194236=CARTESIAN_POINT ( 'NONE',  ( -9.333041836230020039, 14.55305236562984383, 7.472413793098202639 ) ) ;
#194238=LINE ( 'NONE', #210479, #75372 ) ;
#194242=AXIS2_PLACEMENT_3D ( 'NONE', #105549, #135900, #124000 ) ;
#194251=CARTESIAN_POINT ( 'NONE',  ( -11.86685672517501899, 11.10918917859810584, -1.056525322636018727 ) ) ;
#194264=DIRECTION ( 'NONE',  ( -1.000000000000000000, -6.873509095275351032E-09, 4.111253358064373089E-11 ) ) ;
#194279=CARTESIAN_POINT ( 'NONE',  ( -1.724555757183727112, 15.99999999999692335, 11.68000002332616205 ) ) ;
#194280=DIRECTION ( 'NONE',  ( 0.000000000000000000, 0.000000000000000000, 1.000000000000000000 ) ) ;
#194285=CARTESIAN_POINT ( 'NONE',  ( -11.41381675112453387, 13.39999999999998259, 3.704697986577180746 ) ) ;
#194321=DIRECTION ( 'NONE',  ( 0.000000000000000000, -1.445602896647338917E-16, 1.000000000000000000 ) ) ;
#194325=CARTESIAN_POINT ( 'NONE',  ( 8.655013507854587118, 13.90139471787301240, -7.850520059195646105 ) ) ;
#194328=CARTESIAN_POINT ( 'NONE',  ( 9.196684282068718019, 13.24788661686111091, 9.037284322956145033 ) ) ;
#194342=AXIS2_PLACEMENT_3D ( 'NONE', #182304, #33931, #66401 ) ;
#194350=EDGE_LOOP ( 'NONE', ( #152135, #84711, #49068, #79673 ) ) ;
#194360=CARTESIAN_POINT ( 'NONE',  ( -11.91006458477769314, 5.204012295529565790, -4.700227299318338936 ) ) ;
#194372=DIRECTION ( 'NONE',  ( 0.000000000000000000, 0.000000000000000000, -1.000000000000000000 ) ) ;
#194378=CARTESIAN_POINT ( 'NONE',  ( -9.438511317130744871, 15.32520388209415785, 7.309645043510521134 ) ) ;
#194385=CARTESIAN_POINT ( 'NONE',  ( 11.75595146754954357, 7.889406149263008317, 2.187765205025514970 ) ) ;
#194398=VECTOR ( 'NONE', #31701, 1000.000000000000000 ) ;
#194435=CARTESIAN_POINT ( 'NONE',  ( -11.99966308016123229, 8.078345815552603781, 0.5440065656137862415 ) ) ;
#194443=CARTESIAN_POINT ( 'NONE',  ( -11.95038703364911470, 8.982067687420316915, -1.244795252127886664 ) ) ;
#194446=LINE ( 'NONE', #195523, #64390 ) ;
#194449=ORIENTED_EDGE ( 'NONE', *, *, #177319, .T. ) ;
#194465=CARTESIAN_POINT ( 'NONE',  ( -11.97181042169641962, 12.22000000000000597, -0.8318531151397202672 ) ) ;
#194474=CARTESIAN_POINT ( 'NONE',  ( -11.31903982423144051, 5.215113036472975416, 5.710294617915439019 ) ) ;
#194493=CARTESIAN_POINT ( 'NONE',  ( -10.97030319645364749, 12.29999999999998295, 1.695206765504801094 ) ) ;
#194501=DIRECTION ( 'NONE',  ( 1.000000000000000000, 0.000000000000000000, -3.706092522800016599E-15 ) ) ;
#194511=CARTESIAN_POINT ( 'NONE',  ( 9.622290429756469976, 3.756446959784764061, 7.170831222936541849 ) ) ;
#194525=DIRECTION ( 'NONE',  ( -0.000000000000000000, -1.000000000000000000, -0.000000000000000000 ) ) ;
#194535=CARTESIAN_POINT ( 'NONE',  ( 1.999999999994443289E-05, 14.55305236562340809, 11.95586206896494197 ) ) ;
#194545=STYLED_ITEM ( 'NONE', ( #137734 ), #50792 ) ;
#194550=FILL_AREA_STYLE ('',( #129648 ) ) ;
#194571=EDGE_CURVE ( 'NONE', #54861, #115034, #146881, .T. ) ;
#194584=CARTESIAN_POINT ( 'NONE',  ( -1.249999999999964695, 8.500000000000000000, -11.02939254900287303 ) ) ;
#194614=AXIS2_PLACEMENT_3D ( 'NONE', #173383, #41252, #88932 ) ;
#194640=SURFACE_STYLE_FILL_AREA ( #62508 ) ;
#194645=CARTESIAN_POINT ( 'NONE',  ( -9.993490455110626058, 4.532987658119245644, 6.649910637754151921 ) ) ;
#194667=CARTESIAN_POINT ( 'NONE',  ( 11.55950211276791428, 9.719999999999982876, 3.221476510067112109 ) ) ;
#194678=CARTESIAN_POINT ( 'NONE',  ( 6.928203230275523872, 15.51845925587262620, -9.797958971132697314 ) ) ;
#194701=EDGE_CURVE ( 'NONE', #144017, #76712, #177227, .T. ) ;
#194707=CARTESIAN_POINT ( 'NONE',  ( -9.541882734523161602, 5.027466607964795386, -6.730450668810338044 ) ) ;
#194715=CARTESIAN_POINT ( 'NONE',  ( -11.94105721237523099, 13.40000000000000036, -1.187919463087249827 ) ) ;
#194721=DIRECTION ( 'NONE',  ( 1.000000000000000000, -0.000000000000000000, -0.000000000000000000 ) ) ;
#194730=CARTESIAN_POINT ( 'NONE',  ( 9.741349722503858999, 13.15934765701661391, 8.090281636115273400 ) ) ;
#194757=SURFACE_STYLE_FILL_AREA ( #197947 ) ;
#194759=CARTESIAN_POINT ( 'NONE',  ( 9.406473873361589355, 3.553052728507827052, -7.380697183404369532 ) ) ;
#194775=FILL_AREA_STYLE_COLOUR ( '', #18996 ) ;
#194838=CARTESIAN_POINT ( 'NONE',  ( -11.86145016429273014, 12.69999999999999929, -1.180000000000002158 ) ) ;
#194846=EDGE_LOOP ( 'NONE', ( #148025, #166384, #76619, #198512, #196779, #101579, #4380, #155007 ) ) ;
#194848=FACE_OUTER_BOUND ( 'NONE', #79057, .T. ) ;
#194849=STYLED_ITEM ( 'NONE', ( #112401 ), #55200 ) ;
#194864=ORIENTED_EDGE ( 'NONE', *, *, #9705, .T. ) ;
#194875=( NAMED_UNIT ( * ) PLANE_ANGLE_UNIT ( ) SI_UNIT ( $, .RADIAN. ) );
#194882=DIRECTION ( 'NONE',  ( 0.000000000000000000, 0.000000000000000000, -1.000000000000000000 ) ) ;
#194903=ORIENTED_EDGE ( 'NONE', *, *, #209369, .F. ) ;
#194912=TOROIDAL_SURFACE ( 'NONE', #56544, 11.92000000000000171, 0.08000000000000000167 ) ;
#194914=AXIS2_PLACEMENT_3D ( 'NONE', #141045, #139962, #75998 ) ;
#194931=CIRCLE ( 'NONE', #101535, 0.08000000000000014044 ) ;
#194969=CARTESIAN_POINT ( 'NONE',  ( 11.33772463945036790, 12.69999999999999929, -3.600000000000000977 ) ) ;
#194987=( NAMED_UNIT ( * ) SI_UNIT ( $, .STERADIAN. ) SOLID_ANGLE_UNIT ( ) );
#194989=CARTESIAN_POINT ( 'NONE',  ( -11.04986239659823433, 11.10939231485699175, -1.056426191432995765 ) ) ;
#195002=( NAMED_UNIT ( * ) SI_UNIT ( $, .STERADIAN. ) SOLID_ANGLE_UNIT ( ) );
#195013=VERTEX_POINT ( 'NONE', #169485 ) ;
#195033=CARTESIAN_POINT ( 'NONE',  ( -11.89942855770813956, 12.22000000000000064, 0.6999999999999992895 ) ) ;
#195042=ORIENTED_EDGE ( 'NONE', *, *, #35345, .T. ) ;
#195085=B_SPLINE_CURVE_WITH_KNOTS ( 'NONE', 3,
 ( #9936, #110713, #124843, #45666, #26183, #176713 ),
 .UNSPECIFIED., .F., .F.,
 ( 4, 2, 4 ),
 ( 0.000000000000000000, 0.0003767011250903909100, 0.0007534022501807818200 ),
 .UNSPECIFIED. ) ;
#195108=CARTESIAN_POINT ( 'NONE',  ( -11.97297122925952095, 13.79874920673088567, -0.8121202983519171248 ) ) ;
#195119=EDGE_CURVE ( 'NONE', #103981, #167139, #64421, .T. ) ;
#195126=CARTESIAN_POINT ( 'NONE',  ( 11.86239285000045740, 13.87999999999998302, 1.812080536912751061 ) ) ;
#195186=ORIENTED_EDGE ( 'NONE', *, *, #7050, .T. ) ;
#195212=CARTESIAN_POINT ( 'NONE',  ( 11.48243876534946217, 11.29999999999999893, -3.200000000000001510 ) ) ;
#195268=CARTESIAN_POINT ( 'NONE',  ( 0.000000000000000000, 19.00000000000000000, 0.000000000000000000 ) ) ;
#195279=ADVANCED_FACE ( 'NONE', ( #109903 ), #23212, .T. ) ;
#195285=EDGE_CURVE ( 'NONE', #198869, #145411, #39486, .T. ) ;
#195302=CARTESIAN_POINT ( 'NONE',  ( 8.639639562656480365, 12.08920847220495887, 8.327081629787771888 ) ) ;
#195311=CARTESIAN_POINT ( 'NONE',  ( 10.95308175811721085, 9.799999999999982947, 1.799999999999999600 ) ) ;
#195324=DIRECTION ( 'NONE',  ( -8.881784197001252323E-16, 0.000000000000000000, 1.000000000000000000 ) ) ;
#195328=EDGE_CURVE ( 'NONE', #8666, #175384, #175915, .T. ) ;
#195356=CARTESIAN_POINT ( 'NONE',  ( -11.33772463945037146, 13.50911576511424173, 3.599999999999998757 ) ) ;
#195357=DIRECTION ( 'NONE',  ( -0.000000000000000000, -1.000000000000000000, -0.000000000000000000 ) ) ;
#195372=VERTEX_POINT ( 'NONE', #139136 ) ;
#195385=CYLINDRICAL_SURFACE ( 'NONE', #26583, 0.07999999999999998779 ) ;
#195387=CIRCLE ( 'NONE', #160748, 12.00000000000000178 ) ;
#195389=EDGE_CURVE ( 'NONE', #85120, #131174, #85125, .T. ) ;
#195398=EDGE_CURVE ( 'NONE', #125687, #158402, #191765, .T. ) ;
#195400=DIRECTION ( 'NONE',  ( -0.000000000000000000, 1.000000000000000000, 1.804652791718263484E-16 ) ) ;
#195404=CARTESIAN_POINT ( 'NONE',  ( 8.233435442164850571, 14.52223435847226618, -8.288968424944320290 ) ) ;
#195407=CARTESIAN_POINT ( 'NONE',  ( 8.327294770833812976, 13.18750184243608103, 8.540276611412847885 ) ) ;
#195439=CARTESIAN_POINT ( 'NONE',  ( -11.97594889418004804, 7.449136658168690417, 0.9368335759953716479 ) ) ;
#195445=COLOUR_RGB ( '', 0.40784314, 0.44705882, 0.49803922) ;
#195465=CARTESIAN_POINT ( 'NONE',  ( 11.99424499309541758, 7.649948518832609956, -0.4322994337658502828 ) ) ;
#195511=CARTESIAN_POINT ( 'NONE',  ( -11.82472405718483266, 7.630400978341936202, 2.057497206828635239 ) ) ;
#195520=CARTESIAN_POINT ( 'NONE',  ( -10.64335489816787650, 5.927586918088680434, -5.550313554347075851 ) ) ;
#195523=CARTESIAN_POINT ( 'NONE',  ( -10.50000000000000000, 0.000000000000000000, -3.600000000000002309 ) ) ;
#195532=EDGE_LOOP ( 'NONE', ( #39695, #60383, #86313, #175542 ) ) ;
#195536=STYLED_ITEM ( 'NONE', ( #204916 ), #120967 ) ;
#195542=STYLED_ITEM ( 'NONE', ( #29935 ), #191869 ) ;
#195552=CARTESIAN_POINT ( 'NONE',  ( -11.76696981052429614, 4.673730779118272061, -4.995440715239800156 ) ) ;
#195571=( NAMED_UNIT ( * ) SI_UNIT ( $, .STERADIAN. ) SOLID_ANGLE_UNIT ( ) );
#195582=CARTESIAN_POINT ( 'NONE',  ( -8.752797858673307729, 15.44734748039404515, 8.156385747514464768 ) ) ;
#195593=CARTESIAN_POINT ( 'NONE',  ( 9.518950567327420842, 3.582805947357989851, 7.307358422849582702 ) ) ;
#195600=EDGE_CURVE ( 'NONE', #66223, #170318, #65156, .T. ) ;
#195625=CARTESIAN_POINT ( 'NONE',  ( -10.30104275384242740, 4.689840931292195592, -5.506867539468097483 ) ) ;
#195633=CARTESIAN_POINT ( 'NONE',  ( -15.75000000000000000, 10.90000000000000036, -1.400000000000001910 ) ) ;
#195646=ORIENTED_EDGE ( 'NONE', *, *, #138353, .F. ) ;
#195648=EDGE_CURVE ( 'NONE', #139393, #60282, #209727, .T. ) ;
#195689=CARTESIAN_POINT ( 'NONE',  ( 10.98549472050129694, 9.842702027212720139, -1.592011381755358723 ) ) ;
#195696=CIRCLE ( 'NONE', #140371, 0.5000000000000013323 ) ;
#195702=VERTEX_POINT ( 'NONE', #185477 ) ;
#195720=CARTESIAN_POINT ( 'NONE',  ( 11.96533679318059917, 11.25246011187004491, 0.9151144679398781623 ) ) ;
#195721=CARTESIAN_POINT ( 'NONE',  ( 8.917589090474498548, 12.70555303101720135, -7.960785596413196608 ) ) ;
#195724=CARTESIAN_POINT ( 'NONE',  ( -9.985564813494324454, 4.581166929158016821, 6.661451624069083977 ) ) ;
#195758=CARTESIAN_POINT ( 'NONE',  ( -15.75000000000000000, 12.69999999999999929, -1.400000000000001910 ) ) ;
#195777=ADVANCED_FACE ( 'NONE', ( #32845 ), #12598, .T. ) ;
#195779=EDGE_CURVE ( 'NONE', #138623, #95365, #75542, .T. ) ;
#195784=CARTESIAN_POINT ( 'NONE',  ( 9.367496997597598352, 3.481540744127370690, 7.500000000000000000 ) ) ;
#195799=CARTESIAN_POINT ( 'NONE',  ( 9.450148846975686467, 11.05536808409302907, -7.324943998173960580 ) ) ;
#195807=FILL_AREA_STYLE_COLOUR ( '', #92315 ) ;
#195808=CARTESIAN_POINT ( 'NONE',  ( 10.16623870845280742, 13.45394180708211351, -7.231736421947215554 ) ) ;
#195824=CARTESIAN_POINT ( 'NONE',  ( 9.508009452425755015, 4.000007913748543587, -7.612499999891275237 ) ) ;
#195827=AXIS2_PLACEMENT_3D ( 'NONE', #100256, #117643, #184689 ) ;
#195833=CARTESIAN_POINT ( 'NONE',  ( -11.92045683181315674, 11.15275927879484641, -1.382340670101859237 ) ) ;
#195839=CARTESIAN_POINT ( 'NONE',  ( -9.409940793360268785, 3.999985931113709814, -6.919963696468023784 ) ) ;
#195844=VERTEX_POINT ( 'NONE', #199589 ) ;
#195852=CARTESIAN_POINT ( 'NONE',  ( -9.404204974767472081, 15.50982908332066401, -7.453969465644266990 ) ) ;
#195866=AXIS2_PLACEMENT_3D ( 'NONE', #167830, #163582, #53007 ) ;
#195885=EDGE_LOOP ( 'NONE', ( #73873, #54084, #145461, #24461 ) ) ;
#195893=EDGE_CURVE ( 'NONE', #209617, #140333, #85860, .T. ) ;
#195957=FACE_OUTER_BOUND ( 'NONE', #7860, .T. ) ;
#196023=DIRECTION ( 'NONE',  ( 1.000000000000000000, -0.000000000000000000, -0.000000000000000000 ) ) ;
#196030=TOROIDAL_SURFACE ( 'NONE', #120020, 11.92000000000000171, 0.08000000000000000167 ) ;
#196052=CARTESIAN_POINT ( 'NONE',  ( 0.008622056077349157799, 14.55305231409391808, 11.95585894185517084 ) ) ;
#196062=MECHANICAL_DESIGN_GEOMETRIC_PRESENTATION_REPRESENTATION('',(#109697),#78534);
#196082=DIRECTION ( 'NONE',  ( 1.224643483124940471E-16, 0.002327115863039739760, 0.9999972922622140103 ) ) ;
#196087=DIRECTION ( 'NONE',  ( -0.000000000000000000, 1.000000000000000000, -0.000000000000000000 ) ) ;
#196088=ORIENTED_EDGE ( 'NONE', *, *, #66969, .F. ) ;
#196109=CARTESIAN_POINT ( 'NONE',  ( -11.94105721237523099, 10.19999999999999929, -1.187919463087248939 ) ) ;
#196119=ORIENTED_EDGE ( 'NONE', *, *, #15602, .F. ) ;
#196165=CARTESIAN_POINT ( 'NONE',  ( -11.89942855770814134, 12.30000000000000071, 0.6999999999999992895 ) ) ;
#196177=CARTESIAN_POINT ( 'NONE',  ( -11.48243876534946217, 12.29999999999998295, 3.199999999999997957 ) ) ;
#196188=( NAMED_UNIT ( * ) PLANE_ANGLE_UNIT ( ) SI_UNIT ( $, .RADIAN. ) );
#196189=PRESENTATION_STYLE_ASSIGNMENT (( #146395 ) ) ;
#196276=CARTESIAN_POINT ( 'NONE',  ( 11.07790593930098311, 13.79999999999999893, 0.6999999999999992895 ) ) ;
#196316=ORIENTED_EDGE ( 'NONE', *, *, #194701, .F. ) ;
#196354=ADVANCED_FACE ( 'NONE', ( #153271 ), #103461, .F. ) ;
#196360=EDGE_CURVE ( 'NONE', #95942, #116100, #212479, .T. ) ;
#196366=CARTESIAN_POINT ( 'NONE',  ( 9.681426354872456841, 13.43812210156014508, -8.165041025796162089 ) ) ;
#196368=ORIENTED_EDGE ( 'NONE', *, *, #210558, .T. ) ;
#196383=CARTESIAN_POINT ( 'NONE',  ( -11.92046840572485777, 11.15252124794268695, 1.382231356234940867 ) ) ;
#196415=EDGE_CURVE ( 'NONE', #129544, #93416, #36721, .T. ) ;
#196417=CARTESIAN_POINT ( 'NONE',  ( -11.91110530558079006, 8.003273469779060179, -1.051614653808552013 ) ) ;
#196421=CARTESIAN_POINT ( 'NONE',  ( -10.91033749632886973, 4.885617943545219610, -4.996452313011736202 ) ) ;
#196445=MECHANICAL_DESIGN_GEOMETRIC_PRESENTATION_REPRESENTATION('',(#6243),#16596);
#196446=AXIS2_PLACEMENT_3D ( 'NONE', #48275, #181435, #213911 ) ;
#196448=CARTESIAN_POINT ( 'NONE',  ( -15.75000000000000000, 11.29999999999999893, -0.7000000000000009548 ) ) ;
#196465=CARTESIAN_POINT ( 'NONE',  ( 8.982121351223291583, 14.65570953369224050, -7.241029012671043930 ) ) ;
#196468=CARTESIAN_POINT ( 'NONE',  ( 8.825981184337843288, 13.64596675382960100, 9.281099656089114802 ) ) ;
#196498=CARTESIAN_POINT ( 'NONE',  ( -10.93359526636954193, 4.740328704497578372, 4.433404364989353752 ) ) ;
#196518=CARTESIAN_POINT ( 'NONE',  ( -9.437944175107181977, 14.51387423797986642, 7.411204044495644183 ) ) ;
#196526=CARTESIAN_POINT ( 'NONE',  ( 11.28784473853554537, 8.874586039915849156, -4.090552291126032358 ) ) ;
#196531=MECHANICAL_DESIGN_GEOMETRIC_PRESENTATION_REPRESENTATION('',(#206871),#51345);
#196553=CARTESIAN_POINT ( 'NONE',  ( 10.97011102005664185, 13.79999999999998472, 1.696376167609456198 ) ) ;
#196563=CARTESIAN_POINT ( 'NONE',  ( -7.093554249807959344, 14.55189866933985421, -9.633885861679724272 ) ) ;
#196571=CARTESIAN_POINT ( 'NONE',  ( -15.75000000000000000, 10.89999999999998259, 1.799999999999999600 ) ) ;
#196575=CARTESIAN_POINT ( 'NONE',  ( -11.91093491413953309, 8.002894165250459935, -1.053637727194525642 ) ) ;
#196583=CARTESIAN_POINT ( 'NONE',  ( -10.49167095263961613, 5.343775707538775066, -5.730694126968514546 ) ) ;
#196594=ORIENTED_EDGE ( 'NONE', *, *, #20726, .T. ) ;
#196604=EDGE_CURVE ( 'NONE', #207604, #185122, #168320, .T. ) ;
#196606=DIRECTION ( 'NONE',  ( 0.000000000000000000, 1.000000000000000000, 0.000000000000000000 ) ) ;
#196643=CARTESIAN_POINT ( 'NONE',  ( -0.008622056139523381901, 15.44694768828586540, 11.95585894197802013 ) ) ;
#196652=CARTESIAN_POINT ( 'NONE',  ( 9.444297818688886181, 3.530917896769821152, 7.404075800242620353 ) ) ;
#196722=UNCERTAINTY_MEASURE_WITH_UNIT (LENGTH_MEASURE( 1.000000000000000082E-05 ), #25166, 'distance_accuracy_value', 'NONE');
#196764=ORIENTED_EDGE ( 'NONE', *, *, #106881, .T. ) ;
#196777=CARTESIAN_POINT ( 'NONE',  ( -15.75000000000000000, 9.799999999999982947, 3.199999999999997957 ) ) ;
#196779=ORIENTED_EDGE ( 'NONE', *, *, #197807, .T. ) ;
#196781=VECTOR ( 'NONE', #160017, 1000.000000000000000 ) ;
#196782=( NAMED_UNIT ( * ) PLANE_ANGLE_UNIT ( ) SI_UNIT ( $, .RADIAN. ) );
#196848=ADVANCED_FACE ( 'NONE', ( #27542 ), #39525, .F. ) ;
#196856=CARTESIAN_POINT ( 'NONE',  ( 8.731030487143305763, 13.51342317695541873, -8.232470247100428296 ) ) ;
#196862=ORIENTED_EDGE ( 'NONE', *, *, #83855, .T. ) ;
#196865=CARTESIAN_POINT ( 'NONE',  ( 8.846954724764692912, 13.14807067402342255, -7.639157931441056704 ) ) ;
#196868=ORIENTED_EDGE ( 'NONE', *, *, #69678, .F. ) ;
#196876=CARTESIAN_POINT ( 'NONE',  ( 0.000000000000000000, 4.446947634372834912, 11.95586206896558146 ) ) ;
#196890=CARTESIAN_POINT ( 'NONE',  ( -11.89829993707161648, 11.32919228251126142, -1.561606677374349772 ) ) ;
#196892=SURFACE_STYLE_USAGE ( .BOTH. , #210993 ) ;
#196895=CARTESIAN_POINT ( 'NONE',  ( 1.349890321011279370, 8.200329036966271801, 10.79298809153610073 ) ) ;
#196898=CARTESIAN_POINT ( 'NONE',  ( -9.367496997601190145, 14.57669131240758276, 7.413898975931879853 ) ) ;
#196900=ORIENTED_EDGE ( 'NONE', *, *, #14467, .F. ) ;
#196921=DIRECTION ( 'NONE',  ( 0.000000000000000000, 0.000000000000000000, -1.000000000000000000 ) ) ;
#196941=ORIENTED_EDGE ( 'NONE', *, *, #196604, .F. ) ;
#196977=ORIENTED_EDGE ( 'NONE', *, *, #126765, .T. ) ;
#197015=CARTESIAN_POINT ( 'NONE',  ( -11.81900460097218186, 12.34242865125860078, 1.592493057836596115 ) ) ;
#197019=ORIENTED_EDGE ( 'NONE', *, *, #24813, .F. ) ;
#197068=B_SPLINE_CURVE_WITH_KNOTS ( 'NONE', 3,
 ( #119969, #185946, #5045, #170779, #72189, #155607 ),
 .UNSPECIFIED., .F., .F.,
 ( 4, 2, 4 ),
 ( 0.000000000000000000, 3.619701867372329955E-05, 7.239403734744659911E-05 ),
 .UNSPECIFIED. ) ;
#197071=CARTESIAN_POINT ( 'NONE',  ( 8.118347949970196709, 14.25971613632666823, 8.777447096691743056 ) ) ;
#197091=CARTESIAN_POINT ( 'NONE',  ( 11.41108574530281494, 12.34163144622374375, -3.405883542057589253 ) ) ;
#197107=ADVANCED_FACE ( 'NONE', ( #1054 ), #206337, .F. ) ;
#197123=ORIENTED_EDGE ( 'NONE', *, *, #2690, .F. ) ;
#197125=FILL_AREA_STYLE ('',( #2094 ) ) ;
#197130=LINE ( 'NONE', #48768, #16651 ) ;
#197137=( NAMED_UNIT ( * ) PLANE_ANGLE_UNIT ( ) SI_UNIT ( $, .RADIAN. ) );
#197140=EDGE_LOOP ( 'NONE', ( #138259, #207906, #91763, #19944 ) ) ;
#197149=DIRECTION ( 'NONE',  ( 0.9632918427306580433, 0.000000000000000000, -0.2684563758389303945 ) ) ;
#197154=CARTESIAN_POINT ( 'NONE',  ( -11.52546672121288296, 8.148966486963653111, -3.186023502380144645 ) ) ;
#197155=DIRECTION ( 'NONE',  ( 0.000000000000000000, 0.000000000000000000, -1.000000000000000000 ) ) ;
#197165=CARTESIAN_POINT ( 'NONE',  ( -10.50000000000000000, 0.000000000000000000, 3.599999999999999201 ) ) ;
#197202=CARTESIAN_POINT ( 'NONE',  ( -10.04024307340833566, 4.584664385129866737, -6.492703511775993697 ) ) ;
#197204=ORIENTED_EDGE ( 'NONE', *, *, #193907, .T. ) ;
#197221=CARTESIAN_POINT ( 'NONE',  ( -11.86145017354119879, 13.50485634456125261, -1.100000000000000533 ) ) ;
#197222=( BOUNDED_SURFACE ( )  B_SPLINE_SURFACE ( 3, 2, ( 
 ( #185336, #118282, #20693 ),
 ( #82508, #148595, #36960 ),
 ( #99841, #68375, #164 ),
 ( #184267, #35892, #168037 ),
 ( #19640, #120428, #69441 ),
 ( #66231, #149659, #133440 ) ),
 .UNSPECIFIED., .F., .F., .F. ) 
 B_SPLINE_SURFACE_WITH_KNOTS ( ( 4, 2, 4 ),
 ( 3, 3 ),
 ( 0.000000000000000000, 0.0003766365702389428338, 0.0007532731404778856676 ),
 ( 0.000000000000000000, 1.000000000000000000 ),
 .UNSPECIFIED. ) 
 GEOMETRIC_REPRESENTATION_ITEM ( )  RATIONAL_B_SPLINE_SURFACE ( (
 ( 1.000000000000000000, 0.7452309222762957264, 1.000000000000000000),
 ( 1.000000000000000000, 0.7451892422674365468, 1.000000000000000000),
 ( 1.000000000000000000, 0.7429606254235103791, 1.000000000000000000),
 ( 1.000000000000000000, 0.7311462761269298394, 1.000000000000000000),
 ( 1.000000000000000000, 0.7212257702788642533, 1.000000000000000000),
 ( 1.000000000000000000, 0.7071067811865551223, 1.000000000000000000) ) ) 
 REPRESENTATION_ITEM ( '' )  SURFACE ( )  );
#197233=SURFACE_STYLE_FILL_AREA ( #78159 ) ;
#197257=LINE ( 'NONE', #13180, #124675 ) ;
#197258=EDGE_CURVE ( 'NONE', #108056, #80159, #125581, .T. ) ;
#197274=ORIENTED_EDGE ( 'NONE', *, *, #43007, .T. ) ;
#197301=CARTESIAN_POINT ( 'NONE',  ( -9.342754679277470942, 15.44694753537003962, -7.460282140120185090 ) ) ;
#197304=B_SPLINE_CURVE_WITH_KNOTS ( 'NONE', 3,
 ( #158748, #25534, #206417, #159808, #125264, #77487 ),
 .UNSPECIFIED., .F., .F.,
 ( 4, 2, 4 ),
 ( 0.000000000000000000, 0.0003767011250903910184, 0.0007534022501807820368 ),
 .UNSPECIFIED. ) ;
#197321=VERTEX_POINT ( 'NONE', #132229 ) ;
#197327=CARTESIAN_POINT ( 'NONE',  ( 11.44779963594995564, 10.90000000000000391, -3.600000000000078693 ) ) ;
#197346=EDGE_LOOP ( 'NONE', ( #144076, #127491, #154531, #202735 ) ) ;
#197353=FILL_AREA_STYLE_COLOUR ( '', #202759 ) ;
#197354=CARTESIAN_POINT ( 'NONE',  ( 11.86687215968023601, 11.10942212305790022, -1.056395335932036383 ) ) ;
#197365=VERTEX_POINT ( 'NONE', #38956 ) ;
#197375=DIRECTION ( 'NONE',  ( -0.2684563758389253985, 0.000000000000000000, 0.9632918427306595976 ) ) ;
#197386=ORIENTED_EDGE ( 'NONE', *, *, #12829, .T. ) ;
#197387=CARTESIAN_POINT ( 'NONE',  ( -15.75000000000000000, 10.90000000000000036, -1.400000000000001910 ) ) ;
#197395=CARTESIAN_POINT ( 'NONE',  ( -11.81911962874442068, 9.842894265158834699, -1.591749704452499303 ) ) ;
#197401=AXIS2_PLACEMENT_3D ( 'NONE', #141107, #172507, #106480 ) ;
#197414=CARTESIAN_POINT ( 'NONE',  ( 8.390031855354989077, 12.96148178021487318, 8.510248056045641718 ) ) ;
#197465=CARTESIAN_POINT ( 'NONE',  ( -11.51813239974987191, 7.080297235915058884, -3.210003848481874922 ) ) ;
#197481=MECHANICAL_DESIGN_GEOMETRIC_PRESENTATION_REPRESENTATION('',(#86792),#79971);
#197486=ORIENTED_EDGE ( 'NONE', *, *, #64145, .F. ) ;
#197488=CIRCLE ( 'NONE', #207841, 12.00000000000000178 ) ;
#197500=DIRECTION ( 'NONE',  ( 0.000000000000000000, -1.000000000000000000, -0.000000000000000000 ) ) ;
#197513=CARTESIAN_POINT ( 'NONE',  ( 10.07587973459925124, 13.99570152553757474, -7.402601053387023455 ) ) ;
#197544=CARTESIAN_POINT ( 'NONE',  ( -10.90756946389101323, 4.636105284860338571, -4.485523696119586567 ) ) ;
#197565=CARTESIAN_POINT ( 'NONE',  ( -9.438383064798124167, 14.67447095286016001, 7.309821827705476061 ) ) ;
#197573=CARTESIAN_POINT ( 'NONE',  ( 10.41996096743601186, 10.52647388830694375, -5.960368362366588180 ) ) ;
#197587=CARTESIAN_POINT ( 'NONE',  ( 11.87815913191725947, 12.29692179368584881, -1.708869976696599791 ) ) ;
#197621=CARTESIAN_POINT ( 'NONE',  ( -11.96431501343968584, 7.947166663703205458, 1.055127650031288278 ) ) ;
#197622=ADVANCED_FACE ( 'NONE', ( #101818 ), #6426, .T. ) ;
#197630=CARTESIAN_POINT ( 'NONE',  ( -11.59406913519968363, 8.291489155621126983, -2.927768694594159893 ) ) ;
#197638=VERTEX_POINT ( 'NONE', #100747 ) ;
#197667=VERTEX_POINT ( 'NONE', #85562 ) ;
#197679=CARTESIAN_POINT ( 'NONE',  ( -10.98550897202509269, 12.34280431172945214, 1.591908179352832242 ) ) ;
#197687=DIRECTION ( 'NONE',  ( -3.491481338843133750E-15, -0.000000000000000000, -1.000000000000000000 ) ) ;
#197688=PLANE ( 'NONE',  #86734 ) ;
#197696=B_SPLINE_CURVE_WITH_KNOTS ( 'NONE', 3,
 ( #124764, #157188, #42387, #92210, #205913, #191789 ),
 .UNSPECIFIED., .F., .F.,
 ( 4, 2, 4 ),
 ( 0.000000000000000000, 0.0003205138222656014457, 0.0006410276445312028913 ),
 .UNSPECIFIED. ) ;
#197721=STYLED_ITEM ( 'NONE', ( #151966 ), #172902 ) ;
#197737=TOROIDAL_SURFACE ( 'NONE', #208103, 11.92000000000000171, 0.08000000000000000167 ) ;
#197785=COLOUR_RGB ( '', 0.72549020, 0.75294118, 0.79215686) ;
#197798=CARTESIAN_POINT ( 'NONE',  ( -10.45142682343936791, 5.144546645612242841, 5.216777551074719632 ) ) ;
#197807=EDGE_CURVE ( 'NONE', #94599, #108406, #108448, .T. ) ;
#197814=EDGE_CURVE ( 'NONE', #54188, #35130, #147131, .T. ) ;
#197829=( NAMED_UNIT ( * ) PLANE_ANGLE_UNIT ( ) SI_UNIT ( $, .RADIAN. ) );
#197833=ORIENTED_EDGE ( 'NONE', *, *, #183770, .F. ) ;
#197839=CARTESIAN_POINT ( 'NONE',  ( -11.88235317400313917, 9.843357602269703577, 0.9089793033029933689 ) ) ;
#197865=CARTESIAN_POINT ( 'NONE',  ( 11.97929049433705373, 9.719999999999998863, -0.7046979865771821894 ) ) ;
#197866=DIRECTION ( 'NONE',  ( 1.000000000000000000, -0.000000000000000000, -0.000000000000000000 ) ) ;
#197868=CARTESIAN_POINT ( 'NONE',  ( 11.89942855770814312, 9.799999999999998934, -0.7000000000000009548 ) ) ;
#197872=CARTESIAN_POINT ( 'NONE',  ( -15.75000000000000000, 10.89999999999998259, 3.599999999999999201 ) ) ;
#197895=CARTESIAN_POINT ( 'NONE',  ( -9.505468521307150809, 5.017170101577987928, -6.783879874543660371 ) ) ;
#197909=B_SPLINE_CURVE_WITH_KNOTS ( 'NONE', 3,
 ( #49072, #131429, #113067, #198484, #179073, #30694 ),
 .UNSPECIFIED., .F., .F.,
 ( 4, 2, 4 ),
 ( 0.001877801214402442754, 0.002190719108449961511, 0.002503637002497480051 ),
 .UNSPECIFIED. ) ;
#197910=CARTESIAN_POINT ( 'NONE',  ( 8.868211955184602147, 12.79485499900459367, -8.085349282452083841 ) ) ;
#197918=( LENGTH_UNIT ( ) NAMED_UNIT ( * ) SI_UNIT ( .MILLI., .METRE. ) );
#197919=CARTESIAN_POINT ( 'NONE',  ( 10.20449125605852458, 13.21811437223454178, 7.146917523142401585 ) ) ;
#197925=CIRCLE ( 'NONE', #121965, 11.09999999999999964 ) ;
#197927=( GEOMETRIC_REPRESENTATION_CONTEXT ( 3 ) GLOBAL_UNCERTAINTY_ASSIGNED_CONTEXT ( ( #70949 ) ) GLOBAL_UNIT_ASSIGNED_CONTEXT ( ( #108005, #207555, #174032 ) ) REPRESENTATION_CONTEXT ( 'NONE', 'WORKASPACE' ) );
#197931=CARTESIAN_POINT ( 'NONE',  ( 8.433462717895558569, 14.01452863678292715, -8.474055829133085638 ) ) ;
#197933=ORIENTED_EDGE ( 'NONE', *, *, #194701, .T. ) ;
#197947=FILL_AREA_STYLE ('',( #144986 ) ) ;
#197970=DIRECTION ( 'NONE',  ( -0.000000000000000000, 1.000000000000000000, -0.000000000000000000 ) ) ;
#197971=EDGE_CURVE ( 'NONE', #191521, #191009, #106367, .T. ) ;
#197992=DIRECTION ( 'NONE',  ( 0.000000000000000000, -0.000000000000000000, 1.000000000000000000 ) ) ;
#197993=AXIS2_PLACEMENT_3D ( 'NONE', #39893, #103822, #106003 ) ;
#197995=TOROIDAL_SURFACE ( 'NONE', #132352, 12.17999999982603576, 0.5000000000000008882 ) ;
#198008=FILL_AREA_STYLE ('',( #165518 ) ) ;
#198031=DIRECTION ( 'NONE',  ( -0.000000000000000000, 1.000000000000000000, 9.023263958591317418E-17 ) ) ;
#198042=SURFACE_SIDE_STYLE ('',( #50736 ) ) ;
#198088=DIRECTION ( 'NONE',  ( -0.000000000000000000, -1.000000000000000000, -0.000000000000000000 ) ) ;
#198128=CARTESIAN_POINT ( 'NONE',  ( 7.327176377373612048, 14.51562980571618056, 9.506369224037232613 ) ) ;
#198182=ADVANCED_FACE ( 'NONE', ( #81044 ), #82099, .F. ) ;
#198198=ADVANCED_FACE ( 'NONE', ( #78896 ), #95976, .T. ) ;
#198226=CYLINDRICAL_SURFACE ( 'NONE', #1668, 0.3999999999999993006 ) ;
#198227=DIRECTION ( 'NONE',  ( 0.1510067114093955887, 0.000000000000000000, -0.9885327375000383388 ) ) ;
#198234=DIRECTION ( 'NONE',  ( -0.8003905296791196111, 0.000000000000000000, -0.5994789404140719036 ) ) ;
#198256=CARTESIAN_POINT ( 'NONE',  ( -10.85951921430376288, 4.658322617273027433, 5.107420070442172388 ) ) ;
#198315=AXIS2_PLACEMENT_3D ( 'NONE', #69331, #120320, #52051 ) ;
#198322=CARTESIAN_POINT ( 'NONE',  ( 10.98546216864998826, 11.25741378991010677, -1.592236800091192395 ) ) ;
#198323=CARTESIAN_POINT ( 'NONE',  ( -9.470186914265017464, 4.005096909781187264, 6.837150237413082365 ) ) ;
#198330=VERTEX_POINT ( 'NONE', #15819 ) ;
#198337=ORIENTED_EDGE ( 'NONE', *, *, #47209, .T. ) ;
#198354=CARTESIAN_POINT ( 'NONE',  ( 11.89197369110779334, 9.799999999999998934, 0.8056055387119843703 ) ) ;
#198372=ORIENTED_EDGE ( 'NONE', *, *, #60772, .F. ) ;
#198379=CARTESIAN_POINT ( 'NONE',  ( 11.91294103507069302, 12.48539910043597345, 1.446263142085445041 ) ) ;
#198380=CARTESIAN_POINT ( 'NONE',  ( -9.540655113774946017, 4.518459255872632419, 7.145788969735951568 ) ) ;
#198397=DIRECTION ( 'NONE',  ( -0.000000000000000000, 0.000000000000000000, -1.000000000000000000 ) ) ;
#198408=CARTESIAN_POINT ( 'NONE',  ( 11.94651559118242901, 11.15130655878981791, -1.135242698369562042 ) ) ;
#198459=CYLINDRICAL_SURFACE ( 'NONE', #56633, 0.3999999999999997446 ) ;
#198471=CARTESIAN_POINT ( 'NONE',  ( 10.87630568456067692, 9.715185551068161729, 7.311958335779218388 ) ) ;
#198484=CARTESIAN_POINT ( 'NONE',  ( 11.04986239659823433, 12.49060768514300079, -1.056426191432995765 ) ) ;
#198490=DIRECTION ( 'NONE',  ( -0.000000000000000000, -1.000000000000000000, -0.000000000000000000 ) ) ;
#198512=ORIENTED_EDGE ( 'NONE', *, *, #36673, .F. ) ;
#198514=EDGE_CURVE ( 'NONE', #49203, #7674, #199673, .T. ) ;
#198533=( BOUNDED_SURFACE ( )  B_SPLINE_SURFACE ( 3, 2, ( 
 ( #35605, #19351, #86500 ),
 ( #122301, #51879, #38822 ),
 ( #136334, #201289, #135274 ),
 ( #88652, #36670, #20418 ),
 ( #85431, #102759, #119064 ),
 ( #188258, #121224, #168814 ) ),
 .UNSPECIFIED., .F., .F., .T. ) 
 B_SPLINE_SURFACE_WITH_KNOTS ( ( 4, 2, 4 ),
 ( 3, 3 ),
 ( 0.000000000000000000, 0.0003831327362561326704, 0.0007662654725122653408 ),
 ( 0.000000000000000000, 1.000000000000000000 ),
 .UNSPECIFIED. ) 
 GEOMETRIC_REPRESENTATION_ITEM ( )  RATIONAL_B_SPLINE_SURFACE ( (
 ( 1.000000000000000000, 0.5879095031487664436, 1.000000000000000000),
 ( 1.000000000000000000, 0.5873691247589374331, 1.000000000000000000),
 ( 1.000000000000000000, 0.6054349545483206363, 1.000000000000000000),
 ( 1.000000000000000000, 0.6533334602780871414, 1.000000000000000000),
 ( 1.000000000000000000, 0.6828746263140246242, 1.000000000000000000),
 ( 1.000000000000000000, 0.7071067811865475727, 1.000000000000000000) ) ) 
 REPRESENTATION_ITEM ( '' )  SURFACE ( )  );
#198565=CARTESIAN_POINT ( 'NONE',  ( 9.082291402135501457, 13.43266975004936192, -9.116315574465707172 ) ) ;
#198585=CARTESIAN_POINT ( 'NONE',  ( 11.91826848330681976, 13.50729645956968206, -1.400000080589506757 ) ) ;
#198660=CARTESIAN_POINT ( 'NONE',  ( 0.000000000000000000, 9.719999999999998863, 0.000000000000000000 ) ) ;
#198671=FACE_OUTER_BOUND ( 'NONE', #142317, .T. ) ;
#198675=CARTESIAN_POINT ( 'NONE',  ( -11.95360554405576714, 12.49555003497401451, -1.059413164304690680 ) ) ;
#198677=CARTESIAN_POINT ( 'NONE',  ( -11.26733562030481473, 6.406227745073034718, -3.999921830493572195 ) ) ;
#198685=CARTESIAN_POINT ( 'NONE',  ( -10.66331579904126414, 5.901770781639986474, 5.511956274691907076 ) ) ;
#198688=SURFACE_STYLE_USAGE ( .BOTH. , #68683 ) ;
#198718=ORIENTED_EDGE ( 'NONE', *, *, #74380, .F. ) ;
#198748=STYLED_ITEM ( 'NONE', ( #49044 ), #186074 ) ;
#198793=VERTEX_POINT ( 'NONE', #146942 ) ;
#198797=SURFACE_STYLE_FILL_AREA ( #85068 ) ;
#198798=EDGE_CURVE ( 'NONE', #210726, #193462, #71651, .T. ) ;
#198807=AXIS2_PLACEMENT_3D ( 'NONE', #68215, #187315, #117055 ) ;
#198816=FILL_AREA_STYLE ('',( #66665 ) ) ;
#198819=( NAMED_UNIT ( * ) SI_UNIT ( $, .STERADIAN. ) SOLID_ANGLE_UNIT ( ) );
#198847=CARTESIAN_POINT ( 'NONE',  ( -8.065673753976707161, 15.99999996918363010, -8.613976771941846522 ) ) ;
#198849=CARTESIAN_POINT ( 'NONE',  ( -10.57232898948313604, 5.599354254162436817, 4.968808419985093039 ) ) ;
#198860=VERTEX_POINT ( 'NONE', #166459 ) ;
#198869=VERTEX_POINT ( 'NONE', #114582 ) ;
#198880=VERTEX_POINT ( 'NONE', #173960 ) ;
#198907=DIRECTION ( 'NONE',  ( 0.000000000000000000, 1.000000000000000000, 0.000000000000000000 ) ) ;
#198912=ORIENTED_EDGE ( 'NONE', *, *, #61190, .F. ) ;
#198935=ORIENTED_EDGE ( 'NONE', *, *, #186335, .F. ) ;
#198945=CARTESIAN_POINT ( 'NONE',  ( -9.917242840447775265, 4.174869238508773783, -6.172972641688763140 ) ) ;
#198961=CARTESIAN_POINT ( 'NONE',  ( 9.967295635675853305, 9.878600899727834062, 6.621762730473949254 ) ) ;
#198965=ORIENTED_EDGE ( 'NONE', *, *, #134782, .F. ) ;
#198970=ORIENTED_EDGE ( 'NONE', *, *, #6610, .F. ) ;
#198972=CARTESIAN_POINT ( 'NONE',  ( 10.28861420900376089, 12.75941440320506004, 6.944769193408874663 ) ) ;
#198975=EDGE_LOOP ( 'NONE', ( #14234, #135417, #27042, #59794 ) ) ;
#198983=CARTESIAN_POINT ( 'NONE',  ( 7.971049111166076173, 14.32663455170581379, -8.970823572502334642 ) ) ;
#198987=CARTESIAN_POINT ( 'NONE',  ( 11.78331023100045627, 11.29999999999999893, -1.800000000000001155 ) ) ;
#198988=CARTESIAN_POINT ( 'NONE',  ( 0.01853509810217068496, 14.54321759157664395, 11.97163369463103599 ) ) ;
#199002=DIRECTION ( 'NONE',  ( 1.000000000000000000, -0.000000000000000000, -0.000000000000000000 ) ) ;
#199028=CARTESIAN_POINT ( 'NONE',  ( -10.91033749632886973, 4.885617943545219610, -4.996452313011736202 ) ) ;
#199034=ORIENTED_EDGE ( 'NONE', *, *, #195328, .F. ) ;
#199090=SURFACE_STYLE_USAGE ( .BOTH. , #198042 ) ;
#199094=CARTESIAN_POINT ( 'NONE',  ( 11.52483635780546045, 12.22000008642463165, 3.345866325258042284 ) ) ;
#199114=DIRECTION ( 'NONE',  ( 0.000000000000000000, 0.000000000000000000, -1.000000000000000000 ) ) ;
#199127=( NAMED_UNIT ( * ) SI_UNIT ( $, .STERADIAN. ) SOLID_ANGLE_UNIT ( ) );
#199136=CARTESIAN_POINT ( 'NONE',  ( -9.508795732819951496, 14.91378867702411171, -7.212928819065533403 ) ) ;
#199173=DIRECTION ( 'NONE',  ( 0.8003905289055504024, -4.396526966619893387E-05, 0.5994789398347104559 ) ) ;
#199179=CARTESIAN_POINT ( 'NONE',  ( 7.860983254381821439, 14.39106760530863838, 9.010984000332380006 ) ) ;
#199214=ORIENTED_EDGE ( 'NONE', *, *, #120681, .F. ) ;
#199221=CARTESIAN_POINT ( 'NONE',  ( 11.87815913191726125, 9.796921793685850588, -1.708869976696599347 ) ) ;
#199234=EDGE_LOOP ( 'NONE', ( #167954, #17839, #118239, #209217 ) ) ;
#199236=CARTESIAN_POINT ( 'NONE',  ( 6.928203230275522095, 15.51887838114830132, 9.797958971132704420 ) ) ;
#199238=CARTESIAN_POINT ( 'NONE',  ( -9.587704862635016312, 4.026159954882873926, 6.671158199369250141 ) ) ;
#199253=MECHANICAL_DESIGN_GEOMETRIC_PRESENTATION_REPRESENTATION('',(#57967),#81775);
#199287=DIRECTION ( 'NONE',  ( -0.05872483221476467591, -7.952201780260630618E-17, 0.9982742078614211811 ) ) ;
#199299=CARTESIAN_POINT ( 'NONE',  ( 1.313174662617409227, 8.310476012147654856, -10.86148356754324773 ) ) ;
#199316=SURFACE_SIDE_STYLE ('',( #70375 ) ) ;
#199317=DIRECTION ( 'NONE',  ( 0.000000000000000000, 0.000000000000000000, -1.000000000000000000 ) ) ;
#199318=EDGE_LOOP ( 'NONE', ( #196900, #117477, #58457, #78328 ) ) ;
#199326=CARTESIAN_POINT ( 'NONE',  ( 0.000000000000000000, 4.446947634372835800, 0.000000000000000000 ) ) ;
#199338=CARTESIAN_POINT ( 'NONE',  ( -11.86239285000045918, 13.88000000000000078, -1.812080536912752837 ) ) ;
#199350=CARTESIAN_POINT ( 'NONE',  ( -11.33772463945036968, 13.40000000000000036, -3.600000000000002309 ) ) ;
#199356=PRESENTATION_STYLE_ASSIGNMENT (( #132287 ) ) ;
#199362=VECTOR ( 'NONE', #9123, 1000.000000000000000 ) ;
#199404=ORIENTED_EDGE ( 'NONE', *, *, #156764, .T. ) ;
#199406=B_SPLINE_CURVE_WITH_KNOTS ( 'NONE', 3,
 ( #95391, #62850, #177686, #194989, #63919, #79100 ),
 .UNSPECIFIED., .F., .F.,
 ( 4, 2, 4 ),
 ( 0.001877801214402442754, 0.002190719108449961511, 0.002503637002497480051 ),
 .UNSPECIFIED. ) ;
#199418=EDGE_CURVE ( 'NONE', #57689, #20233, #203865, .T. ) ;
#199419=CARTESIAN_POINT ( 'NONE',  ( -9.393959922460844325, 15.45881633117845055, -7.466876303545585181 ) ) ;
#199426=CARTESIAN_POINT ( 'NONE',  ( -11.94654170777226021, 9.948256738410641731, 1.134972293687618539 ) ) ;
#199466=DIRECTION ( 'NONE',  ( 0.000000000000000000, 0.000000000000000000, -1.000000000000000000 ) ) ;
#199471=CARTESIAN_POINT ( 'NONE',  ( -0.2226028112648442414, 15.44694767462292440, -11.95586206701304199 ) ) ;
#199474=ORIENTED_EDGE ( 'NONE', *, *, #137412, .F. ) ;
#199501=DIRECTION ( 'NONE',  ( 0.000000000000000000, 0.000000000000000000, -1.000000000000000000 ) ) ;
#199504=CARTESIAN_POINT ( 'NONE',  ( 11.33772463945036790, 10.19999999999999929, -3.600000000000000977 ) ) ;
#199507=ORIENTED_EDGE ( 'NONE', *, *, #25664, .F. ) ;
#199511=VERTEX_POINT ( 'NONE', #26600 ) ;
#199516=FACE_OUTER_BOUND ( 'NONE', #26651, .T. ) ;
#199524=CARTESIAN_POINT ( 'NONE',  ( -11.58081452147585289, 6.132683923455591213, -5.154482061493088629 ) ) ;
#199526=SURFACE_STYLE_FILL_AREA ( #66314 ) ;
#199558=DIRECTION ( 'NONE',  ( -0.000000000000000000, -1.000000000000000000, -0.000000000000000000 ) ) ;
#199580=DIRECTION ( 'NONE',  ( 0.1510067114093955887, 0.000000000000000000, -0.9885327375000383388 ) ) ;
#199581=STYLED_ITEM ( 'NONE', ( #18182 ), #146262 ) ;
#199588=CARTESIAN_POINT ( 'NONE',  ( -10.19200560444942560, 4.477620260464512114, -5.707107691925500603 ) ) ;
#199589=CARTESIAN_POINT ( 'NONE',  ( -9.367496996292747014, 15.51845925588232333, -7.500000001629758550 ) ) ;
#199592=DIRECTION ( 'NONE',  ( -1.000000000000000000, 0.000000000000000000, 0.000000000000000000 ) ) ;
#199608=ORIENTED_EDGE ( 'NONE', *, *, #58273, .T. ) ;
#199636=CARTESIAN_POINT ( 'NONE',  ( 6.852217057538298128, 14.00000000000000000, -9.459770950306301884 ) ) ;
#199642=ORIENTED_EDGE ( 'NONE', *, *, #10029, .T. ) ;
#199653=CARTESIAN_POINT ( 'NONE',  ( 11.91826849282518275, 13.39999999999999858, -1.400000000000001465 ) ) ;
#199673=CIRCLE ( 'NONE', #47420, 11.09999999999999964 ) ;
#199686=CARTESIAN_POINT ( 'NONE',  ( 6.902720145097976712, 15.44736672593543148, 9.761920446463514978 ) ) ;
#199698=CARTESIAN_POINT ( 'NONE',  ( 11.97185388258315264, 13.87999990720392596, -0.8311143155443057040 ) ) ;
#199749=CARTESIAN_POINT ( 'NONE',  ( -10.84253909858433040, 4.919570308430903260, -5.035411995924087059 ) ) ;
#199757=CARTESIAN_POINT ( 'NONE',  ( -11.55895101287907067, 8.210663139309525960, 3.234169276427452111 ) ) ;
#199786=ORIENTED_EDGE ( 'NONE', *, *, #22230, .T. ) ;
#199802=DIRECTION ( 'NONE',  ( 0.9885327375000381167, 0.000000000000000000, -0.1510067114093955609 ) ) ;
#199808=CIRCLE ( 'NONE', #78763, 0.07999999999999998779 ) ;
#199847=( NAMED_UNIT ( * ) PLANE_ANGLE_UNIT ( ) SI_UNIT ( $, .RADIAN. ) );
#199852=AXIS2_PLACEMENT_3D ( 'NONE', #127914, #57485, #44449 ) ;
#199869=ORIENTED_EDGE ( 'NONE', *, *, #89552, .T. ) ;
#199875=PRESENTATION_STYLE_ASSIGNMENT (( #166324 ) ) ;
#199921=CARTESIAN_POINT ( 'NONE',  ( -3.796053574490474869, 15.00000000000207656, -12.24940615670125510 ) ) ;
#199924=CARTESIAN_POINT ( 'NONE',  ( -10.99931038725301846, 6.873658557531565627, -3.960823121322395224 ) ) ;
#199953=UNCERTAINTY_MEASURE_WITH_UNIT (LENGTH_MEASURE( 1.000000000000000082E-05 ), #135717, 'distance_accuracy_value', 'NONE');
#199955=FACE_OUTER_BOUND ( 'NONE', #182807, .T. ) ;
#199965=VECTOR ( 'NONE', #185441, 1000.000000000000000 ) ;
#199971=CARTESIAN_POINT ( 'NONE',  ( 11.33772463945036790, 19.00000000000000000, -3.680000000000002824 ) ) ;
#199993=CARTESIAN_POINT ( 'NONE',  ( 11.89197816957260478, 9.799999999999998934, -0.8055420615339534685 ) ) ;
#200012=ORIENTED_EDGE ( 'NONE', *, *, #100151, .T. ) ;
#200017=MECHANICAL_DESIGN_GEOMETRIC_PRESENTATION_REPRESENTATION('',(#175935),#117071);
#200022=CARTESIAN_POINT ( 'NONE',  ( -10.55260481140867235, 5.124873218919925755, -7.009574331923702495 ) ) ;
#200039=CARTESIAN_POINT ( 'NONE',  ( 9.280199541404417829, 11.48923774938119635, 7.537149123760571889 ) ) ;
#200040=EDGE_CURVE ( 'NONE', #80409, #138814, #96129, .T. ) ;
#200044=VERTEX_POINT ( 'NONE', #68952 ) ;
#200053=CARTESIAN_POINT ( 'NONE',  ( 9.267535596873369030, 13.53505500093428893, -6.807038118641733249 ) ) ;
#200056=EDGE_LOOP ( 'NONE', ( #176289, #107237, #26137, #85317 ) ) ;
#200062=CARTESIAN_POINT ( 'NONE',  ( -11.94105721237523277, 19.00000000000000000, -1.187919463087249827 ) ) ;
#200063=CARTESIAN_POINT ( 'NONE',  ( 8.381179344826065858, 14.06946724413340100, -8.588858344356935959 ) ) ;
#200065=AXIS2_PLACEMENT_3D ( 'NONE', #126023, #142227, #57744 ) ;
#200069=CARTESIAN_POINT ( 'NONE',  ( 10.50000000000000178, 10.19999999999998153, 3.599999999999999201 ) ) ;
#200092=( NAMED_UNIT ( * ) PLANE_ANGLE_UNIT ( ) SI_UNIT ( $, .RADIAN. ) );
#200108=VECTOR ( 'NONE', #103959, 1000.000000000000000 ) ;
#200122=VECTOR ( 'NONE', #132774, 1000.000000000000000 ) ;
#200168=UNCERTAINTY_MEASURE_WITH_UNIT (LENGTH_MEASURE( 1.000000000000000082E-05 ), #60805, 'distance_accuracy_value', 'NONE');
#200171=LINE ( 'NONE', #101626, #142937 ) ;
#200222=FILL_AREA_STYLE_COLOUR ( '', #139280 ) ;
#200250=CARTESIAN_POINT ( 'NONE',  ( 7.704529957180471733, 14.43789495343931506, 9.203201968345597450 ) ) ;
#200258=COLOUR_RGB ( '', 0.66274510, 0.83137255, 0.94901961) ;
#200304=ORIENTED_EDGE ( 'NONE', *, *, #212491, .T. ) ;
#200306=PRESENTATION_STYLE_ASSIGNMENT (( #68167 ) ) ;
#200311=LINE ( 'NONE', #69237, #151507 ) ;
#200327=( BOUNDED_SURFACE ( )  B_SPLINE_SURFACE ( 3, 2, ( 
 ( #183825, #82052, #113570 ),
 ( #49557, #101513, #115684 ),
 ( #147085, #100444, #31193 ),
 ( #66837, #64739, #117834 ),
 ( #167584, #18106, #116753 ),
 ( #33304, #132980, #165441 ),
 ( #130882, #198983, #35437 ),
 ( #114633, #179574, #85258 ),
 ( #34370, #97267, #131921 ),
 ( #80997, #200063, #135106 ),
 ( #197931, #151347, #148145 ),
 ( #14903, #17038, #68988 ),
 ( #214147, #150280, #2915 ),
 ( #83115, #166515, #149196 ) ),
 .UNSPECIFIED., .F., .F., .T. ) 
 B_SPLINE_SURFACE_WITH_KNOTS ( ( 4, 2, 2, 2, 2, 2, 4 ),
 ( 3, 3 ),
 ( 0.000000000000000000, 0.0007244816566593680670, 0.001086722484989051992, 0.001448963313318736134, 0.001811204141648420059, 0.002173444969978103984, 0.002897926626637472268 ),
 ( 0.000000000000000000, 1.000000000000000000 ),
 .UNSPECIFIED. ) 
 GEOMETRIC_REPRESENTATION_ITEM ( )  RATIONAL_B_SPLINE_SURFACE ( (
 ( 1.000000000000000000, 0.8509629433967720313, 1.000000000000000000),
 ( 1.000000000000000000, 0.8509409660886558813, 1.000000000000000000),
 ( 1.000000000000000000, 0.8506801742508753872, 1.000000000000000000),
 ( 1.000000000000000000, 0.8504573418716681044, 1.000000000000000000),
 ( 1.000000000000000000, 0.8503421207546283389, 1.000000000000000000),
 ( 1.000000000000000000, 0.8502290005389957495, 1.000000000000000000),
 ( 1.000000000000000000, 0.8502658874624668961, 1.000000000000000000),
 ( 1.000000000000000000, 0.8500987576256546774, 1.000000000000000000),
 ( 1.000000000000000000, 0.8497013267704406347, 1.000000000000000000),
 ( 1.000000000000000000, 0.8485069977425411247, 1.000000000000000000),
 ( 1.000000000000000000, 0.8477706576622060508, 1.000000000000000000),
 ( 1.000000000000000000, 0.8457454946330462686, 1.000000000000000000),
 ( 1.000000000000000000, 0.8445998729257416793, 1.000000000000000000),
 ( 1.000000000000000000, 0.8434733505592222347, 1.000000000000000000) ) ) 
 REPRESENTATION_ITEM ( '' )  SURFACE ( )  );
#200358=CARTESIAN_POINT ( 'NONE',  ( -11.89942855770814134, 12.30000000000000071, -0.7000000000000009548 ) ) ;
#200376=DIRECTION ( 'NONE',  ( 0.000000000000000000, -1.000000000000000000, -9.023263958591317418E-17 ) ) ;
#200379=EDGE_LOOP ( 'NONE', ( #94338, #90913, #66441, #21032 ) ) ;
#200384=FILL_AREA_STYLE_COLOUR ( '', #161587 ) ;
#200385=CARTESIAN_POINT ( 'NONE',  ( -10.17810690056512613, 3.623929045899029866, 6.361496871862332370 ) ) ;
#200400=CARTESIAN_POINT ( 'NONE',  ( 0.000000000000000000, 12.22000000000000064, 0.000000000000000000 ) ) ;
#200407=AXIS2_PLACEMENT_3D ( 'NONE', #95216, #132002, #161266 ) ;
#200412=ORIENTED_EDGE ( 'NONE', *, *, #129984, .F. ) ;
#200451=CARTESIAN_POINT ( 'NONE',  ( 6.928203230275524760, 14.48154074412737202, -9.797958971132702644 ) ) ;
#200452=CARTESIAN_POINT ( 'NONE',  ( -9.505648412044632067, 5.017053549588888828, 6.783778555801666776 ) ) ;
#200453=ORIENTED_EDGE ( 'NONE', *, *, #137597, .T. ) ;
#200459=ORIENTED_EDGE ( 'NONE', *, *, #125621, .T. ) ;
#200505=CARTESIAN_POINT ( 'NONE',  ( -10.77716609946257620, 4.490170579428209408, -5.280790421213856334 ) ) ;
#200573=ORIENTED_EDGE ( 'NONE', *, *, #176483, .T. ) ;
#200584=CARTESIAN_POINT ( 'NONE',  ( -11.31088518949709965, 5.182344123437907513, 5.726584094856639773 ) ) ;
#200596=CARTESIAN_POINT ( 'NONE',  ( 9.686381629184177555, 13.40773330361598248, 8.159561931930056744 ) ) ;
#200600=ORIENTED_EDGE ( 'NONE', *, *, #132358, .F. ) ;
#200612=CARTESIAN_POINT ( 'NONE',  ( -9.604686356149274573, 3.481540744127369802, 7.193747284969079558 ) ) ;
#200626=AXIS2_PLACEMENT_3D ( 'NONE', #78183, #194061, #44643 ) ;
#200631=CARTESIAN_POINT ( 'NONE',  ( -11.97929049433705373, 11.37999999999999901, -0.7046979865771834106 ) ) ;
#200646=CARTESIAN_POINT ( 'NONE',  ( -1.292128843000392768, 8.373613470998940045, -10.90074592850029767 ) ) ;
#200653=EDGE_CURVE ( 'NONE', #11477, #138322, #66889, .T. ) ;
#200665=ORIENTED_EDGE ( 'NONE', *, *, #114498, .F. ) ;
#200695=CARTESIAN_POINT ( 'NONE',  ( 7.459175572040564361, 13.90551515481552691, -8.979190973933295794 ) ) ;
#200702=ORIENTED_EDGE ( 'NONE', *, *, #117977, .F. ) ;
#200713=ORIENTED_EDGE ( 'NONE', *, *, #103222, .F. ) ;
#200715=COLOUR_RGB ( '', 0.08235294, 0.09019608, 0.10196078) ;
#200740=VERTEX_POINT ( 'NONE', #33307 ) ;
#200747=ORIENTED_EDGE ( 'NONE', *, *, #90049, .F. ) ;
#200757=CARTESIAN_POINT ( 'NONE',  ( 11.96212011828583677, 13.82812445049936834, -0.9569185076418588176 ) ) ;
#200767=CARTESIAN_POINT ( 'NONE',  ( 11.92050416151432835, 12.44794624720375786, -1.381922468431410866 ) ) ;
#200800=CARTESIAN_POINT ( 'NONE',  ( -11.97929049433705551, 12.22000000000000064, -0.7046979865771821894 ) ) ;
#200810=CARTESIAN_POINT ( 'NONE',  ( -10.49167311136684866, 5.343773310534622567, 5.730690286876301442 ) ) ;
#200820=( GEOMETRIC_REPRESENTATION_CONTEXT ( 3 ) GLOBAL_UNCERTAINTY_ASSIGNED_CONTEXT ( ( #161340 ) ) GLOBAL_UNIT_ASSIGNED_CONTEXT ( ( #71720, #56574, #122733 ) ) REPRESENTATION_CONTEXT ( 'NONE', 'WORKASPACE' ) );
#200824=CARTESIAN_POINT ( 'NONE',  ( 11.55950211276791251, 11.37999999999999901, -3.221476510067114329 ) ) ;
#200825=FILL_AREA_STYLE_COLOUR ( '', #142278 ) ;
#200836=ORIENTED_EDGE ( 'NONE', *, *, #211067, .F. ) ;
#200922=FILL_AREA_STYLE_COLOUR ( '', #61226 ) ;
#200946=CARTESIAN_POINT ( 'NONE',  ( -9.748756651491515157, 4.000000000000000888, 7.301653494243616649 ) ) ;
#200954=STYLED_ITEM ( 'NONE', ( #53801 ), #170192 ) ;
#200972=CARTESIAN_POINT ( 'NONE',  ( -6.671583288098925202, 14.00000000000492939, -9.747470831327131435 ) ) ;
#200974=CARTESIAN_POINT ( 'NONE',  ( -10.37109829931902816, 6.927524423111719898, -5.134218648570218591 ) ) ;
#201005=ORIENTED_EDGE ( 'NONE', *, *, #153308, .T. ) ;
#201079=CARTESIAN_POINT ( 'NONE',  ( 0.000000000000000000, 0.08000000000000020983, 0.000000000000000000 ) ) ;
#201080=CARTESIAN_POINT ( 'NONE',  ( -10.90756946389101323, 4.636105284860334130, -4.485523696119589232 ) ) ;
#201090=CARTESIAN_POINT ( 'NONE',  ( -10.57232049882948388, 5.599334429189661400, -4.968988939937085014 ) ) ;
#201096=CARTESIAN_POINT ( 'NONE',  ( 11.96883372729383055, 6.669921767506581389, -0.9937123909951041112 ) ) ;
#201101=ORIENTED_EDGE ( 'NONE', *, *, #110409, .F. ) ;
#201108=CARTESIAN_POINT ( 'NONE',  ( 8.806171940766569506, 13.38206018750110360, -7.684638306840279043 ) ) ;
#201109=MECHANICAL_DESIGN_GEOMETRIC_PRESENTATION_REPRESENTATION('',(#48859),#159560);
#201119=DIRECTION ( 'NONE',  ( 0.000000000000000000, 1.000000000000000000, 0.000000000000000000 ) ) ;
#201121=CARTESIAN_POINT ( 'NONE',  ( -4.933501174700577302E-10, 15.51845925587262975, -12.00000000000000355 ) ) ;
#201122=EDGE_LOOP ( 'NONE', ( #119301, #19705, #46167, #25319 ) ) ;
#201145=VERTEX_POINT ( 'NONE', #123209 ) ;
#201175=CIRCLE ( 'NONE', #107893, 0.08000000000000014044 ) ;
#201236=CARTESIAN_POINT ( 'NONE',  ( 9.998716872439858960, 9.834509080145350524, -6.644787476054019315 ) ) ;
#201250=EDGE_CURVE ( 'NONE', #30537, #172216, #100299, .T. ) ;
#201282=PLANE ( 'NONE',  #204948 ) ;
#201283=FACE_OUTER_BOUND ( 'NONE', #111020, .T. ) ;
#201289=CARTESIAN_POINT ( 'NONE',  ( 11.45846087878786790, 13.59311600781417972, 3.566076377698205846 ) ) ;
#201306=CARTESIAN_POINT ( 'NONE',  ( 11.44789321844504215, 12.29999999999998295, 3.303298730975393838 ) ) ;
#201311=CARTESIAN_POINT ( 'NONE',  ( -15.75000000000000000, 13.79999999999999893, -1.800000000000001155 ) ) ;
#201314=CARTESIAN_POINT ( 'NONE',  ( -1.448815997565459757, 7.903552007303734861, -10.65195286442483358 ) ) ;
#201330=VERTEX_POINT ( 'NONE', #183574 ) ;
#201334=FACE_OUTER_BOUND ( 'NONE', #111242, .T. ) ;
#201350=CARTESIAN_POINT ( 'NONE',  ( 11.86239285000045918, 9.719999999999998863, -1.812080536912753059 ) ) ;
#201366=CARTESIAN_POINT ( 'NONE',  ( 7.074468237148123784, 15.51887838114830309, 9.694533992922792720 ) ) ;
#201369=FACE_OUTER_BOUND ( 'NONE', #132276, .T. ) ;
#201377=CARTESIAN_POINT ( 'NONE',  ( -11.52901446936773944, 11.29425527467597412, 3.330874149801173356 ) ) ;
#201384=CIRCLE ( 'NONE', #170184, 0.07999999999999946043 ) ;
#201417=ORIENTED_EDGE ( 'NONE', *, *, #87595, .F. ) ;
#201418=AXIS2_PLACEMENT_3D ( 'NONE', #121410, #3277, #87757 ) ;
#201423=DIRECTION ( 'NONE',  ( -1.000000000000000000, 0.000000000000000000, 3.491481338843133355E-15 ) ) ;
#201435=CARTESIAN_POINT ( 'NONE',  ( -11.86145017031048177, 11.00581953513854394, 1.099999999999996980 ) ) ;
#201443=PLANE ( 'NONE',  #26736 ) ;
#201447=CARTESIAN_POINT ( 'NONE',  ( -9.367496997601300279, 15.00000000000599343, -7.499999999995378808 ) ) ;
#201454=ORIENTED_EDGE ( 'NONE', *, *, #126765, .F. ) ;
#201473=DIRECTION ( 'NONE',  ( -0.1510067114093955887, 0.000000000000000000, -0.9885327375000383388 ) ) ;
#201475=TOROIDAL_SURFACE ( 'NONE', #201636, 11.92000000000000171, 0.08000000000000000167 ) ;
#201490=VERTEX_POINT ( 'NONE', #86081 ) ;
#201496=B_SPLINE_CURVE_WITH_KNOTS ( 'NONE', 3,
 ( #119844, #185822, #103532, #169591, #21173, #54777, #90494, #187962 ),
 .UNSPECIFIED., .F., .F.,
 ( 4, 2, 2, 4 ),
 ( -5.999999999245582952E-08, 0.001012685428351500902, 0.001519058142527249765, 0.002025430856702998845 ),
 .UNSPECIFIED. ) ;
#201512=CARTESIAN_POINT ( 'NONE',  ( -9.970593900173907898, 5.552053933461305490, 5.997145116287158295 ) ) ;
#201527=DIRECTION ( 'NONE',  ( 0.000000000000000000, 0.000000000000000000, -1.000000000000000000 ) ) ;
#201542=CARTESIAN_POINT ( 'NONE',  ( -9.372067988322836385, 15.41907390678799494, -7.405912380499037440 ) ) ;
#201543=( GEOMETRIC_REPRESENTATION_CONTEXT ( 3 ) GLOBAL_UNCERTAINTY_ASSIGNED_CONTEXT ( ( #32340 ) ) GLOBAL_UNIT_ASSIGNED_CONTEXT ( ( #87568, #55069, #153635 ) ) REPRESENTATION_CONTEXT ( 'NONE', 'WORKASPACE' ) );
#201545=COLOUR_RGB ( '', 0.31764706, 0.68627451, 0.89019608) ;
#201561=AXIS2_PLACEMENT_3D ( 'NONE', #199326, #2180, #20579 ) ;
#201571=CARTESIAN_POINT ( 'NONE',  ( 11.91826849282518275, 12.69999999999997975, 1.399999999999998579 ) ) ;
#201583=DIRECTION ( 'NONE',  ( -0.000000000000000000, -0.000000000000000000, 1.000000000000000000 ) ) ;
#201626=CARTESIAN_POINT ( 'NONE',  ( 11.89942855770814312, 11.29999999999999893, 0.6999999999999992895 ) ) ;
#201635=ORIENTED_EDGE ( 'NONE', *, *, #154010, .F. ) ;
#201636=AXIS2_PLACEMENT_3D ( 'NONE', #84686, #150773, #149693 ) ;
#201647=CARTESIAN_POINT ( 'NONE',  ( -10.90756946389101323, 4.636105284860338571, -4.485523696119586567 ) ) ;
#201664=ORIENTED_EDGE ( 'NONE', *, *, #137524, .F. ) ;
#201672=AXIS2_PLACEMENT_3D ( 'NONE', #23462, #9367, #26678 ) ;
#201678=( BOUNDED_SURFACE ( )  B_SPLINE_SURFACE ( 3, 2, ( 
 ( #187975, #191168, #141423 ),
 ( #105705, #140341, #174962 ),
 ( #139252, #42835, #40689 ),
 ( #106792, #24392, #206359 ),
 ( #57986, #26544, #124149 ),
 ( #41764, #173903, #25478 ),
 ( #137118, #91585, #157637 ),
 ( #9235, #207429, #71005 ),
 ( #59048, #108941, #180278 ),
 ( #210631, #192233, #128418 ),
 ( #112149, #62257, #60117 ),
 ( #64391, #160827, #95851 ),
 ( #63322, #126276, #13494 ),
 ( #145688, #129483, #92652 ),
 ( #28693, #142473, #46028 ),
 ( #194385, #127348, #162970 ),
 ( #158694, #178151, #193317 ),
 ( #27615, #161907, #61188 ),
 ( #79569, #29766, #48169 ),
 ( #111071, #93715, #211686 ),
 ( #177077, #159756, #195465 ),
 ( #179217, #12419, #11353 ),
 ( #113212, #94779, #77434 ),
 ( #78499, #144616, #47096 ),
 ( #43896, #30842, #96919 ),
 ( #110010, #176023, #14550 ),
 ( #80646, #146738, #212756 ),
 ( #130535, #143551, #196526 ),
 ( #114282, #10292, #76366 ),
 ( #209545, #44963, #208481 ),
 ( #149913, #69689, #16677 ),
 ( #201817, #118529, #197573 ),
 ( #15613, #100084, #135793 ),
 ( #148835, #119599, #116391 ),
 ( #51339, #32956, #99031 ),
 ( #97979, #18808, #2546 ),
 ( #213800, #83820, #407 ),
 ( #134744, #165086, #49217 ) ),
 .UNSPECIFIED., .F., .F., .T. ) 
 B_SPLINE_SURFACE_WITH_KNOTS ( ( 4, 2, 2, 2, 2, 2, 2, 2, 2, 2, 2, 2, 2, 2, 2, 2, 2, 2, 4 ),
 ( 3, 3 ),
 ( -6.071532165918824830E-18, 0.001328702784605519409, 0.002657405569211044889, 0.003986108353816570152, 0.005314811138422095849, 0.005979162530724858697, 0.006643513923027621546, 0.007972216707633147242, 0.009300919492238671205, 0.01062962227684419690, 0.01129397366914695888, 0.01195832506144972260, 0.01328702784605524656, 0.01461573063066077226, 0.01594443341526629795, 0.01727313619987182192, 0.01860183898447734935, 0.01993054176908287678, 0.02125924455368840074 ),
 ( 0.000000000000000000, 1.000000000000000000 ),
 .UNSPECIFIED. ) 
 GEOMETRIC_REPRESENTATION_ITEM ( )  RATIONAL_B_SPLINE_SURFACE ( (
 ( 1.000000000000000000, 0.8435444081808770589, 1.000000000000000000),
 ( 1.000000000000000000, 0.8432483325082756886, 1.000000000000000000),
 ( 1.000000000000000000, 0.8427406575464768679, 1.000000000000000000),
 ( 1.000000000000000000, 0.8410405345067828442, 1.000000000000000000),
 ( 1.000000000000000000, 0.8398681797021982920, 1.000000000000000000),
 ( 1.000000000000000000, 0.8370024961260722485, 1.000000000000000000),
 ( 1.000000000000000000, 0.8353284867502276390, 1.000000000000000000),
 ( 1.000000000000000000, 0.8314541250028352204, 1.000000000000000000),
 ( 1.000000000000000000, 0.8292703529264303652, 1.000000000000000000),
 ( 1.000000000000000000, 0.8250608724160720664, 1.000000000000000000),
 ( 1.000000000000000000, 0.8247076902036051260, 1.000000000000000000),
 ( 1.000000000000000000, 0.8254996870500060924, 1.000000000000000000),
 ( 1.000000000000000000, 0.8265215800901872800, 1.000000000000000000),
 ( 1.000000000000000000, 0.8285699112141275968, 1.000000000000000000),
 ( 1.000000000000000000, 0.8294744577800686747, 1.000000000000000000),
 ( 1.000000000000000000, 0.8313365137719098685, 1.000000000000000000),
 ( 1.000000000000000000, 0.8318058077052401522, 1.000000000000000000),
 ( 1.000000000000000000, 0.8328176945125120856, 1.000000000000000000),
 ( 1.000000000000000000, 0.8334056329371573035, 1.000000000000000000),
 ( 1.000000000000000000, 0.8334130558649108789, 1.000000000000000000),
 ( 1.000000000000000000, 0.8331786830936150912, 1.000000000000000000),
 ( 1.000000000000000000, 0.8326565767077455105, 1.000000000000000000),
 ( 1.000000000000000000, 0.8323703136855602480, 1.000000000000000000),
 ( 1.000000000000000000, 0.8316300192767074329, 1.000000000000000000),
 ( 1.000000000000000000, 0.8314051384442139314, 1.000000000000000000),
 ( 1.000000000000000000, 0.8294588192946742433, 1.000000000000000000),
 ( 1.000000000000000000, 0.8281603792329889080, 1.000000000000000000),
 ( 1.000000000000000000, 0.8254551073024104513, 1.000000000000000000),
 ( 1.000000000000000000, 0.8237213491650171582, 1.000000000000000000),
 ( 1.000000000000000000, 0.8292902593114940268, 1.000000000000000000),
 ( 1.000000000000000000, 0.8313446087002768214, 1.000000000000000000),
 ( 1.000000000000000000, 0.8350647946855377368, 1.000000000000000000),
 ( 1.000000000000000000, 0.8366996347242240395, 1.000000000000000000),
 ( 1.000000000000000000, 0.8395672446973311276, 1.000000000000000000),
 ( 1.000000000000000000, 0.8407915391627092117, 1.000000000000000000),
 ( 1.000000000000000000, 0.8426130235641089428, 1.000000000000000000),
 ( 1.000000000000000000, 0.8431855836768197276, 1.000000000000000000),
 ( 1.000000000000000000, 0.8434758251109458760, 1.000000000000000000) ) ) 
 REPRESENTATION_ITEM ( '' )  SURFACE ( )  );
#201680=DIRECTION ( 'NONE',  ( -0.000000000000000000, 1.000000000000000000, -0.000000000000000000 ) ) ;
#201714=CARTESIAN_POINT ( 'NONE',  ( -15.75000000000000000, 10.89999999999998259, 3.199999999999997957 ) ) ;
#201724=CARTESIAN_POINT ( 'NONE',  ( -10.95308175811721085, 11.29999999999999893, -1.800000000000001155 ) ) ;
#201761=CARTESIAN_POINT ( 'NONE',  ( 9.573135803333604699, 13.80976963840737248, -8.295511852730781399 ) ) ;
#201779=CARTESIAN_POINT ( 'NONE',  ( 11.94655611907589865, 13.65200944546904083, -1.134828163062138628 ) ) ;
#201791=CARTESIAN_POINT ( 'NONE',  ( -10.60630082101195804, 5.715768461961713953, -4.896526734066639186 ) ) ;
#201810=CARTESIAN_POINT ( 'NONE',  ( 7.185352960343817763, 15.44063983605676604, 9.557346848789475047 ) ) ;
#201815=DIRECTION ( 'NONE',  ( 0.000000000000000000, 0.1994302930878473212, -0.9799120155396071619 ) ) ;
#201817=CARTESIAN_POINT ( 'NONE',  ( 10.35141017034361788, 10.47591664987898241, -5.982769973146199405 ) ) ;
#201831=CARTESIAN_POINT ( 'NONE',  ( 11.80247861663003484, 9.799999999999984723, 1.695431928471866190 ) ) ;
#201840=EDGE_CURVE ( 'NONE', #103541, #95942, #87144, .T. ) ;
#201853=VECTOR ( 'NONE', #196023, 1000.000000000000000 ) ;
#201873=DIRECTION ( 'NONE',  ( 0.000000000000000000, 1.000000000000000000, 0.000000000000000000 ) ) ;
#201874=CARTESIAN_POINT ( 'NONE',  ( -10.79501016327925633, 6.383858692899066156, 5.153711710998491569 ) ) ;
#201918=CARTESIAN_POINT ( 'NONE',  ( -0.02978472384952053284, 15.46795719462065577, 11.98291739243534160 ) ) ;
#201925=PLANE ( 'NONE',  #17305 ) ;
#201940=EDGE_CURVE ( 'NONE', #209056, #198860, #180491, .T. ) ;
#201955=CARTESIAN_POINT ( 'NONE',  ( -11.84668730067608600, 10.19999999999998153, 1.319999999999998286 ) ) ;
#202009=CARTESIAN_POINT ( 'NONE',  ( -11.92619526913699879, 10.89999999999998259, 1.328859060402684644 ) ) ;
#202029=CARTESIAN_POINT ( 'NONE',  ( 0.6674790882332001241, 14.00000000000001066, -11.66566053519550650 ) ) ;
#202031=CARTESIAN_POINT ( 'NONE',  ( -10.50660484223216606, 5.359830900411396648, 5.105327592218940502 ) ) ;
#202048=EDGE_LOOP ( 'NONE', ( #202396, #89104, #178730, #174378 ) ) ;
#202063=CARTESIAN_POINT ( 'NONE',  ( -15.75000000000000000, 13.40000000000000036, -3.600000000000002309 ) ) ;
#202073=PLANE ( 'NONE',  #136111 ) ;
#202109=CARTESIAN_POINT ( 'NONE',  ( -11.04536101718726293, 12.69999999999999929, 1.099999999999996758 ) ) ;
#202127=VERTEX_POINT ( 'NONE', #36828 ) ;
#202133=ORIENTED_EDGE ( 'NONE', *, *, #14440, .F. ) ;
#202140=CARTESIAN_POINT ( 'NONE',  ( -10.74038358936941506, 4.109630040845076770, -4.806702709432750353 ) ) ;
#202141=SURFACE_SIDE_STYLE ('',( #203223 ) ) ;
#202155=VECTOR ( 'NONE', #29097, 1000.000000000000000 ) ;
#202160=CARTESIAN_POINT ( 'NONE',  ( 12.00010711203362312, 6.624312021734491296, -0.4953576099243469089 ) ) ;
#202169=ORIENTED_EDGE ( 'NONE', *, *, #129583, .T. ) ;
#202172=CARTESIAN_POINT ( 'NONE',  ( 12.19178133996304148, 6.204039751267350411, 2.192769013902648112 ) ) ;
#202184=CARTESIAN_POINT ( 'NONE',  ( -4.363504500571202982, 15.44735459669111854, -11.13999821485972674 ) ) ;
#202188=DIRECTION ( 'NONE',  ( 6.938893903907222067E-15, 1.000000000000000000, 0.000000000000000000 ) ) ;
#202203=EDGE_CURVE ( 'NONE', #135251, #18531, #127426, .T. ) ;
#202216=CARTESIAN_POINT ( 'NONE',  ( -9.523271317088290999, 14.62225410442589002, -7.301265812034692715 ) ) ;
#202225=B_SPLINE_CURVE_WITH_KNOTS ( 'NONE', 3,
 ( #35949, #85774, #182191, #149715, #151855, #67353 ),
 .UNSPECIFIED., .F., .F.,
 ( 4, 2, 4 ),
 ( 0.000000000000000000, 0.0003258677429877276867, 0.0006517354859754553734 ),
 .UNSPECIFIED. ) ;
#202238=ORIENTED_EDGE ( 'NONE', *, *, #59260, .T. ) ;
#202242=EDGE_CURVE ( 'NONE', #121570, #45318, #40924, .T. ) ;
#202247=B_SPLINE_CURVE_WITH_KNOTS ( 'NONE', 3,
 ( #27293, #146075, #98365, #149243, #131969, #84242 ),
 .UNSPECIFIED., .F., .F.,
 ( 4, 2, 4 ),
 ( 0.000000000000000000, 0.0003132070624402877746, 0.0006264141248805755492 ),
 .UNSPECIFIED. ) ;
#202284=( BOUNDED_SURFACE ( )  B_SPLINE_SURFACE ( 3, 2, ( 
 ( #64677, #92949, #193616 ),
 ( #158995, #76665, #97211 ),
 ( #78790, #142779, #208785 ),
 ( #96149, #60415, #79861 ),
 ( #95080, #31136, #27923 ),
 ( #179517, #210920, #147026 ),
 ( #61487, #45257, #163263 ),
 ( #192536, #94018, #175260 ),
 ( #110310, #211982, #191471 ),
 ( #111376, #11661, #213049 ),
 ( #14845, #176318, #43138 ),
 ( #77734, #143856, #26845 ),
 ( #44190, #145970, #209848 ),
 ( #127652, #63622, #80935 ),
 ( #177380, #161129, #144913 ),
 ( #62546, #128709, #194678 ) ),
 .UNSPECIFIED., .F., .F., .T. ) 
 B_SPLINE_SURFACE_WITH_KNOTS ( ( 4, 2, 2, 2, 2, 2, 2, 4 ),
 ( 3, 3 ),
 ( -3.469446951953614189E-18, 0.0005295610108084591698, 0.001059122021616921809, 0.001588683032425384448, 0.002118244043233847088, 0.002647805054042309727, 0.003177366064850772366, 0.004236488086467697645 ),
 ( 0.000000000000000000, 1.000000000000000000 ),
 .UNSPECIFIED. ) 
 GEOMETRIC_REPRESENTATION_ITEM ( )  RATIONAL_B_SPLINE_SURFACE ( (
 ( 1.000000000000000000, 0.8434758251109465421, 1.000000000000000000),
 ( 1.000000000000000000, 0.8438484666245520405, 1.000000000000000000),
 ( 1.000000000000000000, 0.8442947513603508147, 1.000000000000000000),
 ( 1.000000000000000000, 0.8452199691704415097, 1.000000000000000000),
 ( 1.000000000000000000, 0.8457194463841322118, 1.000000000000000000),
 ( 1.000000000000000000, 0.8468087058708519965, 1.000000000000000000),
 ( 1.000000000000000000, 0.8474271749261985676, 1.000000000000000000),
 ( 1.000000000000000000, 0.8486845056840492951, 1.000000000000000000),
 ( 1.000000000000000000, 0.8493328185060563529, 1.000000000000000000),
 ( 1.000000000000000000, 0.8502002772864952762, 1.000000000000000000),
 ( 1.000000000000000000, 0.8502729042284375982, 1.000000000000000000),
 ( 1.000000000000000000, 0.8504148911931121990, 1.000000000000000000),
 ( 1.000000000000000000, 0.8504126782990119038, 1.000000000000000000),
 ( 1.000000000000000000, 0.8505517453013814455, 1.000000000000000000),
 ( 1.000000000000000000, 0.8508995438024010705, 1.000000000000000000),
 ( 1.000000000000000000, 0.8509629433967770273, 1.000000000000000000) ) ) 
 REPRESENTATION_ITEM ( '' )  SURFACE ( )  );
#202290=ORIENTED_EDGE ( 'NONE', *, *, #206026, .F. ) ;
#202295=CARTESIAN_POINT ( 'NONE',  ( 0.000000000000000000, 0.08000000000000020983, 0.000000000000000000 ) ) ;
#202309=VECTOR ( 'NONE', #199002, 1000.000000000000000 ) ;
#202316=B_SPLINE_CURVE_WITH_KNOTS ( 'NONE', 3,
 ( #85928, #135756, #116351, #201779, #119556, #16636 ),
 .UNSPECIFIED., .F., .F.,
 ( 4, 2, 4 ),
 ( 0.000000000000000000, 0.0003767643964918269734, 0.0007535287929836536214 ),
 .UNSPECIFIED. ) ;
#202332=UNCERTAINTY_MEASURE_WITH_UNIT (LENGTH_MEASURE( 1.000000000000000082E-05 ), #130101, 'distance_accuracy_value', 'NONE');
#202348=FACE_OUTER_BOUND ( 'NONE', #117249, .T. ) ;
#202351=( GEOMETRIC_REPRESENTATION_CONTEXT ( 3 ) GLOBAL_UNCERTAINTY_ASSIGNED_CONTEXT ( ( #49652 ) ) GLOBAL_UNIT_ASSIGNED_CONTEXT ( ( #51684, #1821, #88455 ) ) REPRESENTATION_CONTEXT ( 'NONE', 'WORKASPACE' ) );
#202396=ORIENTED_EDGE ( 'NONE', *, *, #89006, .T. ) ;
#202459=DIRECTION ( 'NONE',  ( 0.000000000000000000, 1.000000000000000000, 0.000000000000000000 ) ) ;
#202473=SURFACE_STYLE_FILL_AREA ( #105023 ) ;
#202478=DIRECTION ( 'NONE',  ( 0.9982742078614211811, 0.000000000000000000, 0.05872483221476467591 ) ) ;
#202497=EDGE_CURVE ( 'NONE', #48843, #51477, #102580, .T. ) ;
#202504=DIRECTION ( 'NONE',  ( -0.9632918427306580433, 0.000000000000000000, -0.2684563758389303945 ) ) ;
#202512=SURFACE_STYLE_USAGE ( .BOTH. , #199316 ) ;
#202520=FACE_OUTER_BOUND ( 'NONE', #188887, .T. ) ;
#202539=ORIENTED_EDGE ( 'NONE', *, *, #70476, .F. ) ;
#202580=CARTESIAN_POINT ( 'NONE',  ( -11.76695491367977198, 4.673720869072629291, 4.995412848167409159 ) ) ;
#202610=ADVANCED_FACE ( 'NONE', ( #58678 ), #94402, .F. ) ;
#202613=DIRECTION ( 'NONE',  ( 0.000000000000000000, 0.000000000000000000, 1.000000000000000000 ) ) ;
#202616=VECTOR ( 'NONE', #124684, 1000.000000000000000 ) ;
#202641=CARTESIAN_POINT ( 'NONE',  ( -10.06283597805679975, 4.651455381798285771, -6.539173949727397961 ) ) ;
#202647=CARTESIAN_POINT ( 'NONE',  ( 11.89942855770814312, 13.79999999999999893, 0.6999999999999992895 ) ) ;
#202667=( GEOMETRIC_REPRESENTATION_CONTEXT ( 3 ) GLOBAL_UNCERTAINTY_ASSIGNED_CONTEXT ( ( #77635 ) ) GLOBAL_UNIT_ASSIGNED_CONTEXT ( ( #87687, #69277, #153761 ) ) REPRESENTATION_CONTEXT ( 'NONE', 'WORKASPACE' ) );
#202669=ORIENTED_EDGE ( 'NONE', *, *, #28369, .F. ) ;
#202679=VECTOR ( 'NONE', #22918, 1000.000000000000000 ) ;
#202700=SURFACE_STYLE_USAGE ( .BOTH. , #170218 ) ;
#202705=ORIENTED_EDGE ( 'NONE', *, *, #156690, .F. ) ;
#202720=ADVANCED_FACE ( 'NONE', ( #145302 ), #20002, .T. ) ;
#202735=ORIENTED_EDGE ( 'NONE', *, *, #177319, .F. ) ;
#202736=LINE ( 'NONE', #104207, #202679 ) ;
#202741=EDGE_CURVE ( 'NONE', #142717, #200044, #190420, .T. ) ;
#202745=CARTESIAN_POINT ( 'NONE',  ( 11.88234649872613602, 12.34339217083249096, -0.9090484974825243647 ) ) ;
#202759=COLOUR_RGB ( '', 0.72549020, 0.75294118, 0.79215686) ;
#202767=EDGE_LOOP ( 'NONE', ( #42118, #43895, #44007, #127672 ) ) ;
#202783=CARTESIAN_POINT ( 'NONE',  ( 11.04536101718726293, 12.69999999999999929, 1.099999999999996758 ) ) ;
#202787=DIRECTION ( 'NONE',  ( -0.9632918427306580433, 0.000000000000000000, 0.2684563758389303945 ) ) ;
#202792=DIRECTION ( 'NONE',  ( 0.9885327375000381167, 0.000000000000000000, -0.1510067114093955609 ) ) ;
#202798=STYLED_ITEM ( 'NONE', ( #74865 ), #98352 ) ;
#202830=CARTESIAN_POINT ( 'NONE',  ( 8.312826421212609063, 13.22328045796207086, -8.547122492678219885 ) ) ;
#202836=ORIENTED_EDGE ( 'NONE', *, *, #23138, .T. ) ;
#202863=CARTESIAN_POINT ( 'NONE',  ( 7.853188201116851452, 15.31763947413069715, -9.016399092843794705 ) ) ;
#202879=CARTESIAN_POINT ( 'NONE',  ( 8.944921657900962941, 14.55297637781186637, 7.932298026445150363 ) ) ;
#202884=SURFACE_STYLE_USAGE ( .BOTH. , #136860 ) ;
#202907=CARTESIAN_POINT ( 'NONE',  ( 6.928203230275522095, 15.51887838114830132, 9.797958971132704420 ) ) ;
#202920=CARTESIAN_POINT ( 'NONE',  ( -11.86239285000045918, 11.37999999999998302, 1.812080536912751061 ) ) ;
#202924=STYLED_ITEM ( 'NONE', ( #61112 ), #196848 ) ;
#202948=CARTESIAN_POINT ( 'NONE',  ( 9.243516698675458443, 13.40993305631030985, 7.925370479070547702 ) ) ;
#202962=AXIS2_PLACEMENT_3D ( 'NONE', #149330, #133116, #199114 ) ;
#202967=SURFACE_STYLE_USAGE ( .BOTH. , #100159 ) ;
#202985=EDGE_LOOP ( 'NONE', ( #117304, #68259, #48884, #56770 ) ) ;
#202990=EDGE_CURVE ( 'NONE', #67257, #143616, #166841, .T. ) ;
#203004=CARTESIAN_POINT ( 'NONE',  ( -10.64364919647040786, 5.928722196471193584, -5.549781512408035411 ) ) ;
#203005=FILL_AREA_STYLE_COLOUR ( '', #156337 ) ;
#203041=DIRECTION ( 'NONE',  ( -7.993605777301127091E-15, 0.000000000000000000, 1.000000000000000000 ) ) ;
#203063=CARTESIAN_POINT ( 'NONE',  ( -10.95308175811721085, 13.79999999999999893, -1.800000000000001155 ) ) ;
#203071=DIRECTION ( 'NONE',  ( 0.000000000000000000, -1.000000000000000000, 0.000000000000000000 ) ) ;
#203084=UNCERTAINTY_MEASURE_WITH_UNIT (LENGTH_MEASURE( 1.000000000000000082E-05 ), #160485, 'distance_accuracy_value', 'NONE');
#203085=DIRECTION ( 'NONE',  ( 0.5994789404140898892, -1.444427003850258927E-16, 0.8003905296791063995 ) ) ;
#203112=CARTESIAN_POINT ( 'NONE',  ( -10.84558554699185784, 5.653278704827924273, 6.476092148523931336 ) ) ;
#203116=ADVANCED_FACE ( 'NONE', ( #212366 ), #113902, .T. ) ;
#203123=CARTESIAN_POINT ( 'NONE',  ( 10.97011102005664185, 11.29999999999997939, 1.696376167609456198 ) ) ;
#203139=ORIENTED_EDGE ( 'NONE', *, *, #130231, .T. ) ;
#203147=CARTESIAN_POINT ( 'NONE',  ( 0.000000000000000000, 11.37999999999999901, 0.000000000000000000 ) ) ;
#203157=( NAMED_UNIT ( * ) SI_UNIT ( $, .STERADIAN. ) SOLID_ANGLE_UNIT ( ) );
#203222=CARTESIAN_POINT ( 'NONE',  ( -11.25771003949915539, 3.534410846742664702, -5.930344140359695260 ) ) ;
#203223=SURFACE_STYLE_FILL_AREA ( #52722 ) ;
#203232=CARTESIAN_POINT ( 'NONE',  ( -10.47476631618627252, 5.237304525980054137, 5.169966676860812349 ) ) ;
#203238=CARTESIAN_POINT ( 'NONE',  ( 11.35349642860619390, 7.539003845593507336, 3.753059129874396493 ) ) ;
#203261=CARTESIAN_POINT ( 'NONE',  ( -9.333041836229160282, 15.44694763439141205, -7.472413793097630652 ) ) ;
#203265=DIRECTION ( 'NONE',  ( 0.000000000000000000, 7.228014483236694583E-17, -1.000000000000000000 ) ) ;
#203276=ADVANCED_FACE ( 'NONE', ( #66099 ), #61608, .T. ) ;
#203300=CARTESIAN_POINT ( 'NONE',  ( 11.89942855770814312, 13.79999999999999893, -0.7000000000000009548 ) ) ;
#203304=CARTESIAN_POINT ( 'NONE',  ( -10.41986968326957808, 5.020773655391575829, -5.279272669861445166 ) ) ;
#203320=ORIENTED_EDGE ( 'NONE', *, *, #163044, .F. ) ;
#203343=ADVANCED_FACE ( 'NONE', ( #89873 ), #130204, .T. ) ;
#203350=EDGE_CURVE ( 'NONE', #48473, #144017, #186069, .T. ) ;
#203360=EDGE_LOOP ( 'NONE', ( #28202, #189927, #46405, #185662 ) ) ;
#203406=STYLED_ITEM ( 'NONE', ( #63680 ), #105592 ) ;
#203436=CARTESIAN_POINT ( 'NONE',  ( 9.681421036508346845, 3.864712292056655230, -7.090140105714071161 ) ) ;
#203460=CARTESIAN_POINT ( 'NONE',  ( -9.361980464089038279, 15.42898634278301628, -7.422930886903965408 ) ) ;
#203483=CARTESIAN_POINT ( 'NONE',  ( -11.86239285000045918, 9.719999999999982876, 1.812080536912751283 ) ) ;
#203495=VERTEX_POINT ( 'NONE', #206787 ) ;
#203499=CARTESIAN_POINT ( 'NONE',  ( -9.348561386651960348, 4.000000000000000888, 7.001914024036569373 ) ) ;
#203505=CIRCLE ( 'NONE', #6534, 0.07999999999999998779 ) ;
#203510=ORIENTED_EDGE ( 'NONE', *, *, #150811, .T. ) ;
#203521=CARTESIAN_POINT ( 'NONE',  ( 11.33772463945036790, 13.40000000000000036, -3.600000000000002309 ) ) ;
#203530=ORIENTED_EDGE ( 'NONE', *, *, #72282, .T. ) ;
#203546=( NAMED_UNIT ( * ) PLANE_ANGLE_UNIT ( ) SI_UNIT ( $, .RADIAN. ) );
#203578=DIRECTION ( 'NONE',  ( 0.000000000000000000, -0.000000000000000000, 1.000000000000000000 ) ) ;
#203579=CARTESIAN_POINT ( 'NONE',  ( -11.04536101718726293, 10.90000000000000036, 1.099999999999996758 ) ) ;
#203598=CARTESIAN_POINT ( 'NONE',  ( -4.767738813365186346, 15.46911576196198901, 11.02133430360666644 ) ) ;
#203611=CARTESIAN_POINT ( 'NONE',  ( -10.97011102005664185, 9.799999999999982947, 1.696376167609455310 ) ) ;
#203646=CARTESIAN_POINT ( 'NONE',  ( -10.97061778408437505, 3.255139717175850933, 6.407648009301818881 ) ) ;
#203664=( GEOMETRIC_REPRESENTATION_CONTEXT ( 3 ) GLOBAL_UNCERTAINTY_ASSIGNED_CONTEXT ( ( #135217 ) ) GLOBAL_UNIT_ASSIGNED_CONTEXT ( ( #89600, #108033, #90666 ) ) REPRESENTATION_CONTEXT ( 'NONE', 'WORKASPACE' ) );
#203666=ORIENTED_EDGE ( 'NONE', *, *, #197814, .T. ) ;
#203677=CARTESIAN_POINT ( 'NONE',  ( -9.523545778475458690, 14.62276350342200359, -7.300907474435643252 ) ) ;
#203686=ADVANCED_FACE ( 'NONE', ( #25899 ), #32063, .T. ) ;
#203699=CARTESIAN_POINT ( 'NONE',  ( -10.10413230197131540, 3.643845688154880857, -6.474695611014302798 ) ) ;
#203768=ORIENTED_EDGE ( 'NONE', *, *, #118985, .F. ) ;
#203784=CARTESIAN_POINT ( 'NONE',  ( -11.83256397649420677, 7.177290438377375459, -1.867481893931521419 ) ) ;
#203785=CARTESIAN_POINT ( 'NONE',  ( 0.000000000000000000, 12.22000000000000064, 0.000000000000000000 ) ) ;
#203788=CARTESIAN_POINT ( 'NONE',  ( 11.89197415570408900, 12.30000000000000071, -0.8055989572471863314 ) ) ;
#203809=ORIENTED_EDGE ( 'NONE', *, *, #78727, .F. ) ;
#203813=FACE_OUTER_BOUND ( 'NONE', #77433, .T. ) ;
#203836=DIRECTION ( 'NONE',  ( -0.000000000000000000, 1.000000000000000000, -0.000000000000000000 ) ) ;
#203843=EDGE_CURVE ( 'NONE', #141526, #185203, #35499, .T. ) ;
#203844=ORIENTED_EDGE ( 'NONE', *, *, #186883, .F. ) ;
#203849=CARTESIAN_POINT ( 'NONE',  ( 11.06297021485807264, 12.34330698512527569, 0.9089447062504968367 ) ) ;
#203865=B_SPLINE_CURVE_WITH_KNOTS ( 'NONE', 3,
 ( #176074, #114079, #66272, #213595, #180070, #212548, #125263, #47963, #32743, #16469, #159806, #31694, #42887 ),
 .UNSPECIFIED., .F., .F.,
 ( 4, 3, 3, 3, 4 ),
 ( 1.011944969444384544E-17, 3.127682647416726467E-05, 7.184504844521671105E-05, 0.0001122487170298541655, 0.0001140435926658500367 ),
 .UNSPECIFIED. ) ;
#203915=CARTESIAN_POINT ( 'NONE',  ( 10.56514123924917392, 12.34108045521194263, -3.404988257269842222 ) ) ;
#203946=ORIENTED_EDGE ( 'NONE', *, *, #205068, .T. ) ;
#203956=CARTESIAN_POINT ( 'NONE',  ( 0.000000000000000000, 9.799999999999998934, 0.000000000000000000 ) ) ;
#203982=EDGE_CURVE ( 'NONE', #97098, #205382, #189784, .T. ) ;
#203988=DIRECTION ( 'NONE',  ( 0.000000000000000000, -1.000000000000000000, 0.000000000000000000 ) ) ;
#204023=CARTESIAN_POINT ( 'NONE',  ( 11.86145016429273191, 12.69999999999999929, -1.180000000000000604 ) ) ;
#204036=CARTESIAN_POINT ( 'NONE',  ( -8.784791485860443672, 14.48107303905707255, -8.187053764137555589 ) ) ;
#204047=CARTESIAN_POINT ( 'NONE',  ( 9.452508394161709404, 3.481540833006149249, -7.393820799723212822 ) ) ;
#204057=CARTESIAN_POINT ( 'NONE',  ( -11.15646993939951059, 7.316272439152442963, -4.426198049908277810 ) ) ;
#204060=EDGE_CURVE ( 'NONE', #125323, #177320, #120606, .T. ) ;
#204119=CARTESIAN_POINT ( 'NONE',  ( -10.97031310326519282, 13.80000000000000071, -1.695146482106561381 ) ) ;
#204133=CARTESIAN_POINT ( 'NONE',  ( -11.88168509644349058, 13.87999999999999901, -1.685788023084331400 ) ) ;
#204153=CARTESIAN_POINT ( 'NONE',  ( 11.97302537858640115, 9.801240101919827197, 0.8111997896468206015 ) ) ;
#204166=CARTESIAN_POINT ( 'NONE',  ( -11.43653507270588499, 5.655220009861049668, 5.468867579827167980 ) ) ;
#204174=CARTESIAN_POINT ( 'NONE',  ( 10.98546401119367566, 11.25740562920347365, 1.592223900679732518 ) ) ;
#204177=B_SPLINE_CURVE_WITH_KNOTS ( 'NONE', 3,
 ( #151681, #82393, #83458, #149538, #168979, #1124 ),
 .UNSPECIFIED., .F., .F.,
 ( 4, 2, 4 ),
 ( 0.000000000000000000, 0.0003844267940947826011, 0.0007688535881895652022 ),
 .UNSPECIFIED. ) ;
#204197=DIRECTION ( 'NONE',  ( 0.000000000000000000, 0.000000000000000000, -1.000000000000000000 ) ) ;
#204209=DIRECTION ( 'NONE',  ( 0.000000000000000000, -0.000000000000000000, 1.000000000000000000 ) ) ;
#204232=DIRECTION ( 'NONE',  ( 0.000000000000000000, -1.000000000000000000, 0.000000000000000000 ) ) ;
#204233=LINE ( 'NONE', #24428, #179298 ) ;
#204246=CARTESIAN_POINT ( 'NONE',  ( 11.94105721237523277, 10.19999999999999929, 1.187919463087244720 ) ) ;
#204277=CARTESIAN_POINT ( 'NONE',  ( -11.30309668167796922, 5.150585336095395483, -5.742054036728553967 ) ) ;
#204287=CARTESIAN_POINT ( 'NONE',  ( -10.01593736600300311, 5.734280347462529015, 5.906528988732270058 ) ) ;
#204291=ORIENTED_EDGE ( 'NONE', *, *, #210514, .F. ) ;
#204294=CARTESIAN_POINT ( 'NONE',  ( 8.776224899084628106, 13.27471476138783224, 8.184001253707569035 ) ) ;
#204306=DIRECTION ( 'NONE',  ( 0.000000000000000000, 1.000000000000000000, 0.000000000000000000 ) ) ;
#204332=EDGE_CURVE ( 'NONE', #129544, #93441, #7255, .T. ) ;
#204338=VERTEX_POINT ( 'NONE', #43010 ) ;
#204360=( NAMED_UNIT ( * ) SI_UNIT ( $, .STERADIAN. ) SOLID_ANGLE_UNIT ( ) );
#204364=CARTESIAN_POINT ( 'NONE',  ( -9.968662085647130411, 5.546348307810219147, -6.001034872913991514 ) ) ;
#204371=ORIENTED_EDGE ( 'NONE', *, *, #97999, .T. ) ;
#204381=DIRECTION ( 'NONE',  ( 0.000000000000000000, 0.000000000000000000, 1.000000000000000000 ) ) ;
#204391=DIRECTION ( 'NONE',  ( 1.000000000000000000, -0.000000000000000000, -0.000000000000000000 ) ) ;
#204424=VERTEX_POINT ( 'NONE', #47878 ) ;
#204429=AXIS2_PLACEMENT_3D ( 'NONE', #89749, #121242, #154730 ) ;
#204450=ORIENTED_EDGE ( 'NONE', *, *, #117680, .T. ) ;
#204454=ORIENTED_EDGE ( 'NONE', *, *, #59437, .T. ) ;
#204496=FILL_AREA_STYLE ('',( #138474 ) ) ;
#204528=LINE ( 'NONE', #108198, #936 ) ;
#204568=CARTESIAN_POINT ( 'NONE',  ( 1.734723475976807094E-15, 14.56776713488954655, 11.92913357381758388 ) ) ;
#204569=DIRECTION ( 'NONE',  ( 0.000000000000000000, -0.000000000000000000, 1.000000000000000000 ) ) ;
#204570=CARTESIAN_POINT ( 'NONE',  ( -10.78913822082115281, 5.463154562124156399, 6.589184675844935057 ) ) ;
#204597=CARTESIAN_POINT ( 'NONE',  ( -4.933501523973760072E-10, 15.51845925587262798, -12.00000000000000178 ) ) ;
#204598=CARTESIAN_POINT ( 'NONE',  ( -6.755468634461358590, 14.48046873815656177, 9.927994241953896903 ) ) ;
#204600=ORIENTED_EDGE ( 'NONE', *, *, #39272, .F. ) ;
#204673=CARTESIAN_POINT ( 'NONE',  ( 0.000000000000000000, 9.719999999999982876, 0.000000000000000000 ) ) ;
#204681=CARTESIAN_POINT ( 'NONE',  ( 10.65531535955785536, 9.862547934939467353, 5.420879958757526929 ) ) ;
#204683=AXIS2_PLACEMENT_3D ( 'NONE', #184079, #69243, #70308 ) ;
#204692=ORIENTED_EDGE ( 'NONE', *, *, #120407, .T. ) ;
#204711=CARTESIAN_POINT ( 'NONE',  ( -11.38450596090590849, 3.710255710271473273, 5.708599601896569453 ) ) ;
#204726=LINE ( 'NONE', #7602, #62650 ) ;
#204735=CARTESIAN_POINT ( 'NONE',  ( 1.734723475976807094E-15, 15.43265149481033305, 11.92913362508773822 ) ) ;
#204753=FACE_OUTER_BOUND ( 'NONE', #174875, .T. ) ;
#204762=CARTESIAN_POINT ( 'NONE',  ( -9.367496997750912158, 14.48154074412965997, 7.499999999808506068 ) ) ;
#204795=DIRECTION ( 'NONE',  ( -1.000000000000000000, -2.210062264950106756E-32, 1.224646799147353207E-16 ) ) ;
#204806=VERTEX_POINT ( 'NONE', #202109 ) ;
#204834=( BOUNDED_SURFACE ( )  B_SPLINE_SURFACE ( 3, 2, ( 
 ( #89192, #140084, #41508 ),
 ( #208237, #56677, #7901 ),
 ( #188802, #24148, #27364 ),
 ( #8982, #123898, #75057 ),
 ( #155243, #6825, #93465 ),
 ( #141170, #72905, #139009 ),
 ( #205031, #122841, #172565 ),
 ( #173653, #175771, #90251 ),
 ( #109763, #207179, #77178 ),
 ( #40439, #121757, #105449 ),
 ( #209291, #159505, #11102 ),
 ( #73990, #42584, #106540 ),
 ( #156318, #143300, #187725 ),
 ( #206108, #58804, #39353 ) ),
 .UNSPECIFIED., .F., .F., .F. ) 
 B_SPLINE_SURFACE_WITH_KNOTS ( ( 4, 2, 2, 2, 2, 2, 4 ),
 ( 3, 3 ),
 ( -6.505213034913026604E-19, 0.002680181519792705202, 0.004020272279689058453, 0.005360363039585411271, 0.006700453799481764089, 0.008040544559378116907, 0.01072072607917082254 ),
 ( 0.000000000000000000, 1.000000000000000000 ),
 .UNSPECIFIED. ) 
 GEOMETRIC_REPRESENTATION_ITEM ( )  RATIONAL_B_SPLINE_SURFACE ( (
 ( 1.000000000000000000, 0.8509629433892340611, 1.000000000000000000),
 ( 1.000000000000000000, 0.8507311530181393966, 1.000000000000000000),
 ( 1.000000000000000000, 0.8494583134163782301, 1.000000000000000000),
 ( 1.000000000000000000, 0.8495296534838289171, 1.000000000000000000),
 ( 1.000000000000000000, 0.8498242239227816741, 1.000000000000000000),
 ( 1.000000000000000000, 0.8505549521784944167, 1.000000000000000000),
 ( 1.000000000000000000, 0.8509834526754082029, 1.000000000000000000),
 ( 1.000000000000000000, 0.8509410435525731620, 1.000000000000000000),
 ( 1.000000000000000000, 0.8504680959802140006, 1.000000000000000000),
 ( 1.000000000000000000, 0.8496964069595507318, 1.000000000000000000),
 ( 1.000000000000000000, 0.8493987049676730017, 1.000000000000000000),
 ( 1.000000000000000000, 0.8493809005009217428, 1.000000000000000000),
 ( 1.000000000000000000, 0.8507510709369977553, 1.000000000000000000),
 ( 1.000000000000000000, 0.8509629433967522694, 1.000000000000000000) ) ) 
 REPRESENTATION_ITEM ( '' )  SURFACE ( )  );
#204847=CARTESIAN_POINT ( 'NONE',  ( -11.14501278000869355, 7.223412960316487386, -3.546411330735405265 ) ) ;
#204859=EDGE_CURVE ( 'NONE', #125687, #83422, #168908, .T. ) ;
#204864=ORIENTED_EDGE ( 'NONE', *, *, #59542, .T. ) ;
#204916=PRESENTATION_STYLE_ASSIGNMENT (( #40327 ) ) ;
#204921=SURFACE_SIDE_STYLE ('',( #41408 ) ) ;
#204948=AXIS2_PLACEMENT_3D ( 'NONE', #945, #36664, #102751 ) ;
#204964=CARTESIAN_POINT ( 'NONE',  ( 9.397486876216094132, 13.53113053364065443, 7.462549781540788629 ) ) ;
#204969=CARTESIAN_POINT ( 'NONE',  ( -11.86687934130374167, 12.49048050383441577, -1.056332641424308827 ) ) ;
#204976=UNCERTAINTY_MEASURE_WITH_UNIT (LENGTH_MEASURE( 1.000000000000000082E-05 ), #111538, 'distance_accuracy_value', 'NONE');
#204988=VERTEX_POINT ( 'NONE', #119902 ) ;
#205011=CARTESIAN_POINT ( 'NONE',  ( -10.56199358538776778, 4.161122272433269487, 5.602120407118017731 ) ) ;
#205018=( NAMED_UNIT ( * ) PLANE_ANGLE_UNIT ( ) SI_UNIT ( $, .RADIAN. ) );
#205024=( BOUNDED_SURFACE ( )  B_SPLINE_SURFACE ( 3, 3, ( 
 ( #68318, #127312, #198323, #116081, #48907, #19583, #210595, #98720, #18514, #150680, #182072, #99781, #177042, #82448, #35834, #165846 ),
 ( #134449, #3312, #164779, #200452, #193282, #83515, #101912, #85655, #44927, #151742, #111035, #94744, #120370, #91014, #201512, #71517 ),
 ( #189552, #36898, #72593, #154932, #4373, #102980, #157076, #137629, #88879, #5438, #187416, #41199, #169038, #40117, #20635, #107306 ),
 ( #86724, #186345, #185275, #152793, #188487, #39047, #105132, #22762, #6517, #70443, #24908, #89949, #37980, #56361, #119289, #23841 ),
 ( #171172, #136559, #121447, #69382, #173330, #57426, #203646, #138694, #204711, #104053, #139770, #170099, #21685, #122524, #135490, #202580 ),
 ( #106228, #172254, #87795, #123588, #155999, #205796, #53160, #7586, #54232, #153869, #55297, #73671, #78999, #108377, #28124, #12919 ),
 ( #44391, #144058, #46523, #60618, #158141, #95287, #206861, #125708, #11859, #9732, #145115, #75807, #94218, #211121, #178654, #176512 ) ),
 .UNSPECIFIED., .T., .F., .T. ) 
 B_SPLINE_SURFACE_WITH_KNOTS ( ( 4, 3, 4 ),
 ( 4, 2, 2, 2, 2, 2, 2, 4 ),
 ( 0.000000000000000000, 0.5000000000000000000, 1.000000000000000000 ),
 ( 0.3501333200791456046, 0.3551713324458994903, 0.3602093448126533759, 0.3702853695461611472, 0.3803518226137216351, 0.3853850491475018791, 0.3879016624143920011, 0.3904182756812821231 ),
 .UNSPECIFIED. ) 
 GEOMETRIC_REPRESENTATION_ITEM ( )  RATIONAL_B_SPLINE_SURFACE ( (
 ( 1.000000000000000000, 1.000000000000000000, 1.000000000000000000, 1.000000000000000000, 1.000000000000000000, 1.000000000000000000, 1.000000000000000000, 1.000000000000000000, 1.000000000000000000, 1.000000000000000000, 1.000000000000000000, 1.000000000000000000, 1.000000000000000000, 1.000000000000000000, 1.000000000000000000, 1.000000000000000000),
 ( 0.3333333333333333703, 0.3333333333333333703, 0.3333333333333333703, 0.3333333333333333703, 0.3333333333333333703, 0.3333333333333333703, 0.3333333333333333703, 0.3333333333333333703, 0.3333333333333333703, 0.3333333333333333703, 0.3333333333333333703, 0.3333333333333333703, 0.3333333333333333703, 0.3333333333333333703, 0.3333333333333333703, 0.3333333333333333703),
 ( 0.3333333333333333703, 0.3333333333333333703, 0.3333333333333333703, 0.3333333333333333703, 0.3333333333333333703, 0.3333333333333333703, 0.3333333333333333703, 0.3333333333333333703, 0.3333333333333333703, 0.3333333333333333703, 0.3333333333333333703, 0.3333333333333333703, 0.3333333333333333703, 0.3333333333333333703, 0.3333333333333333703, 0.3333333333333333703),
 ( 1.000000000000000000, 1.000000000000000000, 1.000000000000000000, 1.000000000000000000, 1.000000000000000000, 1.000000000000000000, 1.000000000000000000, 1.000000000000000000, 1.000000000000000000, 1.000000000000000000, 1.000000000000000000, 1.000000000000000000, 1.000000000000000000, 1.000000000000000000, 1.000000000000000000, 1.000000000000000000),
 ( 0.3333333333333333703, 0.3333333333333333703, 0.3333333333333333703, 0.3333333333333333703, 0.3333333333333333703, 0.3333333333333333703, 0.3333333333333333703, 0.3333333333333333703, 0.3333333333333333703, 0.3333333333333333703, 0.3333333333333333703, 0.3333333333333333703, 0.3333333333333333703, 0.3333333333333333703, 0.3333333333333333703, 0.3333333333333333703),
 ( 0.3333333333333333703, 0.3333333333333333703, 0.3333333333333333703, 0.3333333333333333703, 0.3333333333333333703, 0.3333333333333333703, 0.3333333333333333703, 0.3333333333333333703, 0.3333333333333333703, 0.3333333333333333703, 0.3333333333333333703, 0.3333333333333333703, 0.3333333333333333703, 0.3333333333333333703, 0.3333333333333333703, 0.3333333333333333703),
 ( 1.000000000000000000, 1.000000000000000000, 1.000000000000000000, 1.000000000000000000, 1.000000000000000000, 1.000000000000000000, 1.000000000000000000, 1.000000000000000000, 1.000000000000000000, 1.000000000000000000, 1.000000000000000000, 1.000000000000000000, 1.000000000000000000, 1.000000000000000000, 1.000000000000000000, 1.000000000000000000) ) ) 
 REPRESENTATION_ITEM ( '' )  SURFACE ( )  );
#205026=CARTESIAN_POINT ( 'NONE',  ( -10.57232898948313604, 5.599354254162436817, 4.968808419985093039 ) ) ;
#205031=CARTESIAN_POINT ( 'NONE',  ( -5.580962959613590790, 14.55306900392666947, -10.58267955529689175 ) ) ;
#205036=CARTESIAN_POINT ( 'NONE',  ( -9.305047017617296135, 14.48154074412967596, 7.449999999995404742 ) ) ;
#205041=COLOUR_RGB ( '', 0.66274510, 0.83137255, 0.94901961) ;
#205068=EDGE_CURVE ( 'NONE', #193462, #45616, #161664, .T. ) ;
#205078=CARTESIAN_POINT ( 'NONE',  ( -11.96209379583854293, 12.27207059405763445, 0.9572398070798600056 ) ) ;
#205090=DIRECTION ( 'NONE',  ( -0.1959617823641899015, 0.8823239620903393643, -0.4279058375085054156 ) ) ;
#205104=DIRECTION ( 'NONE',  ( 0.000000000000000000, 0.000000000000000000, -1.000000000000000000 ) ) ;
#205118=CARTESIAN_POINT ( 'NONE',  ( -11.44800751629991353, 9.799999999999998934, -3.302956944461114652 ) ) ;
#205138=CARTESIAN_POINT ( 'NONE',  ( -11.90498647923048914, 8.894293214940326209, 1.536019656081360152 ) ) ;
#205156=EDGE_CURVE ( 'NONE', #149901, #208182, #171782, .T. ) ;
#205164=CARTESIAN_POINT ( 'NONE',  ( -11.33772463945036968, 12.69999999999999929, -3.680000000000002824 ) ) ;
#205186=ORIENTED_EDGE ( 'NONE', *, *, #17565, .T. ) ;
#205200=CARTESIAN_POINT ( 'NONE',  ( -15.75000000000000000, 11.29999999999998117, 3.199999999999997957 ) ) ;
#205203=FILL_AREA_STYLE_COLOUR ( '', #106205 ) ;
#205217=CARTESIAN_POINT ( 'NONE',  ( -11.92619526913700057, 13.52781666661243243, -1.328859060402685976 ) ) ;
#205237=CARTESIAN_POINT ( 'NONE',  ( 11.89942855770814312, 9.799999999999998934, 0.6999999999999992895 ) ) ;
#205250=CARTESIAN_POINT ( 'NONE',  ( -10.99298880388840338, 6.209297407268072888, -6.173882299569079635 ) ) ;
#205261=ORIENTED_EDGE ( 'NONE', *, *, #171086, .T. ) ;
#205294=PRESENTATION_STYLE_ASSIGNMENT (( #20143 ) ) ;
#205314=CARTESIAN_POINT ( 'NONE',  ( 11.07123604129543359, 9.799999999999998934, 0.8055550039003240848 ) ) ;
#205347=AXIS2_PLACEMENT_3D ( 'NONE', #203785, #71653, #107451 ) ;
#205357=ORIENTED_EDGE ( 'NONE', *, *, #101740, .T. ) ;
#205362=B_SPLINE_CURVE_WITH_KNOTS ( 'NONE', 3,
 ( #173658, #194135, #75061, #27369, #109768, #127099 ),
 .UNSPECIFIED., .F., .F.,
 ( 4, 2, 4 ),
 ( 0.000000000000000000, 0.0003239988925529259747, 0.0006479977851058519494 ),
 .UNSPECIFIED. ) ;
#205363=DIRECTION ( 'NONE',  ( 0.000000000000000000, 0.000000000000000000, 1.000000000000000000 ) ) ;
#205374=CARTESIAN_POINT ( 'NONE',  ( -10.28816806463375144, 6.680837282875757843, -5.326249955113787848 ) ) ;
#205380=CARTESIAN_POINT ( 'NONE',  ( 8.776224899084631659, 13.27471476138782336, 8.184001253707570811 ) ) ;
#205382=VERTEX_POINT ( 'NONE', #143593 ) ;
#205388=AXIS2_PLACEMENT_3D ( 'NONE', #125781, #108452, #28196 ) ;
#205432=CARTESIAN_POINT ( 'NONE',  ( -15.75000000000000000, 11.29999999999999893, -3.200000000000001510 ) ) ;
#205447=( LENGTH_UNIT ( ) NAMED_UNIT ( * ) SI_UNIT ( .MILLI., .METRE. ) );
#205453=CARTESIAN_POINT ( 'NONE',  ( -9.812680342707254866, 4.108039100808300148, -6.337802944732694677 ) ) ;
#205458=LINE ( 'NONE', #141586, #49466 ) ;
#205462=CARTESIAN_POINT ( 'NONE',  ( 11.44791656467458374, 11.29999999999997939, 3.303228920649577294 ) ) ;
#205474=CARTESIAN_POINT ( 'NONE',  ( 6.902720145097993587, 14.55347103577521217, 9.761920446463554057 ) ) ;
#205478=SURFACE_STYLE_USAGE ( .BOTH. , #186020 ) ;
#205517=CARTESIAN_POINT ( 'NONE',  ( 11.96864102214210135, 6.616705618073630113, -0.9970986697839275825 ) ) ;
#205548=( LENGTH_UNIT ( ) NAMED_UNIT ( * ) SI_UNIT ( .MILLI., .METRE. ) );
#205564=CARTESIAN_POINT ( 'NONE',  ( 7.901650181845425891, 15.38517925215461979, -9.032942408684748514 ) ) ;
#205587=CYLINDRICAL_SURFACE ( 'NONE', #41411, 0.3999999999999997446 ) ;
#205590=CARTESIAN_POINT ( 'NONE',  ( -15.75000000000000000, 13.40000000000000036, -1.100000000000002087 ) ) ;
#205618=( NAMED_UNIT ( * ) PLANE_ANGLE_UNIT ( ) SI_UNIT ( $, .RADIAN. ) );
#205622=EDGE_CURVE ( 'NONE', #119038, #31723, #182344, .T. ) ;
#205631=CARTESIAN_POINT ( 'NONE',  ( -11.88156762547254175, 9.720000084540298957, 1.686557021358693564 ) ) ;
#205647=DIRECTION ( 'NONE',  ( 0.000000000000000000, 1.000000000000000000, 0.000000000000000000 ) ) ;
#205648=CARTESIAN_POINT ( 'NONE',  ( -11.25356361929547688, 4.972433335311166935, 5.839389443199928920 ) ) ;
#205654=CARTESIAN_POINT ( 'NONE',  ( -11.91826849282518452, 10.89999999999999858, -1.400000000000001465 ) ) ;
#205702=CARTESIAN_POINT ( 'NONE',  ( -1.785986935459600966, 14.55200959964326124, 11.82982753855158542 ) ) ;
#205705=FACE_OUTER_BOUND ( 'NONE', #96617, .T. ) ;
#205727=FACE_OUTER_BOUND ( 'NONE', #116089, .T. ) ;
#205743=UNCERTAINTY_MEASURE_WITH_UNIT (LENGTH_MEASURE( 1.000000000000000082E-05 ), #183504, 'distance_accuracy_value', 'NONE');
#205746=CARTESIAN_POINT ( 'NONE',  ( -0.8416405318397626178, 15.44692714072533590, 11.95990509367077514 ) ) ;
#205762=CARTESIAN_POINT ( 'NONE',  ( -11.97929049433705373, 11.37999999999999901, 0.7046979865771783036 ) ) ;
#205763=CARTESIAN_POINT ( 'NONE',  ( 11.08832952072288869, 9.065454946559635019, 4.456401202325765531 ) ) ;
#205764=CARTESIAN_POINT ( 'NONE',  ( -1.474414414893379099, 7.826756755319753900, 10.64843978026286386 ) ) ;
#205775=ORIENTED_EDGE ( 'NONE', *, *, #87967, .T. ) ;
#205796=CARTESIAN_POINT ( 'NONE',  ( -9.978677811866239367, 3.146997876264563843, 6.103086072356673775 ) ) ;
#205815=ORIENTED_EDGE ( 'NONE', *, *, #42056, .F. ) ;
#205819=CARTESIAN_POINT ( 'NONE',  ( -0.007339009020582241277, 15.44567596354698402, 11.95332398895799386 ) ) ;
#205848=CARTESIAN_POINT ( 'NONE',  ( -7.084991283289517661, 14.48020839276600213, 9.695715787647801065 ) ) ;
#205879=CIRCLE ( 'NONE', #84673, 11.95586206896552284 ) ;
#205909=ORIENTED_EDGE ( 'NONE', *, *, #147648, .T. ) ;
#205913=CARTESIAN_POINT ( 'NONE',  ( 10.59782195348455680, 13.80000000000000249, -3.302675849420335208 ) ) ;
#205919=ORIENTED_EDGE ( 'NONE', *, *, #135941, .T. ) ;
#205934=CARTESIAN_POINT ( 'NONE',  ( -11.97711842482174305, 7.451475930019106464, -0.9249707317075172019 ) ) ;
#205935=MECHANICAL_DESIGN_GEOMETRIC_PRESENTATION_REPRESENTATION('',(#178280),#202351);
#205987=DIRECTION ( 'NONE',  ( 0.000000000000000000, 1.000000000000000000, 0.000000000000000000 ) ) ;
#206019=FILL_AREA_STYLE ('',( #158363 ) ) ;
#206026=EDGE_CURVE ( 'NONE', #7711, #54188, #65577, .T. ) ;
#206054=ORIENTED_EDGE ( 'NONE', *, *, #211770, .F. ) ;
#206088=CARTESIAN_POINT ( 'NONE',  ( -9.860732380151581822, 3.579270011397724272, 6.765084847522528477 ) ) ;
#206099=ORIENTED_EDGE ( 'NONE', *, *, #61570, .F. ) ;
#206102=( NAMED_UNIT ( * ) PLANE_ANGLE_UNIT ( ) SI_UNIT ( $, .RADIAN. ) );
#206103=CARTESIAN_POINT ( 'NONE',  ( -10.99931038725301846, 6.873658557531565627, -3.960823121322395224 ) ) ;
#206108=CARTESIAN_POINT ( 'NONE',  ( 4.121519629048689001E-15, 14.55305236562702831, -11.95586206896554771 ) ) ;
#206146=EDGE_CURVE ( 'NONE', #198869, #178392, #170560, .T. ) ;
#206180=CARTESIAN_POINT ( 'NONE',  ( -11.55950211276791073, 13.79999999999998472, 3.221476510067111665 ) ) ;
#206181=DIRECTION ( 'NONE',  ( -0.9632918427306595976, 0.000000000000000000, -0.2684563758389253985 ) ) ;
#206182=( LENGTH_UNIT ( ) NAMED_UNIT ( * ) SI_UNIT ( .MILLI., .METRE. ) );
#206191=CARTESIAN_POINT ( 'NONE',  ( 11.74191529183257821, 6.810689793464089981, -0.9382034048196972176 ) ) ;
#206195=CARTESIAN_POINT ( 'NONE',  ( -6.755832246681736208, 14.48046842831809577, -9.927744205739022831 ) ) ;
#206197=ORIENTED_EDGE ( 'NONE', *, *, #73178, .F. ) ;
#206214=MECHANICAL_DESIGN_GEOMETRIC_PRESENTATION_REPRESENTATION('',(#188901),#102484);
#206218=FILL_AREA_STYLE ('',( #74104 ) ) ;
#206231=CARTESIAN_POINT ( 'NONE',  ( 0.000000000000000000, 9.799999999999998934, 0.000000000000000000 ) ) ;
#206242=ADVANCED_FACE ( 'NONE', ( #152193 ), #9966, .T. ) ;
#206247=CARTESIAN_POINT ( 'NONE',  ( -15.75000000000000000, 10.90000000000000036, 1.099999999999996758 ) ) ;
#206271=EDGE_CURVE ( 'NONE', #62806, #198880, #127254, .T. ) ;
#206274=DIRECTION ( 'NONE',  ( 0.000000000000000000, -1.000000000000000000, 0.000000000000000000 ) ) ;
#206292=DIRECTION ( 'NONE',  ( 0.000000000000000000, -1.445602896647338917E-16, 1.000000000000000000 ) ) ;
#206299=CARTESIAN_POINT ( 'NONE',  ( 9.633311866038676285, 13.62946609490282235, 8.224406077922058245 ) ) ;
#206305=AXIS2_PLACEMENT_3D ( 'NONE', #182445, #53525, #103346 ) ;
#206332=CARTESIAN_POINT ( 'NONE',  ( -11.34338453707543515, 5.310936115193626961, -5.661293933977025183 ) ) ;
#206337=TOROIDAL_SURFACE ( 'NONE', #119981, 12.17999951260719804, 0.5000000000000008882 ) ;
#206338=DIRECTION ( 'NONE',  ( -1.000000000000000000, 0.000000000000000000, 0.000000000000000000 ) ) ;
#206359=CARTESIAN_POINT ( 'NONE',  ( 9.842318685493841812, 11.92143744661629867, 6.868033326349857859 ) ) ;
#206362=CARTESIAN_POINT ( 'NONE',  ( -11.48243876534946040, 11.37999999999999901, -3.200000000000001510 ) ) ;
#206408=EDGE_CURVE ( 'NONE', #169055, #45206, #53618, .T. ) ;
#206409=CARTESIAN_POINT ( 'NONE',  ( -1.734723475976807094E-15, 3.481548657788671619, -11.92000000000000171 ) ) ;
#206417=CARTESIAN_POINT ( 'NONE',  ( 11.94654170777226376, 11.15174326158935969, 1.134972293687618539 ) ) ;
#206423=SURFACE_STYLE_USAGE ( .BOTH. , #109004 ) ;
#206439=CARTESIAN_POINT ( 'NONE',  ( -11.41381675112453387, 10.19999999999999929, -3.704697986577184299 ) ) ;
#206447=CARTESIAN_POINT ( 'NONE',  ( -10.48266952940149466, 5.268049057482275366, -5.154014898524191146 ) ) ;
#206456=ORIENTED_EDGE ( 'NONE', *, *, #164554, .F. ) ;
#206466=FILL_AREA_STYLE_COLOUR ( '', #99383 ) ;
#206515=CARTESIAN_POINT ( 'NONE',  ( 1.500000000000035971, 7.750000000000000000, 10.99818166789401275 ) ) ;
#206520=CARTESIAN_POINT ( 'NONE',  ( -10.83922355283164407, 5.627439893072524235, -6.488667358217312220 ) ) ;
#206531=MECHANICAL_DESIGN_GEOMETRIC_PRESENTATION_REPRESENTATION('',(#50847),#106258);
#206552=EDGE_CURVE ( 'NONE', #176022, #170509, #6549, .T. ) ;
#206582=UNCERTAINTY_MEASURE_WITH_UNIT (LENGTH_MEASURE( 1.000000000000000082E-05 ), #123017, 'distance_accuracy_value', 'NONE');
#206588=CARTESIAN_POINT ( 'NONE',  ( 8.776224899084628106, 13.27471476138783224, 8.184001253707569035 ) ) ;
#206597=B_SPLINE_CURVE_WITH_KNOTS ( 'NONE', 3,
 ( #516, #15725, #65533, #182489, #167330, #131679 ),
 .UNSPECIFIED., .F., .F.,
 ( 4, 2, 4 ),
 ( 0.0006378314054480077946, 0.0009584618939205538689, 0.001279092382393099943 ),
 .UNSPECIFIED. ) ;
#206612=CYLINDRICAL_SURFACE ( 'NONE', #123758, 0.3999999999999997446 ) ;
#206614=CARTESIAN_POINT ( 'NONE',  ( 10.50000000000000178, 0.000000000000000000, 3.599999999999999201 ) ) ;
#206662=EDGE_CURVE ( 'NONE', #102037, #169596, #116854, .T. ) ;
#206688=ORIENTED_EDGE ( 'NONE', *, *, #111757, .T. ) ;
#206704=CARTESIAN_POINT ( 'NONE',  ( -11.35610322553117513, 9.985783710708231453, 3.553412924323500199 ) ) ;
#206719=CARTESIAN_POINT ( 'NONE',  ( -11.97929049433705728, 13.80000000000000071, 0.7046979865771805240 ) ) ;
#206720=CARTESIAN_POINT ( 'NONE',  ( -10.14895191633106819, 2.999999999999999112, 7.601392964450658596 ) ) ;
#206751=CARTESIAN_POINT ( 'NONE',  ( -11.41381675112453387, 10.89999999999998259, 3.704697986577180746 ) ) ;
#206765=CARTESIAN_POINT ( 'NONE',  ( 8.776573235218638303, 13.27486625357122385, -8.183627694784497919 ) ) ;
#206772=PRESENTATION_STYLE_ASSIGNMENT (( #140760 ) ) ;
#206782=FACE_OUTER_BOUND ( 'NONE', #178966, .T. ) ;
#206787=CARTESIAN_POINT ( 'NONE',  ( -11.78331023100045627, 13.79999999999999893, -1.800000000000001155 ) ) ;
#206813=CARTESIAN_POINT ( 'NONE',  ( -0.8446225718669002624, 15.51843453237083459, 12.00404876522673447 ) ) ;
#206823=ORIENTED_EDGE ( 'NONE', *, *, #147049, .F. ) ;
#206827=SURFACE_STYLE_USAGE ( .BOTH. , #11823 ) ;
#206829=CARTESIAN_POINT ( 'NONE',  ( 11.47058495203700623, 8.376874303918512510, -3.372313987538385405 ) ) ;
#206853=SURFACE_STYLE_USAGE ( .BOTH. , #155991 ) ;
#206861=CARTESIAN_POINT ( 'NONE',  ( -9.915825940873133959, 4.173851563286998356, 6.175246223022227809 ) ) ;
#206865=UNCERTAINTY_MEASURE_WITH_UNIT (LENGTH_MEASURE( 1.000000000000000082E-05 ), #5118, 'distance_accuracy_value', 'NONE');
#206871=STYLED_ITEM ( 'NONE', ( #23629 ), #39092 ) ;
#206880=ORIENTED_EDGE ( 'NONE', *, *, #206146, .T. ) ;
#206887=STYLED_ITEM ( 'NONE', ( #11435 ), #46551 ) ;
#206911=CARTESIAN_POINT ( 'NONE',  ( -11.04536101718726293, 12.69999999999999929, -1.100000000000000311 ) ) ;
#206947=CARTESIAN_POINT ( 'NONE',  ( 10.50000000000000178, 13.39999999999998259, 3.599999999999999201 ) ) ;
#206948=DIRECTION ( 'NONE',  ( -0.000000000000000000, -0.000000000000000000, 1.000000000000000000 ) ) ;
#206982=ORIENTED_EDGE ( 'NONE', *, *, #27605, .F. ) ;
#206983=CARTESIAN_POINT ( 'NONE',  ( -11.84668730067608422, 13.40000000000000036, -1.400000000000001688 ) ) ;
#206984=EDGE_LOOP ( 'NONE', ( #99782, #106916, #88778, #3473 ) ) ;
#207001=CARTESIAN_POINT ( 'NONE',  ( 7.576886519560940947, 14.99604748842864410, 10.16829559912798686 ) ) ;
#207015=ORIENTED_EDGE ( 'NONE', *, *, #122495, .F. ) ;
#207018=ORIENTED_EDGE ( 'NONE', *, *, #20246, .F. ) ;
#207023=CARTESIAN_POINT ( 'NONE',  ( -11.52469724861193967, 13.87999993351231254, -3.346365485506884063 ) ) ;
#207030=CARTESIAN_POINT ( 'NONE',  ( 11.41381675112453742, 19.00000000000000000, 3.704697986577180746 ) ) ;
#207032=DIRECTION ( 'NONE',  ( -0.000000000000000000, -1.000000000000000000, -0.000000000000000000 ) ) ;
#207039=AXIS2_PLACEMENT_3D ( 'NONE', #16434, #182137, #164842 ) ;
#207060=ORIENTED_EDGE ( 'NONE', *, *, #129145, .F. ) ;
#207086=ORIENTED_EDGE ( 'NONE', *, *, #3092, .T. ) ;
#207113=CARTESIAN_POINT ( 'NONE',  ( 0.000000000000000000, 4.000000000000002665, 1.105031132475055157E-32 ) ) ;
#207119=CARTESIAN_POINT ( 'NONE',  ( -11.86145016429273014, 12.69999999999999929, -1.100000000000000311 ) ) ;
#207130=CARTESIAN_POINT ( 'NONE',  ( 1.050790385994986975, 15.00000000000000711, -12.64745918785790835 ) ) ;
#207151=VECTOR ( 'NONE', #213833, 1000.000000000000000 ) ;
#207167=CARTESIAN_POINT ( 'NONE',  ( 11.48243876534946217, 11.29999999999998117, 3.199999999999997957 ) ) ;
#207175=CARTESIAN_POINT ( 'NONE',  ( -10.45142907045522129, 5.144535043903895932, -5.216774619840575333 ) ) ;
#207179=CARTESIAN_POINT ( 'NONE',  ( -4.385872067527455620, 14.53055287205049240, -11.17868682968782856 ) ) ;
#207180=DIRECTION ( 'NONE',  ( 0.000000000000000000, 1.000000000000000000, 0.000000000000000000 ) ) ;
#207192=CARTESIAN_POINT ( 'NONE',  ( -10.50000000000000000, 0.000000000000000000, -3.600000000000002309 ) ) ;
#207217=EDGE_CURVE ( 'NONE', #54318, #149901, #199808, .T. ) ;
#207224=DIRECTION ( 'NONE',  ( 0.8164965809277251463, 0.000000000000000000, 0.5773502691896270633 ) ) ;
#207244=CARTESIAN_POINT ( 'NONE',  ( 11.88209931242717943, 7.837836862524945936, -1.732717975941681532 ) ) ;
#207262=CARTESIAN_POINT ( 'NONE',  ( 8.858328068414154544, 13.09032149711157444, 7.626023304531035052 ) ) ;
#207282=CARTESIAN_POINT ( 'NONE',  ( -15.75000000000000000, 12.30000000000000071, -0.7000000000000009548 ) ) ;
#207298=( GEOMETRIC_REPRESENTATION_CONTEXT ( 3 ) GLOBAL_UNCERTAINTY_ASSIGNED_CONTEXT ( ( #45165 ) ) GLOBAL_UNIT_ASSIGNED_CONTEXT ( ( #210151, #127961, #194987 ) ) REPRESENTATION_CONTEXT ( 'NONE', 'WORKASPACE' ) );
#207328=STYLED_ITEM ( 'NONE', ( #19080 ), #43714 ) ;
#207343=CIRCLE ( 'NONE', #141692, 0.07999999999999946043 ) ;
#207374=CARTESIAN_POINT ( 'NONE',  ( 9.482679952114482447, 14.00853213111861351, 8.402045824544956076 ) ) ;
#207391=CARTESIAN_POINT ( 'NONE',  ( 11.94651559118242190, 9.948693441210290089, 1.135242698369639980 ) ) ;
#207394=( BOUNDED_SURFACE ( )  B_SPLINE_SURFACE ( 3, 2, ( 
 ( #106629, #187812, #122926 ),
 ( #205118, #121841, #25317 ),
 ( #24233, #123985, #38371 ),
 ( #172658, #9074, #7991 ),
 ( #5841, #189952, #74082 ),
 ( #140173, #188884, #71912 ) ),
 .UNSPECIFIED., .F., .F., .T. ) 
 B_SPLINE_SURFACE_WITH_KNOTS ( ( 4, 2, 4 ),
 ( 3, 3 ),
 ( -4.065758146820641628E-19, 0.0003831416164015016010, 0.0007662832328030036357 ),
 ( 0.000000000000000000, 1.000000000000000000 ),
 .UNSPECIFIED. ) 
 GEOMETRIC_REPRESENTATION_ITEM ( )  RATIONAL_B_SPLINE_SURFACE ( (
 ( 1.000000000000000000, 0.7071067811865475727, 1.000000000000000000),
 ( 1.000000000000000000, 0.6829713513656306967, 1.000000000000000000),
 ( 1.000000000000000000, 0.6534833722368420528, 1.000000000000000000),
 ( 1.000000000000000000, 0.6054027484666428816, 1.000000000000000000),
 ( 1.000000000000000000, 0.5875453974412050417, 1.000000000000000000),
 ( 1.000000000000000000, 0.5879095031487528988, 1.000000000000000000) ) ) 
 REPRESENTATION_ITEM ( '' )  SURFACE ( )  );
#207405=CARTESIAN_POINT ( 'NONE',  ( -11.43645483535884999, 5.654992568747732484, -5.469194708833876817 ) ) ;
#207429=CARTESIAN_POINT ( 'NONE',  ( 10.70559879711738560, 9.877729115460759601, 5.430853593049171479 ) ) ;
#207441=CARTESIAN_POINT ( 'NONE',  ( 11.04978080397792972, 13.60844524987713022, 1.057339094031727988 ) ) ;
#207491=FILL_AREA_STYLE_COLOUR ( '', #78291 ) ;
#207506=EDGE_CURVE ( 'NONE', #158047, #133272, #172014, .T. ) ;
#207510=CYLINDRICAL_SURFACE ( 'NONE', #71891, 0.3999999999999996891 ) ;
#207513=ORIENTED_EDGE ( 'NONE', *, *, #16160, .T. ) ;
#207519=CARTESIAN_POINT ( 'NONE',  ( -9.997720234198379075, 5.662301760159435204, -5.943093865039206669 ) ) ;
#207527=EDGE_LOOP ( 'NONE', ( #36493, #134314, #191689, #150046 ) ) ;
#207534=ORIENTED_EDGE ( 'NONE', *, *, #139088, .T. ) ;
#207555=( NAMED_UNIT ( * ) PLANE_ANGLE_UNIT ( ) SI_UNIT ( $, .RADIAN. ) );
#207566=( BOUNDED_SURFACE ( )  B_SPLINE_SURFACE ( 3, 2, ( 
 ( #19842, #199653, #70707 ),
 ( #35024, #198585, #36092 ),
 ( #53419, #167182, #3574 ),
 ( #182341, #150945, #136820 ),
 ( #49178, #165044, #101096 ),
 ( #181286, #32913, #102176 ) ),
 .UNSPECIFIED., .F., .F., .F. ) 
 B_SPLINE_SURFACE_WITH_KNOTS ( ( 4, 2, 4 ),
 ( 3, 3 ),
 ( 0.000000000000000000, 0.0003766365702389426712, 0.0007532731404778853423 ),
 ( 0.000000000000000000, 1.000000000000000000 ),
 .UNSPECIFIED. ) 
 GEOMETRIC_REPRESENTATION_ITEM ( )  RATIONAL_B_SPLINE_SURFACE ( (
 ( 1.000000000000000000, 0.7452309222762957264, 1.000000000000000000),
 ( 1.000000000000000000, 0.7451892422674152305, 1.000000000000000000),
 ( 1.000000000000000000, 0.7429606254235439078, 1.000000000000000000),
 ( 1.000000000000000000, 0.7311462761268936461, 1.000000000000000000),
 ( 1.000000000000000000, 0.7212257702788928970, 1.000000000000000000),
 ( 1.000000000000000000, 0.7071067811865474617, 1.000000000000000000) ) ) 
 REPRESENTATION_ITEM ( '' )  SURFACE ( )  );
#207589=CARTESIAN_POINT ( 'NONE',  ( -10.67060214796032724, 5.239869845146935212, -6.813287888368859235 ) ) ;
#207604=VERTEX_POINT ( 'NONE', #30123 ) ;
#207656=EDGE_CURVE ( 'NONE', #96576, #90728, #187735, .T. ) ;
#207662=B_SPLINE_CURVE_WITH_KNOTS ( 'NONE', 3,
 ( #97176, #132880, #163230, #182648, #14812, #80903 ),
 .UNSPECIFIED., .F., .F.,
 ( 4, 2, 4 ),
 ( 0.001279092382393099943, 0.001599469101539996744, 0.001919845820686893545 ),
 .UNSPECIFIED. ) ;
#207672=CARTESIAN_POINT ( 'NONE',  ( 11.91294103507080315, 9.985399100435895292, 1.446263142085468134 ) ) ;
#207681=( LENGTH_UNIT ( ) NAMED_UNIT ( * ) SI_UNIT ( .MILLI., .METRE. ) );
#207692=CARTESIAN_POINT ( 'NONE',  ( 11.05216697254199865, 8.017870898877115238, 4.562987691682096170 ) ) ;
#207702=DIRECTION ( 'NONE',  ( -1.000000000000000000, 0.000000000000000000, 0.000000000000000000 ) ) ;
#207709=DIRECTION ( 'NONE',  ( -0.000000000000000000, 1.000000000000000000, -0.000000000000000000 ) ) ;
#207712=DIRECTION ( 'NONE',  ( 0.000000000000000000, 0.000000000000000000, 1.000000000000000000 ) ) ;
#207775=FACE_OUTER_BOUND ( 'NONE', #207527, .T. ) ;
#207781=CARTESIAN_POINT ( 'NONE',  ( -10.81685113641997020, 3.157239479008171035, 6.648618798508739935 ) ) ;
#207786=CARTESIAN_POINT ( 'NONE',  ( -11.92619526248524409, 11.02744613914173932, -1.328859120100604585 ) ) ;
#207788=( NAMED_UNIT ( * ) SI_UNIT ( $, .STERADIAN. ) SOLID_ANGLE_UNIT ( ) );
#207790=ORIENTED_EDGE ( 'NONE', *, *, #129145, .T. ) ;
#207821=DIRECTION ( 'NONE',  ( 0.000000000000000000, -1.000000000000000000, -9.023263958591317418E-17 ) ) ;
#207827=ORIENTED_EDGE ( 'NONE', *, *, #185659, .F. ) ;
#207836=AXIS2_PLACEMENT_3D ( 'NONE', #64893, #198088, #101666 ) ;
#207837=DIRECTION ( 'NONE',  ( 0.000000000000000000, 0.000000000000000000, 1.000000000000000000 ) ) ;
#207841=AXIS2_PLACEMENT_3D ( 'NONE', #113666, #198031, #65872 ) ;
#207842=CARTESIAN_POINT ( 'NONE',  ( -11.48243876534946040, 9.799999999999998934, -3.200000000000001510 ) ) ;
#207847=PRESENTATION_STYLE_ASSIGNMENT (( #172174 ) ) ;
#207860=CARTESIAN_POINT ( 'NONE',  ( 1.474420525118734323E-15, 14.99987590242439595, 11.68000000000000327 ) ) ;
#207872=EDGE_CURVE ( 'NONE', #210693, #106547, #191021, .T. ) ;
#207892=CARTESIAN_POINT ( 'NONE',  ( -15.75000000000000000, 12.69999999999999929, -1.400000000000001910 ) ) ;
#207894=CARTESIAN_POINT ( 'NONE',  ( 10.19581844778559621, 10.80880345838189527, 6.242887950171588152 ) ) ;
#207898=CARTESIAN_POINT ( 'NONE',  ( -15.75000000000000000, 11.29999999999998117, 3.199999999999997957 ) ) ;
#207906=ORIENTED_EDGE ( 'NONE', *, *, #147938, .T. ) ;
#207917=( LENGTH_UNIT ( ) NAMED_UNIT ( * ) SI_UNIT ( .MILLI., .METRE. ) );
#207933=DIRECTION ( 'NONE',  ( 0.000000000000000000, 0.000000000000000000, 1.000000000000000000 ) ) ;
#207940=MECHANICAL_DESIGN_GEOMETRIC_PRESENTATION_REPRESENTATION('',(#200954),#45308);
#207946=CARTESIAN_POINT ( 'NONE',  ( -11.43209210103587559, 9.944039240160824633, 3.649125173352122609 ) ) ;
#207975=CARTESIAN_POINT ( 'NONE',  ( -4.304609288505035103, 14.53049063336417746, 11.21048893683339642 ) ) ;
#208004=ORIENTED_EDGE ( 'NONE', *, *, #119318, .T. ) ;
#208014=DIRECTION ( 'NONE',  ( 0.000000000000000000, 0.000000000000000000, 1.000000000000000000 ) ) ;
#208028=CARTESIAN_POINT ( 'NONE',  ( -1.734723475976807094E-15, 4.446955548196619645, -11.95586206894145676 ) ) ;
#208063=CARTESIAN_POINT ( 'NONE',  ( 9.633311866038676285, 13.62946609490282235, 8.224406077922058245 ) ) ;
#208086=CARTESIAN_POINT ( 'NONE',  ( -11.55950211276791428, 13.80000000000000071, -3.221476510067116550 ) ) ;
#208092=AXIS2_PLACEMENT_3D ( 'NONE', #19956, #52475, #87105 ) ;
#208103=AXIS2_PLACEMENT_3D ( 'NONE', #162605, #81342, #29404 ) ;
#208110=CARTESIAN_POINT ( 'NONE',  ( 8.371655185961106582, 14.07500887114600197, 8.535501002982430307 ) ) ;
#208132=EDGE_CURVE ( 'NONE', #175615, #93441, #27280, .T. ) ;
#208136=CARTESIAN_POINT ( 'NONE',  ( 11.91826848330681976, 11.00729645956991654, -1.400000080589506979 ) ) ;
#208150=CIRCLE ( 'NONE', #114834, 0.07999999999999933553 ) ;
#208182=VERTEX_POINT ( 'NONE', #109864 ) ;
#208203=B_SPLINE_CURVE_WITH_KNOTS ( 'NONE', 3,
 ( #176649, #125847, #28261, #42406, #91153, #93289, #109588, #26115 ),
 .UNSPECIFIED., .F., .F.,
 ( 4, 2, 2, 4 ),
 ( -5.999999999723453794E-08, 0.001495742970897297663, 0.002243644456345944907, 0.002991545941794591934 ),
 .UNSPECIFIED. ) ;
#208218=CARTESIAN_POINT ( 'NONE',  ( -10.24975248460684440, 3.776839368175542777, 6.158671921171848140 ) ) ;
#208232=CARTESIAN_POINT ( 'NONE',  ( 11.78331023100045627, 13.79999999999998295, 1.799999999999999600 ) ) ;
#208237=CARTESIAN_POINT ( 'NONE',  ( -8.770850689852672133, 14.55305235829676391, -8.174590314132164082 ) ) ;
#208289=CARTESIAN_POINT ( 'NONE',  ( -11.52888687719611660, 11.29423125105035730, -3.331331986263548650 ) ) ;
#208303=CARTESIAN_POINT ( 'NONE',  ( 9.502044606515637426, 13.11535572295773555, 7.329770145308074802 ) ) ;
#208312=PRESENTATION_STYLE_ASSIGNMENT (( #106615 ) ) ;
#208321=CARTESIAN_POINT ( 'NONE',  ( 9.053633104220391914, 12.24030617166337898, -7.400564859916917371 ) ) ;
#208338=STYLED_ITEM ( 'NONE', ( #132995 ), #30072 ) ;
#208339=CARTESIAN_POINT ( 'NONE',  ( 9.518950567327413737, 3.582805947358006282, -7.307358422849591584 ) ) ;
#208400=FILL_AREA_STYLE_COLOUR ( '', #208755 ) ;
#208418=SHAPE_REPRESENTATION_RELATIONSHIP ( 'NONE' , 'NONE' ,  #135824, #24096 ) ;
#208422=CARTESIAN_POINT ( 'NONE',  ( -15.75000000000000000, 11.29999999999999893, -1.800000000000001155 ) ) ;
#208425=CARTESIAN_POINT ( 'NONE',  ( 7.457833306149189490, 16.00157973104908393, 10.25342808721416077 ) ) ;
#208431=ORIENTED_EDGE ( 'NONE', *, *, #158613, .T. ) ;
#208447=PLANE ( 'NONE',  #5529 ) ;
#208457=CARTESIAN_POINT ( 'NONE',  ( -11.03376256896084584, 6.348997720274319079, -6.086949085616508270 ) ) ;
#208458=EDGE_CURVE ( 'NONE', #131174, #124865, #194238, .T. ) ;
#208480=VERTEX_POINT ( 'NONE', #161760 ) ;
#208481=CARTESIAN_POINT ( 'NONE',  ( 10.87086078464171202, 9.638125288626520515, -5.094357749550133541 ) ) ;
#208490=DIRECTION ( 'NONE',  ( 0.000000000000000000, 0.000000000000000000, 1.000000000000000000 ) ) ;
#208492=CARTESIAN_POINT ( 'NONE',  ( -11.94105721237523099, 10.90000000000000036, 1.187919463087248273 ) ) ;
#208551=EDGE_LOOP ( 'NONE', ( #25996, #155865, #79879, #108574, #74059, #7740, #41357, #58205 ) ) ;
#208559=EDGE_CURVE ( 'NONE', #77381, #152468, #197909, .T. ) ;
#208563=EDGE_CURVE ( 'NONE', #144257, #132208, #267, .T. ) ;
#208568=CARTESIAN_POINT ( 'NONE',  ( -12.36958382383909871, 9.653479897959526213, -1.396270995789667513 ) ) ;
#208572=ORIENTED_EDGE ( 'NONE', *, *, #176386, .T. ) ;
#208574=FACE_OUTER_BOUND ( 'NONE', #164871, .T. ) ;
#208599=CARTESIAN_POINT ( 'NONE',  ( 11.48243876534946217, 12.21999999999998288, 3.199999999999997957 ) ) ;
#208635=ORIENTED_EDGE ( 'NONE', *, *, #32909, .F. ) ;
#208640=FILL_AREA_STYLE_COLOUR ( '', #200258 ) ;
#208645=CARTESIAN_POINT ( 'NONE',  ( -11.05174500248992331, 4.511067306307721125, -6.216760965876352962 ) ) ;
#208676=AXIS2_PLACEMENT_3D ( 'NONE', #80063, #30259, #176506 ) ;
#208712=EDGE_CURVE ( 'NONE', #62106, #14287, #29911, .T. ) ;
#208749=EDGE_CURVE ( 'NONE', #178392, #72859, #186513, .T. ) ;
#208755=COLOUR_RGB ( '', 0.31764706, 0.68627451, 0.89019608) ;
#208773=DIRECTION ( 'NONE',  ( 1.000000000000000000, -0.000000000000000000, -0.000000000000000000 ) ) ;
#208777=ADVANCED_FACE ( 'NONE', ( #154031 ), #154997, .F. ) ;
#208785=CARTESIAN_POINT ( 'NONE',  ( 9.356044174147720938, 13.88059531916365508, -7.514793805895062739 ) ) ;
#208819=EDGE_CURVE ( 'NONE', #156687, #158767, #166008, .T. ) ;
#208835=ORIENTED_EDGE ( 'NONE', *, *, #210828, .F. ) ;
#208838=CARTESIAN_POINT ( 'NONE',  ( 12.43309052428753070, 7.572468744233063376, 1.895192891247173606 ) ) ;
#208848=CARTESIAN_POINT ( 'NONE',  ( -11.07123604129543182, 13.79999999999999538, 0.8055550039003244178 ) ) ;
#208861=CARTESIAN_POINT ( 'NONE',  ( 9.475937867762608491, 4.398642301159960688, -7.290291149262039916 ) ) ;
#208891=CARTESIAN_POINT ( 'NONE',  ( -9.333041836230020039, 14.55305236562984383, 7.472413793098202639 ) ) ;
#208902=DIRECTION ( 'NONE',  ( 0.000000000000000000, -1.000000000000000000, -1.804652791718263484E-16 ) ) ;
#208906=CARTESIAN_POINT ( 'NONE',  ( -10.79323474359244805, 4.699907862511227385, 5.141973737680021195 ) ) ;
#208909=ORIENTED_EDGE ( 'NONE', *, *, #213110, .F. ) ;
#208945=DIRECTION ( 'NONE',  ( 0.000000000000000000, 1.000000000000000000, 0.000000000000000000 ) ) ;
#208949=CARTESIAN_POINT ( 'NONE',  ( 11.55950211276791251, 13.87999999999998302, 3.221476510067114329 ) ) ;
#208952=EDGE_CURVE ( 'NONE', #86738, #30509, #170264, .T. ) ;
#208966=VECTOR ( 'NONE', #31140, 1000.000000000000000 ) ;
#209035=CARTESIAN_POINT ( 'NONE',  ( -11.81911962874431055, 11.25710573484113830, 1.591749704452489533 ) ) ;
#209041=( LENGTH_UNIT ( ) NAMED_UNIT ( * ) SI_UNIT ( .MILLI., .METRE. ) );
#209056=VERTEX_POINT ( 'NONE', #200612 ) ;
#209075=CARTESIAN_POINT ( 'NONE',  ( 11.33772463945036790, 10.90000000000000036, -3.680000000000002824 ) ) ;
#209096=CARTESIAN_POINT ( 'NONE',  ( 11.00592642091246454, 12.48979727563561504, 1.444015479094872934 ) ) ;
#209118=ADVANCED_FACE ( 'NONE', ( #67404 ), #55470, .T. ) ;
#209120=FACE_OUTER_BOUND ( 'NONE', #67171, .T. ) ;
#209153=CARTESIAN_POINT ( 'NONE',  ( -11.92619526913699879, 10.19999999999999929, -1.328859060402686199 ) ) ;
#209157=CIRCLE ( 'NONE', #108910, 0.5000000000000004441 ) ;
#209167=FILL_AREA_STYLE_COLOUR ( '', #210351 ) ;
#209205=ORIENTED_EDGE ( 'NONE', *, *, #75095, .T. ) ;
#209217=ORIENTED_EDGE ( 'NONE', *, *, #179732, .F. ) ;
#209249=ORIENTED_EDGE ( 'NONE', *, *, #73875, .F. ) ;
#209280=FACE_OUTER_BOUND ( 'NONE', #104319, .T. ) ;
#209287=CARTESIAN_POINT ( 'NONE',  ( -11.14389002924298566, 7.220603907090449525, 3.549113525960188031 ) ) ;
#209291=CARTESIAN_POINT ( 'NONE',  ( -3.099846755496448392, 14.55179011166401892, -11.55524956803910008 ) ) ;
#209339=EDGE_CURVE ( 'NONE', #195013, #127020, #57596, .T. ) ;
#209355=B_SPLINE_CURVE_WITH_KNOTS ( 'NONE', 3,
 ( #8388, #122245, #39841, #75535, #109175, #10518 ),
 .UNSPECIFIED., .F., .F.,
 ( 4, 2, 4 ),
 ( 0.000000000000000000, 0.0003168911866439334617, 0.0006337823732878669234 ),
 .UNSPECIFIED. ) ;
#209360=CARTESIAN_POINT ( 'NONE',  ( 9.605809254248283580, 12.70095519382022964, -7.195141037656365590 ) ) ;
#209365=( GEOMETRIC_REPRESENTATION_CONTEXT ( 3 ) GLOBAL_UNCERTAINTY_ASSIGNED_CONTEXT ( ( #146936 ) ) GLOBAL_UNIT_ASSIGNED_CONTEXT ( ( #179971, #150677, #97668 ) ) REPRESENTATION_CONTEXT ( 'NONE', 'WORKASPACE' ) );
#209369=EDGE_CURVE ( 'NONE', #152913, #149077, #143157, .T. ) ;
#209380=CARTESIAN_POINT ( 'NONE',  ( 11.84405005182567727, 6.745048178605705935, -3.657409634699734458 ) ) ;
#209383=EDGE_LOOP ( 'NONE', ( #3363, #81426, #120328, #38864 ) ) ;
#209385=VERTEX_POINT ( 'NONE', #105297 ) ;
#209403=CARTESIAN_POINT ( 'NONE',  ( 9.427850895902817996, 13.54474674066948481, 7.423989997610750180 ) ) ;
#209404=CARTESIAN_POINT ( 'NONE',  ( -15.75000000000000000, 13.79999999999998295, 1.799999999999999600 ) ) ;
#209409=CARTESIAN_POINT ( 'NONE',  ( -11.94650005372637835, 11.15102700337638097, -1.135399707157295435 ) ) ;
#209439=CARTESIAN_POINT ( 'NONE',  ( 0.7124089920922619390, 15.00000000000000355, 12.66466791154580207 ) ) ;
#209440=DIRECTION ( 'NONE',  ( 0.000000000000000000, 0.000000000000000000, -1.000000000000000000 ) ) ;
#209444=CARTESIAN_POINT ( 'NONE',  ( 10.50000000000000178, 12.69999999999998153, 3.599999999999999201 ) ) ;
#209451=CARTESIAN_POINT ( 'NONE',  ( 11.04536101718726293, 10.19999999999999929, -1.100000000000000311 ) ) ;
#209464=AXIS2_PLACEMENT_3D ( 'NONE', #71385, #55168, #187287 ) ;
#209468=DIRECTION ( 'NONE',  ( -0.05872483221476459958, -0.000000000000000000, -0.9982742078614211811 ) ) ;
#209469=LINE ( 'NONE', #93636, #51206 ) ;
#209480=DIRECTION ( 'NONE',  ( -0.000000000000000000, 1.000000000000000000, 1.804652791718263484E-16 ) ) ;
#209487=CARTESIAN_POINT ( 'NONE',  ( 7.207828345953949167, 14.97151529443900486, 9.191422221725781938 ) ) ;
#209495=B_SPLINE_CURVE_WITH_KNOTS ( 'NONE', 3,
 ( #58492, #75806, #89948, #144057, #107305, #155998, #57425, #123587, #189551, #41198, #91013, #141914, #33452 ),
 .UNSPECIFIED., .F., .F.,
 ( 4, 3, 3, 3, 4 ),
 ( -1.794875635996206868E-06, 0.000000000000000000, 4.049120399957791379E-05, 8.114731789401420019E-05, 0.0001124919062838589578 ),
 .UNSPECIFIED. ) ;
#209521=CARTESIAN_POINT ( 'NONE',  ( -10.50660484223216606, 5.359830900411396648, 5.105327592218940502 ) ) ;
#209538=CARTESIAN_POINT ( 'NONE',  ( -9.333041836230021815, 14.55305236562984383, 7.472413793098204415 ) ) ;
#209545=CARTESIAN_POINT ( 'NONE',  ( 10.80604400872368132, 9.580061684330026139, -5.115041846163436823 ) ) ;
#209603=CARTESIAN_POINT ( 'NONE',  ( -11.76006714841412837, 8.561852472810636883, -2.403998662577486733 ) ) ;
#209617=VERTEX_POINT ( 'NONE', #191839 ) ;
#209629=CARTESIAN_POINT ( 'NONE',  ( 11.86145016429272836, 13.40000000000000036, -1.180000000000002158 ) ) ;
#209637=CARTESIAN_POINT ( 'NONE',  ( -12.45759369916135029, 8.320971494343229580, 2.471636155840711169 ) ) ;
#209709=CARTESIAN_POINT ( 'NONE',  ( -10.81809272050965376, 3.158133435639066899, -6.646723133134004868 ) ) ;
#209722=EDGE_CURVE ( 'NONE', #129981, #48908, #109622, .T. ) ;
#209727=CIRCLE ( 'NONE', #123420, 0.08000000000000020983 ) ;
#209766=COLOUR_RGB ( '', 0.08235294, 0.09019608, 0.10196078) ;
#209785=( NAMED_UNIT ( * ) PLANE_ANGLE_UNIT ( ) SI_UNIT ( $, .RADIAN. ) );
#209789=ORIENTED_EDGE ( 'NONE', *, *, #84048, .F. ) ;
#209795=ORIENTED_EDGE ( 'NONE', *, *, #92162, .T. ) ;
#209809=LINE ( 'NONE', #80898, #196781 ) ;
#209811=CARTESIAN_POINT ( 'NONE',  ( 8.790098660144264997, 13.29414747594432455, 8.101455065885630802 ) ) ;
#209814=CARTESIAN_POINT ( 'NONE',  ( -9.800782855757772083, 4.518459118458827639, 6.931930279218311064 ) ) ;
#209818=CARTESIAN_POINT ( 'NONE',  ( -9.494457024495529751, 14.66554680615851325, -7.338830936511814507 ) ) ;
#209848=CARTESIAN_POINT ( 'NONE',  ( 7.903398181601305694, 15.38462505118610757, -9.031418266963273211 ) ) ;
#209870=AXIS2_PLACEMENT_3D ( 'NONE', #85959, #133681, #21986 ) ;
#209881=EDGE_CURVE ( 'NONE', #174627, #156842, #59721, .T. ) ;
#209900=CARTESIAN_POINT ( 'NONE',  ( 10.14021943694179839, 13.64433865160459192, -7.295449844790285354 ) ) ;
#209951=ADVANCED_FACE ( 'NONE', ( #122691 ), #120436, .F. ) ;
#209952=CARTESIAN_POINT ( 'NONE',  ( 0.000000000000000000, 7.000000000000000000, 0.000000000000000000 ) ) ;
#209958=CARTESIAN_POINT ( 'NONE',  ( -15.75000000000000000, 11.29999999999999893, 0.6999999999999992895 ) ) ;
#209967=SURFACE_STYLE_FILL_AREA ( #92005 ) ;
#210012=SURFACE_STYLE_USAGE ( .BOTH. , #176475 ) ;
#210028=VERTEX_POINT ( 'NONE', #210223 ) ;
#210080=AXIS2_PLACEMENT_3D ( 'NONE', #156312, #142219, #91325 ) ;
#210081=ORIENTED_EDGE ( 'NONE', *, *, #54609, .F. ) ;
#210107=CARTESIAN_POINT ( 'NONE',  ( -11.92051736251533534, 11.15180243792676862, 1.381800029228856808 ) ) ;
#210110=DIRECTION ( 'NONE',  ( -0.000000000000000000, -1.000000000000000000, -0.000000000000000000 ) ) ;
#210134=CARTESIAN_POINT ( 'NONE',  ( 11.41381678389391574, 12.57120581758927003, -3.704697885617874942 ) ) ;
#210146=ORIENTED_EDGE ( 'NONE', *, *, #192419, .F. ) ;
#210151=( LENGTH_UNIT ( ) NAMED_UNIT ( * ) SI_UNIT ( .MILLI., .METRE. ) );
#210168=FILL_AREA_STYLE ('',( #161456 ) ) ;
#210187=EDGE_CURVE ( 'NONE', #204424, #183827, #19990, .T. ) ;
#210190=CARTESIAN_POINT ( 'NONE',  ( -11.97929049433705373, 13.88000000000000078, 0.7046979865771783036 ) ) ;
#210200=CARTESIAN_POINT ( 'NONE',  ( -11.97185388258315086, 9.720000092796073687, -0.8311143155443163621 ) ) ;
#210223=CARTESIAN_POINT ( 'NONE',  ( -10.49167311136684511, 5.343773310534622567, 5.730690286876297002 ) ) ;
#210247=CARTESIAN_POINT ( 'NONE',  ( -11.41381675112460670, 13.53016735491474343, 3.704697986577268232 ) ) ;
#210252=EDGE_CURVE ( 'NONE', #29424, #151228, #193980, .T. ) ;
#210271=CARTESIAN_POINT ( 'NONE',  ( -11.94105721237523099, 13.40000000000000036, -1.187919463087248939 ) ) ;
#210314=CARTESIAN_POINT ( 'NONE',  ( 10.50000000000000178, 0.000000000000000000, 3.599999999999999201 ) ) ;
#210323=VERTEX_POINT ( 'NONE', #144229 ) ;
#210346=DIRECTION ( 'NONE',  ( -0.000000000000000000, -1.000000000000000000, -0.000000000000000000 ) ) ;
#210350=ORIENTED_EDGE ( 'NONE', *, *, #195398, .T. ) ;
#210351=COLOUR_RGB ( '', 0.31764706, 0.68627451, 0.89019608) ;
#210381=MECHANICAL_DESIGN_GEOMETRIC_PRESENTATION_REPRESENTATION('',(#203406),#141179);
#210390=AXIS2_PLACEMENT_3D ( 'NONE', #78605, #30951, #146842 ) ;
#210391=FILL_AREA_STYLE_COLOUR ( '', #117102 ) ;
#210434=VERTEX_POINT ( 'NONE', #32553 ) ;
#210440=( GEOMETRIC_REPRESENTATION_CONTEXT ( 3 ) GLOBAL_UNCERTAINTY_ASSIGNED_CONTEXT ( ( #32091 ) ) GLOBAL_UNIT_ASSIGNED_CONTEXT ( ( #209041, #214083, #68915 ) ) REPRESENTATION_CONTEXT ( 'NONE', 'WORKASPACE' ) );
#210443=ORIENTED_EDGE ( 'NONE', *, *, #163845, .F. ) ;
#210450=FILL_AREA_STYLE ('',( #78325 ) ) ;
#210462=CARTESIAN_POINT ( 'NONE',  ( 8.521429491328973427, 12.47146749443822422, 8.416430775921163843 ) ) ;
#210479=CARTESIAN_POINT ( 'NONE',  ( -11.41381675112453387, 19.00000000000000000, -3.704697986577182522 ) ) ;
#210493=CARTESIAN_POINT ( 'NONE',  ( -11.86145017354119879, 11.00485634456123840, -1.100000000000000533 ) ) ;
#210514=EDGE_CURVE ( 'NONE', #161745, #9995, #36802, .T. ) ;
#210522=CARTESIAN_POINT ( 'NONE',  ( -1.878313713276878127, 14.99999999999692157, 12.68000002627078082 ) ) ;
#210544=CARTESIAN_POINT ( 'NONE',  ( -15.75000000000000000, 12.69999999999998153, 1.799999999999999600 ) ) ;
#210551=CARTESIAN_POINT ( 'NONE',  ( 11.84668730067608600, 19.00000000000000000, -1.320000000000001616 ) ) ;
#210558=EDGE_CURVE ( 'NONE', #64100, #92493, #58206, .T. ) ;
#210567=CARTESIAN_POINT ( 'NONE',  ( 9.272768930052142977, 15.45663049227336039, -8.558335171112736006 ) ) ;
#210570=CARTESIAN_POINT ( 'NONE',  ( 7.837025389534266751, 13.96141657329141061, 9.967208473298693860 ) ) ;
#210595=CARTESIAN_POINT ( 'NONE',  ( -9.915825940873133959, 4.173851563286998356, 6.175246223022227809 ) ) ;
#210596=DIRECTION ( 'NONE',  ( 0.000000000000000000, -1.000000000000000000, -0.000000000000000000 ) ) ;
#210605=CIRCLE ( 'NONE', #41166, 0.07999999999999933553 ) ;
#210607=CARTESIAN_POINT ( 'NONE',  ( -12.93484866278744150, 7.732355869717920882, 1.092763313629060873 ) ) ;
#210624=CARTESIAN_POINT ( 'NONE',  ( -9.549101787482188186, 15.20623330905540982, 7.267872539799826725 ) ) ;
#210630=ORIENTED_EDGE ( 'NONE', *, *, #208819, .T. ) ;
#210631=CARTESIAN_POINT ( 'NONE',  ( 11.01852871259909961, 9.193369260742729310, 4.626256781840949017 ) ) ;
#210679=CARTESIAN_POINT ( 'NONE',  ( -11.07621050858439915, 5.829138686674238734, -4.513195650290508176 ) ) ;
#210688=CARTESIAN_POINT ( 'NONE',  ( -11.33363864608102567, 7.663751225690653257, -3.950522364644465156 ) ) ;
#210693=VERTEX_POINT ( 'NONE', #200358 ) ;
#210704=CIRCLE ( 'NONE', #214065, 11.92000000000000171 ) ;
#210718=CARTESIAN_POINT ( 'NONE',  ( -12.00288634729131232, 5.507422065878898820, 4.496070577805427959 ) ) ;
#210723=( NAMED_UNIT ( * ) SI_UNIT ( $, .STERADIAN. ) SOLID_ANGLE_UNIT ( ) );
#210726=VERTEX_POINT ( 'NONE', #119192 ) ;
#210753=B_SPLINE_CURVE_WITH_KNOTS ( 'NONE', 3,
 ( #116768, #12791, #196890, #195833, #31210, #146042 ),
 .UNSPECIFIED., .F., .F.,
 ( 4, 2, 4 ),
 ( 0.000000000000000000, 0.0003779448103413553901, 0.0007558896206827107802 ),
 .UNSPECIFIED. ) ;
#210758=B_SPLINE_CURVE_WITH_KNOTS ( 'NONE', 3,
 ( #123478, #67402, #41083, #139657, #51192, #38930, #56250, #17589, #72475, #204598, #33862, #74630, #99941, #55183, #22650, #166005 ),
 .UNSPECIFIED., .F., .F.,
 ( 4, 2, 2, 2, 2, 2, 2, 4 ),
 ( 8.045963024324400998E-05, 0.002777617397444224687, 0.004126196281044714788, 0.005474775164645207491, 0.006823354048245700194, 0.008171932931846193765, 0.009520511815446686468, 0.01086909069904717917 ),
 .UNSPECIFIED. ) ;
#210761=CARTESIAN_POINT ( 'NONE',  ( 9.649767104172532584, 4.268299563709526012, 7.133807922836909121 ) ) ;
#210789=CARTESIAN_POINT ( 'NONE',  ( -11.48243876534946217, 12.29999999999998295, 3.199999999999997957 ) ) ;
#210828=EDGE_CURVE ( 'NONE', #6177, #172406, #34074, .T. ) ;
#210836=CIRCLE ( 'NONE', #128067, 0.07999999999999959921 ) ;
#210883=FILL_AREA_STYLE_COLOUR ( '', #4497 ) ;
#210886=CARTESIAN_POINT ( 'NONE',  ( -10.31538147864342925, 4.824606379122443833, 6.138819041055270098 ) ) ;
#210899=CARTESIAN_POINT ( 'NONE',  ( 1.359357947053562156E-15, 0.000000000000000000, -11.09999999999999964 ) ) ;
#210910=CARTESIAN_POINT ( 'NONE',  ( -15.75000000000000000, 13.79999999999998295, 3.199999999999997957 ) ) ;
#210917=DIRECTION ( 'NONE',  ( 0.000000000000000000, 0.000000000000000000, -1.000000000000000000 ) ) ;
#210920=CARTESIAN_POINT ( 'NONE',  ( 8.996714940757932766, 14.55825685055163987, -7.941925727616619746 ) ) ;
#210945=FACE_OUTER_BOUND ( 'NONE', #195885, .T. ) ;
#210958=CARTESIAN_POINT ( 'NONE',  ( 10.40189579028154832, 9.152068647944213708, -6.036026366622869510 ) ) ;
#210964=ORIENTED_EDGE ( 'NONE', *, *, #6048, .F. ) ;
#210966=CARTESIAN_POINT ( 'NONE',  ( 11.96407947313512743, 8.207545470847758651, -0.7892166907401461096 ) ) ;
#210980=CARTESIAN_POINT ( 'NONE',  ( -11.07790593930098311, 13.79999999999999893, 0.6999999999999992895 ) ) ;
#210982=CARTESIAN_POINT ( 'NONE',  ( -11.04986239659823433, 13.60939231485699352, -1.056426191432995765 ) ) ;
#210993=SURFACE_SIDE_STYLE ('',( #178525 ) ) ;
#210999=CARTESIAN_POINT ( 'NONE',  ( -9.645406396194509568, 4.042443384815813445, -6.587269312116742270 ) ) ;
#211004=VERTEX_POINT ( 'NONE', #55202 ) ;
#211051=VERTEX_POINT ( 'NONE', #154837 ) ;
#211067=EDGE_CURVE ( 'NONE', #175025, #204806, #130643, .T. ) ;
#211084=LINE ( 'NONE', #207892, #718 ) ;
#211089=DIRECTION ( 'NONE',  ( 1.000000000000000000, -0.000000000000000000, -0.000000000000000000 ) ) ;
#211111=SURFACE_STYLE_FILL_AREA ( #12909 ) ;
#211121=CARTESIAN_POINT ( 'NONE',  ( -10.41980074470002648, 5.020554563858687480, 5.279403930596816785 ) ) ;
#211122=VERTEX_POINT ( 'NONE', #206765 ) ;
#211139=CARTESIAN_POINT ( 'NONE',  ( 1.734723475976807094E-15, 14.55305236562695193, 11.95586206896570580 ) ) ;
#211169=CARTESIAN_POINT ( 'NONE',  ( 0.1453961305826048100, 14.48154449402677812, 11.99911913288686627 ) ) ;
#211178=CARTESIAN_POINT ( 'NONE',  ( -10.95308175811721085, 11.29999999999999893, -1.800000000000001155 ) ) ;
#211218=EDGE_CURVE ( 'NONE', #106229, #90065, #85874, .T. ) ;
#211240=CARTESIAN_POINT ( 'NONE',  ( -11.78331023100045627, 9.799999999999982947, 1.799999999999999600 ) ) ;
#211247=ORIENTED_EDGE ( 'NONE', *, *, #191199, .T. ) ;
#211251=CIRCLE ( 'NONE', #97185, 0.5000000000000013323 ) ;
#211285=DIRECTION ( 'NONE',  ( 0.000000000000000000, 0.000000000000000000, -1.000000000000000000 ) ) ;
#211291=FACE_OUTER_BOUND ( 'NONE', #74415, .T. ) ;
#211308=CARTESIAN_POINT ( 'NONE',  ( 8.576050019794697832, 13.83380793569078016, 8.329213815152254341 ) ) ;
#211338=CARTESIAN_POINT ( 'NONE',  ( -11.49966000274993583, 12.35767154435234083, 3.429881629452983915 ) ) ;
#211379=DIRECTION ( 'NONE',  ( 0.000000000000000000, -1.000000000000000000, 0.000000000000000000 ) ) ;
#211394=ORIENTED_EDGE ( 'NONE', *, *, #79201, .T. ) ;
#211399=AXIS2_PLACEMENT_3D ( 'NONE', #74762, #139785, #6532 ) ;
#211463=DIRECTION ( 'NONE',  ( 0.000000000000000000, -0.000000000000000000, 1.000000000000000000 ) ) ;
#211468=ORIENTED_EDGE ( 'NONE', *, *, #113810, .T. ) ;
#211493=VECTOR ( 'NONE', #156563, 1000.000000000000000 ) ;
#211494=CARTESIAN_POINT ( 'NONE',  ( 0.000000000000000000, 15.44694763437329676, 0.000000000000000000 ) ) ;
#211497=CARTESIAN_POINT ( 'NONE',  ( 11.94654170777226021, 9.948256738410641731, -1.134972293687621647 ) ) ;
#211523=EDGE_CURVE ( 'NONE', #139784, #79300, #189619, .T. ) ;
#211525=CARTESIAN_POINT ( 'NONE',  ( 8.381989347167957405, 12.99464372445137883, 8.515743443721982331 ) ) ;
#211526=ORIENTED_EDGE ( 'NONE', *, *, #153496, .F. ) ;
#211563=B_SPLINE_CURVE_WITH_KNOTS ( 'NONE', 3,
 ( #61687, #127857, #162402, #29194, #178650, #146166, #191664 ),
 .UNSPECIFIED., .F., .F.,
 ( 4, 3, 4 ),
 ( 0.000000000000000000, 3.302265273836957072E-05, 4.223967315999526832E-05 ),
 .UNSPECIFIED. ) ;
#211594=ORIENTED_EDGE ( 'NONE', *, *, #30633, .T. ) ;
#211602=VECTOR ( 'NONE', #106779, 1000.000000000000000 ) ;
#211607=DIRECTION ( 'NONE',  ( -0.9982742078614211811, 0.000000000000000000, 0.05872483221476467591 ) ) ;
#211619=DIRECTION ( 'NONE',  ( -0.000000000000000000, 1.000000000000000000, 1.804652791718263484E-16 ) ) ;
#211624=CARTESIAN_POINT ( 'NONE',  ( 9.664668247050562044, 13.51658191024029243, -8.185676666504042132 ) ) ;
#211627=CARTESIAN_POINT ( 'NONE',  ( 8.597997168627587783, 14.01909641423478092, 7.911570108784474087 ) ) ;
#211641=AXIS2_PLACEMENT_3D ( 'NONE', #74978, #156242, #155165 ) ;
#211658=CARTESIAN_POINT ( 'NONE',  ( -10.94023239993386554, 4.766145680744502400, 4.420001064107922595 ) ) ;
#211686=CARTESIAN_POINT ( 'NONE',  ( 12.00020817714739785, 7.639625205866504842, -0.2088832295647653214 ) ) ;
#211737=CARTESIAN_POINT ( 'NONE',  ( -11.68215918550372123, 7.481139959555187069, 2.549995685925019462 ) ) ;
#211746=CARTESIAN_POINT ( 'NONE',  ( -11.77162061555259243, 8.648954000449407431, -2.104286885599118140 ) ) ;
#211752=VERTEX_POINT ( 'NONE', #163369 ) ;
#211770=EDGE_CURVE ( 'NONE', #193425, #173258, #54803, .T. ) ;
#211776=CARTESIAN_POINT ( 'NONE',  ( -11.79406710134376191, 4.782197168659454434, 4.941180684906744780 ) ) ;
#211796=SURFACE_SIDE_STYLE ('',( #131677 ) ) ;
#211836=FACE_OUTER_BOUND ( 'NONE', #97270, .T. ) ;
#211846=CARTESIAN_POINT ( 'NONE',  ( -9.979907920417568690, 3.147823346236176878, -6.101210848797135711 ) ) ;
#211851=MECHANICAL_DESIGN_GEOMETRIC_PRESENTATION_REPRESENTATION('',(#80294),#197927);
#211856=CARTESIAN_POINT ( 'NONE',  ( -11.84101807917483740, 12.48978499739122405, -1.444039656437080099 ) ) ;
#211869=EDGE_LOOP ( 'NONE', ( #43076, #173564, #67789, #85405 ) ) ;
#211871=B_SPLINE_CURVE_WITH_KNOTS ( 'NONE', 3,
 ( #195311, #162820, #46942, #180125, #84746, #89037 ),
 .UNSPECIFIED., .F., .F.,
 ( 4, 2, 4 ),
 ( 0.001889712630306643456, 0.002203932548491402497, 0.002518152466676161320 ),
 .UNSPECIFIED. ) ;
#211888=UNCERTAINTY_MEASURE_WITH_UNIT (LENGTH_MEASURE( 1.000000000000000082E-05 ), #161440, 'distance_accuracy_value', 'NONE');
#211945=CARTESIAN_POINT ( 'NONE',  ( 11.91939557091538582, 6.691048939571908605, 0.9932293525215405428 ) ) ;
#211949=CARTESIAN_POINT ( 'NONE',  ( -10.42580506876874047, 5.089579995674308854, 5.943607252937018082 ) ) ;
#211969=CARTESIAN_POINT ( 'NONE',  ( 11.04536101718726293, 13.40000000000000036, -1.100000000000002087 ) ) ;
#211979=( BOUNDED_SURFACE ( )  B_SPLINE_SURFACE ( 3, 2, ( 
 ( #96547, #147409, #213435 ),
 ( #64016, #114955, #129110 ),
 ( #60814, #79197, #44588 ),
 ( #110702, #46722, #131214 ),
 ( #197202, #32578, #30462 ),
 ( #47796, #95486, #15243 ),
 ( #48841, #130164, #180956 ),
 ( #61886, #178851, #162594 ) ),
 .UNSPECIFIED., .F., .F., .T. ) 
 B_SPLINE_SURFACE_WITH_KNOTS ( ( 4, 2, 2, 4 ),
 ( 3, 3 ),
 ( 2.385244779468109755E-18, 0.0004821367237705008143, 0.0009642734475409992434, 0.001928546895081996101 ),
 ( 0.000000000000000000, 1.000000000000000000 ),
 .UNSPECIFIED. ) 
 GEOMETRIC_REPRESENTATION_ITEM ( )  RATIONAL_B_SPLINE_SURFACE ( (
 ( 1.000000000000000000, 0.8509629433086528527, 1.000000000000000000),
 ( 1.000000000000000000, 0.8509293920024736391, 1.000000000000000000),
 ( 1.000000000000000000, 0.8507640800581817153, 1.000000000000000000),
 ( 1.000000000000000000, 0.8504069559990277138, 1.000000000000000000),
 ( 1.000000000000000000, 0.8502555126865255497, 1.000000000000000000),
 ( 1.000000000000000000, 0.8490919837716710550, 1.000000000000000000),
 ( 1.000000000000000000, 0.8474110456169804406, 1.000000000000000000),
 ( 1.000000000000000000, 0.8462382765735556589, 1.000000000000000000) ) ) 
 REPRESENTATION_ITEM ( '' )  SURFACE ( )  );
#211982=CARTESIAN_POINT ( 'NONE',  ( 8.610948272048309704, 14.96724361927355496, -8.359267069145829510 ) ) ;
#211995=STYLED_ITEM ( 'NONE', ( #123004 ), #66139 ) ;
#212006=CARTESIAN_POINT ( 'NONE',  ( -11.01135777277262129, 10.89999999999998259, 1.399999999999998579 ) ) ;
#212019=CARTESIAN_POINT ( 'NONE',  ( 8.206244894449710614, 14.14858862657662009, -8.756074973582041565 ) ) ;
#212029=CARTESIAN_POINT ( 'NONE',  ( 12.54948750854022954, 7.400697955233512815, 0.9574523190714994136 ) ) ;
#212031=CARTESIAN_POINT ( 'NONE',  ( -10.30047605039691128, 4.688744718740807116, 5.507884344589919934 ) ) ;
#212039=ORIENTED_EDGE ( 'NONE', *, *, #213502, .T. ) ;
#212044=CARTESIAN_POINT ( 'NONE',  ( 0.08011315928756995719, 14.48196125337680229, 11.99973258290717659 ) ) ;
#212057=( NAMED_UNIT ( * ) PLANE_ANGLE_UNIT ( ) SI_UNIT ( $, .RADIAN. ) );
#212072=CYLINDRICAL_SURFACE ( 'NONE', #60605, 0.3999999999999997446 ) ;
#212105=ORIENTED_EDGE ( 'NONE', *, *, #14127, .F. ) ;
#212128=B_SPLINE_CURVE_WITH_KNOTS ( 'NONE', 3,
 ( #88614, #153606, #121185, #189293, #36634, #188217 ),
 .UNSPECIFIED., .F., .F.,
 ( 4, 2, 4 ),
 ( 0.000000000000000000, 0.0003155923098472858596, 0.0006311846196945720446 ),
 .UNSPECIFIED. ) ;
#212134=DIRECTION ( 'NONE',  ( -0.05872483221476459958, 0.000000000000000000, 0.9982742078614211811 ) ) ;
#212136=AXIS2_PLACEMENT_3D ( 'NONE', #128641, #162128, #93945 ) ;
#212142=ORIENTED_EDGE ( 'NONE', *, *, #206552, .F. ) ;
#212147=CARTESIAN_POINT ( 'NONE',  ( 8.790438134619869004, 13.29428800202395955, -8.101059483297389008 ) ) ;
#212151=LINE ( 'NONE', #162372, #85745 ) ;
#212154=CARTESIAN_POINT ( 'NONE',  ( -1.499999999999961364, 7.000000000000000000, 10.64483442802188762 ) ) ;
#212174=CARTESIAN_POINT ( 'NONE',  ( -15.75000000000000000, 13.39999999999998259, 3.199999999999997957 ) ) ;
#212181=CARTESIAN_POINT ( 'NONE',  ( 11.94105721237523277, 12.57259609010266921, -1.187919463087249827 ) ) ;
#212198=DIRECTION ( 'NONE',  ( 0.000000000000000000, 0.000000000000000000, 1.000000000000000000 ) ) ;
#212203=ADVANCED_FACE ( 'NONE', ( #35480 ), #115728, .T. ) ;
#212215=LINE ( 'NONE', #101682, #29588 ) ;
#212223=B_SPLINE_CURVE_WITH_KNOTS ( 'NONE', 3,
 ( #22573, #55101, #186145, #169903, #23649, #70248 ),
 .UNSPECIFIED., .F., .F.,
 ( 4, 2, 4 ),
 ( 0.000000000000000000, 0.0003172254002810707399, 0.0006344508005621414797 ),
 .UNSPECIFIED. ) ;
#212232=AXIS2_PLACEMENT_3D ( 'NONE', #13313, #180094, #81522 ) ;
#212265=CARTESIAN_POINT ( 'NONE',  ( 11.44779963594988637, 12.70000000000000107, -3.600000000000000977 ) ) ;
#212266=DIRECTION ( 'NONE',  ( -0.000000000000000000, -1.000000000000000000, -0.000000000000000000 ) ) ;
#212293=EDGE_CURVE ( 'NONE', #9995, #187611, #124003, .T. ) ;
#212303=ORIENTED_EDGE ( 'NONE', *, *, #11240, .F. ) ;
#212311=DIRECTION ( 'NONE',  ( 1.000000000000000000, -0.000000000000000000, -0.000000000000000000 ) ) ;
#212317=CARTESIAN_POINT ( 'NONE',  ( 11.41381675112453387, 10.89999999999998259, 3.704697986577180746 ) ) ;
#212328=DIRECTION ( 'NONE',  ( 1.000000000000000000, 0.000000000000000000, -0.000000000000000000 ) ) ;
#212336=EDGE_LOOP ( 'NONE', ( #11194, #93857, #212754, #132188 ) ) ;
#212366=FACE_OUTER_BOUND ( 'NONE', #30607, .T. ) ;
#212368=AXIS2_PLACEMENT_3D ( 'NONE', #196571, #112193, #80693 ) ;
#212369=ORIENTED_EDGE ( 'NONE', *, *, #2823, .F. ) ;
#212381=CARTESIAN_POINT ( 'NONE',  ( 11.92619526913699879, 19.00000000000000000, 1.328859060402684644 ) ) ;
#212408=PRESENTATION_STYLE_ASSIGNMENT (( #131246 ) ) ;
#212414=EDGE_CURVE ( 'NONE', #11502, #145411, #203505, .T. ) ;
#212435=CARTESIAN_POINT ( 'NONE',  ( 11.86145016429273191, 12.69999999999999929, 1.099999999999996758 ) ) ;
#212473=VERTEX_POINT ( 'NONE', #138342 ) ;
#212479=B_SPLINE_CURVE_WITH_KNOTS ( 'NONE', 3,
 ( #133868, #88282, #35242, #104538, #204119, #203063 ),
 .UNSPECIFIED., .F., .F.,
 ( 4, 2, 4 ),
 ( 0.001259240562161248120, 0.001573673787268790349, 0.001888107012376332794 ),
 .UNSPECIFIED. ) ;
#212491=EDGE_CURVE ( 'NONE', #166496, #25291, #76346, .T. ) ;
#212502=CARTESIAN_POINT ( 'NONE',  ( -11.94105721237523454, 11.02740784401788865, 1.187919463087248273 ) ) ;
#212505=CARTESIAN_POINT ( 'NONE',  ( -9.540655113774946017, 3.481540744127369802, 7.145788969735951568 ) ) ;
#212532=FILL_AREA_STYLE ('',( #197353 ) ) ;
#212534=CARTESIAN_POINT ( 'NONE',  ( 11.89204169242350950, 11.29999999999999893, -0.8046421800350563869 ) ) ;
#212536=CARTESIAN_POINT ( 'NONE',  ( -4.933501523973760072E-10, 15.51845925587262798, -12.00000000000000178 ) ) ;
#212548=CARTESIAN_POINT ( 'NONE',  ( 0.04160626335162659339, 14.52071188304540073, 11.99061301703373417 ) ) ;
#212553=ADVANCED_FACE ( 'NONE', ( #139413 ), #189210, .F. ) ;
#212590=VECTOR ( 'NONE', #57002, 1000.000000000000000 ) ;
#212595=CARTESIAN_POINT ( 'NONE',  ( 9.228631970132603612, 13.18394157654138965, -9.019657609914000673 ) ) ;
#212600=ORIENTED_EDGE ( 'NONE', *, *, #195600, .T. ) ;
#212675=MECHANICAL_DESIGN_GEOMETRIC_PRESENTATION_REPRESENTATION('',(#81279),#191955);
#212687=PRESENTATION_STYLE_ASSIGNMENT (( #159690 ) ) ;
#212691=CARTESIAN_POINT ( 'NONE',  ( 9.503631714379071838, 15.23661009679124057, -8.229227087069268975 ) ) ;
#212694=CARTESIAN_POINT ( 'NONE',  ( 8.250525573328690854, 13.32549038962357635, 8.564080365641034476 ) ) ;
#212695=CIRCLE ( 'NONE', #101526, 11.92000000000000171 ) ;
#212701=ORIENTED_EDGE ( 'NONE', *, *, #71135, .T. ) ;
#212713=EDGE_CURVE ( 'NONE', #108406, #152119, #182180, .T. ) ;
#212718=TOROIDAL_SURFACE ( 'NONE', #164335, -0.1799999999926198968, 0.5000000000000013323 ) ;
#212726=CARTESIAN_POINT ( 'NONE',  ( -10.91672646594461327, 4.673612064222224305, 4.467269497407427181 ) ) ;
#212742=CARTESIAN_POINT ( 'NONE',  ( 11.33772463945037146, 12.69999999999998153, 3.599999999999999201 ) ) ;
#212743=EDGE_CURVE ( 'NONE', #46648, #137788, #110369, .T. ) ;
#212748=CARTESIAN_POINT ( 'NONE',  ( -9.393959922490113357, 14.54118366885366775, 7.466876303508932722 ) ) ;
#212754=ORIENTED_EDGE ( 'NONE', *, *, #1482, .F. ) ;
#212756=CARTESIAN_POINT ( 'NONE',  ( 11.52671564374114155, 8.445739998960311468, -3.359000350707669558 ) ) ;
#212765=DIRECTION ( 'NONE',  ( 0.2150645590070887347, -0.8781765503997437383, 0.4272624273056235267 ) ) ;
#212791=CARTESIAN_POINT ( 'NONE',  ( -1.790573066372362465, 14.55177515835072199, -11.85444247180616095 ) ) ;
#212803=CARTESIAN_POINT ( 'NONE',  ( -12.00016495910608860, 8.079444814310500433, -0.2607765302759474380 ) ) ;
#212812=CARTESIAN_POINT ( 'NONE',  ( -11.94312002716720045, 8.978941879399096493, 0.6089553112034360449 ) ) ;
#212815=CARTESIAN_POINT ( 'NONE',  ( -15.75000000000000000, 13.79999999999999893, -1.800000000000001155 ) ) ;
#212825=ORIENTED_EDGE ( 'NONE', *, *, #189834, .T. ) ;
#212833=STYLED_ITEM ( 'NONE', ( #162275 ), #190216 ) ;
#212845=ORIENTED_EDGE ( 'NONE', *, *, #60871, .T. ) ;
#212861=CARTESIAN_POINT ( 'NONE',  ( -11.89317557362571698, 12.33724156162407226, 1.599935658896036283 ) ) ;
#212872=( NAMED_UNIT ( * ) PLANE_ANGLE_UNIT ( ) SI_UNIT ( $, .RADIAN. ) );
#212890=AXIS2_PLACEMENT_3D ( 'NONE', #11508, #83706, #98914 ) ;
#212918=ORIENTED_EDGE ( 'NONE', *, *, #205156, .F. ) ;
#212957=DIRECTION ( 'NONE',  ( -0.000000000000000000, -1.000000000000000000, -0.000000000000000000 ) ) ;
#212975=CARTESIAN_POINT ( 'NONE',  ( 11.00595142344305444, 9.990095813384931134, -1.443824005414910072 ) ) ;
#212992=ORIENTED_EDGE ( 'NONE', *, *, #212743, .F. ) ;
#213018=CIRCLE ( 'NONE', #161099, 0.08000000000000040412 ) ;
#213027=CARTESIAN_POINT ( 'NONE',  ( -0.0001326642102265163461, 15.43055640418811514, 11.92506554388277706 ) ) ;
#213049=CARTESIAN_POINT ( 'NONE',  ( 8.400184771233881520, 15.16344228256336812, -8.571051625424484399 ) ) ;
#213085=AXIS2_PLACEMENT_3D ( 'NONE', #101199, #205090, #173711 ) ;
#213097=CARTESIAN_POINT ( 'NONE',  ( 10.16976112282614508, 11.75387517088144484, 7.514388995082887490 ) ) ;
#213110=EDGE_CURVE ( 'NONE', #124865, #188409, #70888, .T. ) ;
#213113=CARTESIAN_POINT ( 'NONE',  ( -11.04536101718726293, 13.50462094045401962, 1.099999999999999201 ) ) ;
#213126=CARTESIAN_POINT ( 'NONE',  ( 9.574107819074903603, 3.767510227260138844, -7.159700062698973078 ) ) ;
#213132=ADVANCED_FACE ( 'NONE', ( #10446 ), #142630, .F. ) ;
#213143=PRESENTATION_STYLE_ASSIGNMENT (( #131953 ) ) ;
#213156=CIRCLE ( 'NONE', #150892, 12.00000000000000178 ) ;
#213253=PRESENTATION_STYLE_ASSIGNMENT (( #147227 ) ) ;
#213258=UNCERTAINTY_MEASURE_WITH_UNIT (LENGTH_MEASURE( 1.000000000000000082E-05 ), #16782, 'distance_accuracy_value', 'NONE');
#213276=CARTESIAN_POINT ( 'NONE',  ( 11.04536101718726293, 0.000000000000000000, -1.100000000000002087 ) ) ;
#213280=( GEOMETRIC_REPRESENTATION_CONTEXT ( 3 ) GLOBAL_UNCERTAINTY_ASSIGNED_CONTEXT ( ( #68019 ) ) GLOBAL_UNIT_ASSIGNED_CONTEXT ( ( #72500, #138600, #50942 ) ) REPRESENTATION_CONTEXT ( 'NONE', 'WORKASPACE' ) );
#213301=DIRECTION ( 'NONE',  ( -0.000000000000000000, 1.000000000000000000, -0.000000000000000000 ) ) ;
#213307=CARTESIAN_POINT ( 'NONE',  ( 7.873621124554150974, 14.32272913405169668, 9.058612350049280337 ) ) ;
#213325=ORIENTED_EDGE ( 'NONE', *, *, #74394, .T. ) ;
#213328=FACE_OUTER_BOUND ( 'NONE', #134844, .T. ) ;
#213339=AXIS2_PLACEMENT_3D ( 'NONE', #11279, #93635, #14472 ) ;
#213345=CARTESIAN_POINT ( 'NONE',  ( 11.81907076198602802, 9.842687754035216230, -1.592066415281268243 ) ) ;
#213397=ORIENTED_EDGE ( 'NONE', *, *, #92241, .T. ) ;
#213413=CARTESIAN_POINT ( 'NONE',  ( 1.469576158976824144E-15, 19.00000000000000000, 12.00000000000000178 ) ) ;
#213435=CARTESIAN_POINT ( 'NONE',  ( -9.604686356149271020, 4.518467169708413778, -7.193747284969076006 ) ) ;
#213452=CARTESIAN_POINT ( 'NONE',  ( 11.87828357749949681, 11.30310252740378729, -1.708055325888855114 ) ) ;
#213467=( NAMED_UNIT ( * ) PLANE_ANGLE_UNIT ( ) SI_UNIT ( $, .RADIAN. ) );
#213500=ORIENTED_EDGE ( 'NONE', *, *, #110293, .F. ) ;
#213502=EDGE_CURVE ( 'NONE', #8666, #105457, #44613, .T. ) ;
#213503=UNCERTAINTY_MEASURE_WITH_UNIT (LENGTH_MEASURE( 1.000000000000000082E-05 ), #89871, 'distance_accuracy_value', 'NONE');
#213513=VERTEX_POINT ( 'NONE', #23219 ) ;
#213549=ORIENTED_EDGE ( 'NONE', *, *, #98948, .F. ) ;
#213554=AXIS2_PLACEMENT_3D ( 'NONE', #23812, #89916, #193779 ) ;
#213555=DIRECTION ( 'NONE',  ( 1.224646799147343346E-16, 0.000000000000000000, -1.000000000000000000 ) ) ;
#213557=CARTESIAN_POINT ( 'NONE',  ( 11.52901446936750141, 11.29425527467587465, -3.330874149801114292 ) ) ;
#213595=CARTESIAN_POINT ( 'NONE',  ( 0.02465203476893947088, 14.53755993404379510, 11.97749487451461903 ) ) ;
#213621=CARTESIAN_POINT ( 'NONE',  ( -11.86239285000045918, 9.799999999999997158, -1.812080536912752837 ) ) ;
#213623=EDGE_LOOP ( 'NONE', ( #180610, #156940, #196868, #189125 ) ) ;
#213624=CIRCLE ( 'NONE', #106405, 12.00000000000000178 ) ;
#213630=PRESENTATION_STYLE_ASSIGNMENT (( #194210 ) ) ;
#213642=CARTESIAN_POINT ( 'NONE',  ( 9.318301066091441598, 12.86598888409864472, -8.945124285776126172 ) ) ;
#213657=( BOUNDED_SURFACE ( )  B_SPLINE_SURFACE ( 3, 2, ( 
 ( #204762, #138744, #56414 ),
 ( #40167, #106281, #172302 ),
 ( #23891, #89997, #73722 ),
 ( #205848, #175506, #57481 ),
 ( #41249, #107357, #173379 ),
 ( #24963, #91065, #74799 ),
 ( #124696, #153919, #108431 ),
 ( #174451, #26027, #92137 ),
 ( #141963, #207975, #59602 ),
 ( #125760, #5489, #137678 ),
 ( #10835, #46572, #80113 ),
 ( #61742, #160308, #95339 ),
 ( #110561, #146218, #44443 ),
 ( #211169, #45510, #159234 ) ),
 .UNSPECIFIED., .F., .F., .T. ) 
 B_SPLINE_SURFACE_WITH_KNOTS ( ( 4, 2, 2, 2, 2, 2, 4 ),
 ( 3, 3 ),
 ( 0.01742726680619078455, 0.02012515843099235008, 0.02147410424339313284, 0.02282305005579391213, 0.02417199586819469143, 0.02552094168059547419, 0.02821883330539703971 ),
 ( 0.000000000000000000, 1.000000000000000000 ),
 .UNSPECIFIED. ) 
 GEOMETRIC_REPRESENTATION_ITEM ( )  RATIONAL_B_SPLINE_SURFACE ( (
 ( 1.000000000000000000, 0.8509629433930230302, 1.000000000000000000),
 ( 1.000000000000000000, 0.8507187689822764964, 1.000000000000000000),
 ( 1.000000000000000000, 0.8494327192471640142, 1.000000000000000000),
 ( 1.000000000000000000, 0.8495462935814993566, 1.000000000000000000),
 ( 1.000000000000000000, 0.8498623255111610320, 1.000000000000000000),
 ( 1.000000000000000000, 0.8506092561374887229, 1.000000000000000000),
 ( 1.000000000000000000, 0.8510280321988274999, 1.000000000000000000),
 ( 1.000000000000000000, 0.8508805742456044818, 1.000000000000000000),
 ( 1.000000000000000000, 0.8503832817317976689, 1.000000000000000000),
 ( 1.000000000000000000, 0.8496212719666990099, 1.000000000000000000),
 ( 1.000000000000000000, 0.8493586043581990985, 1.000000000000000000),
 ( 1.000000000000000000, 0.8494730729331905206, 1.000000000000000000),
 ( 1.000000000000000000, 0.8509586478585877689, 1.000000000000000000),
 ( 1.000000000000000000, 0.8509656014577856586, 1.000000000000000000) ) ) 
 REPRESENTATION_ITEM ( '' )  SURFACE ( )  );
#213665=EDGE_CURVE ( 'NONE', #79400, #133821, #61914, .T. ) ;
#213676=CARTESIAN_POINT ( 'NONE',  ( -11.84668730067608600, 13.40000000000000036, -1.400000000000001910 ) ) ;
#213686=EDGE_CURVE ( 'NONE', #28237, #154122, #98660, .T. ) ;
#213693=CARTESIAN_POINT ( 'NONE',  ( -11.26761089376506497, 6.406307030788339851, 3.999051048939115560 ) ) ;
#213697=CARTESIAN_POINT ( 'NONE',  ( -11.82646905334693699, 7.635427781191967078, -2.047549239027206092 ) ) ;
#213736=CARTESIAN_POINT ( 'NONE',  ( 9.333039360705550180, 4.446953957879813402, -7.472411811099956225 ) ) ;
#213740=CARTESIAN_POINT ( 'NONE',  ( 7.320801413324473650, 16.00000000000000000, -10.35317664616355771 ) ) ;
#213763=AXIS2_PLACEMENT_3D ( 'NONE', #24638, #58224, #109183 ) ;
#213774=CARTESIAN_POINT ( 'NONE',  ( -10.92050379694822837, 4.688480456342538183, -4.459762147120462039 ) ) ;
#213792=CARTESIAN_POINT ( 'NONE',  ( -9.421011374644489678, 14.56515202819860377, 7.432750069618532685 ) ) ;
#213800=CARTESIAN_POINT ( 'NONE',  ( 9.423393029473404070, 13.09419267589542457, -7.355985009210963987 ) ) ;
#213806=AXIS2_PLACEMENT_3D ( 'NONE', #59343, #76653, #175249 ) ;
#213810=STYLED_ITEM ( 'NONE', ( #8916 ), #9062 ) ;
#213813=CARTESIAN_POINT ( 'NONE',  ( -10.83760191302001097, 4.885617943545219610, -4.963142630924989973 ) ) ;
#213833=DIRECTION ( 'NONE',  ( 1.000000000000000000, -0.000000000000000000, -0.000000000000000000 ) ) ;
#213852=CARTESIAN_POINT ( 'NONE',  ( -11.51728355775449231, 7.078142246183236175, 3.212931496948879140 ) ) ;
#213861=CARTESIAN_POINT ( 'NONE',  ( -11.15508160014129224, 7.312941860064643862, -4.429679592206957395 ) ) ;
#213882=LINE ( 'NONE', #178235, #46566 ) ;
#213893=SURFACE_STYLE_USAGE ( .BOTH. , #11453 ) ;
#213908=CARTESIAN_POINT ( 'NONE',  ( -11.00593736619310725, 12.48999492864588134, 1.443925800506593804 ) ) ;
#213911=DIRECTION ( 'NONE',  ( 0.000000000000000000, 0.000000000000000000, -1.000000000000000000 ) ) ;
#213927=CARTESIAN_POINT ( 'NONE',  ( 9.445304453185871196, 4.469082159062184978, 7.402818517570845636 ) ) ;
#213959=VERTEX_POINT ( 'NONE', #165787 ) ;
#213960=CIRCLE ( 'NONE', #131048, 11.95586206894162906 ) ;
#213963=SURFACE_SIDE_STYLE ('',( #45135 ) ) ;
#213975=CARTESIAN_POINT ( 'NONE',  ( -11.91826849282518452, 13.39999999999998437, 1.399999999999998579 ) ) ;
#213995=UNCERTAINTY_MEASURE_WITH_UNIT (LENGTH_MEASURE( 1.000000000000000082E-05 ), #101529, 'distance_accuracy_value', 'NONE');
#214002=CARTESIAN_POINT ( 'NONE',  ( 0.000000000000000000, 18.91999999999999815, 0.000000000000000000 ) ) ;
#214020=CARTESIAN_POINT ( 'NONE',  ( 11.52463353791759992, 9.719999999999998863, -3.346594096177641475 ) ) ;
#214030=CARTESIAN_POINT ( 'NONE',  ( -10.87339879486171590, 5.131770238416462959, 5.487091846871368084 ) ) ;
#214031=ORIENTED_EDGE ( 'NONE', *, *, #154855, .T. ) ;
#214044=ORIENTED_EDGE ( 'NONE', *, *, #196360, .T. ) ;
#214049=ADVANCED_FACE ( 'NONE', ( #45659 ), #172781, .F. ) ;
#214065=AXIS2_PLACEMENT_3D ( 'NONE', #74276, #138215, #22278 ) ;
#214076=PLANE ( 'NONE',  #79007 ) ;
#214083=( NAMED_UNIT ( * ) PLANE_ANGLE_UNIT ( ) SI_UNIT ( $, .RADIAN. ) );
#214094=AXIS2_PLACEMENT_3D ( 'NONE', #34274, #18005, #101412 ) ;
#214112=CARTESIAN_POINT ( 'NONE',  ( -9.645452764996941042, 5.068254855380425639, -6.574395040668256307 ) ) ;
#214113=CARTESIAN_POINT ( 'NONE',  ( -11.55950211276791428, 11.37999999999998302, 3.221476510067114329 ) ) ;
#214126=CARTESIAN_POINT ( 'NONE',  ( 8.900805598352070191, 12.81158145916116453, -8.049589252430559227 ) ) ;
#214135=FACE_OUTER_BOUND ( 'NONE', #163325, .T. ) ;
#214136=CARTESIAN_POINT ( 'NONE',  ( 8.892182451728965376, 12.91678122746358248, -7.588089516412551028 ) ) ;
#214147=CARTESIAN_POINT ( 'NONE',  ( 8.742474708574045295, 13.54844359601399972, -8.153352885485730894 ) ) ;
#214187=CIRCLE ( 'NONE', #120944, 12.00000000000000178 ) ;
#214287=CARTESIAN_POINT ( 'NONE',  ( 11.00595142344305444, 12.49009581338493113, -1.443824005414910072 ) ) ;
#214308=EDGE_CURVE ( 'NONE', #31644, #203495, #68213, .T. ) ;
#214333=( NAMED_UNIT ( * ) SI_UNIT ( $, .STERADIAN. ) SOLID_ANGLE_UNIT ( ) );
ENDSEC;
END-ISO-10303-21;
